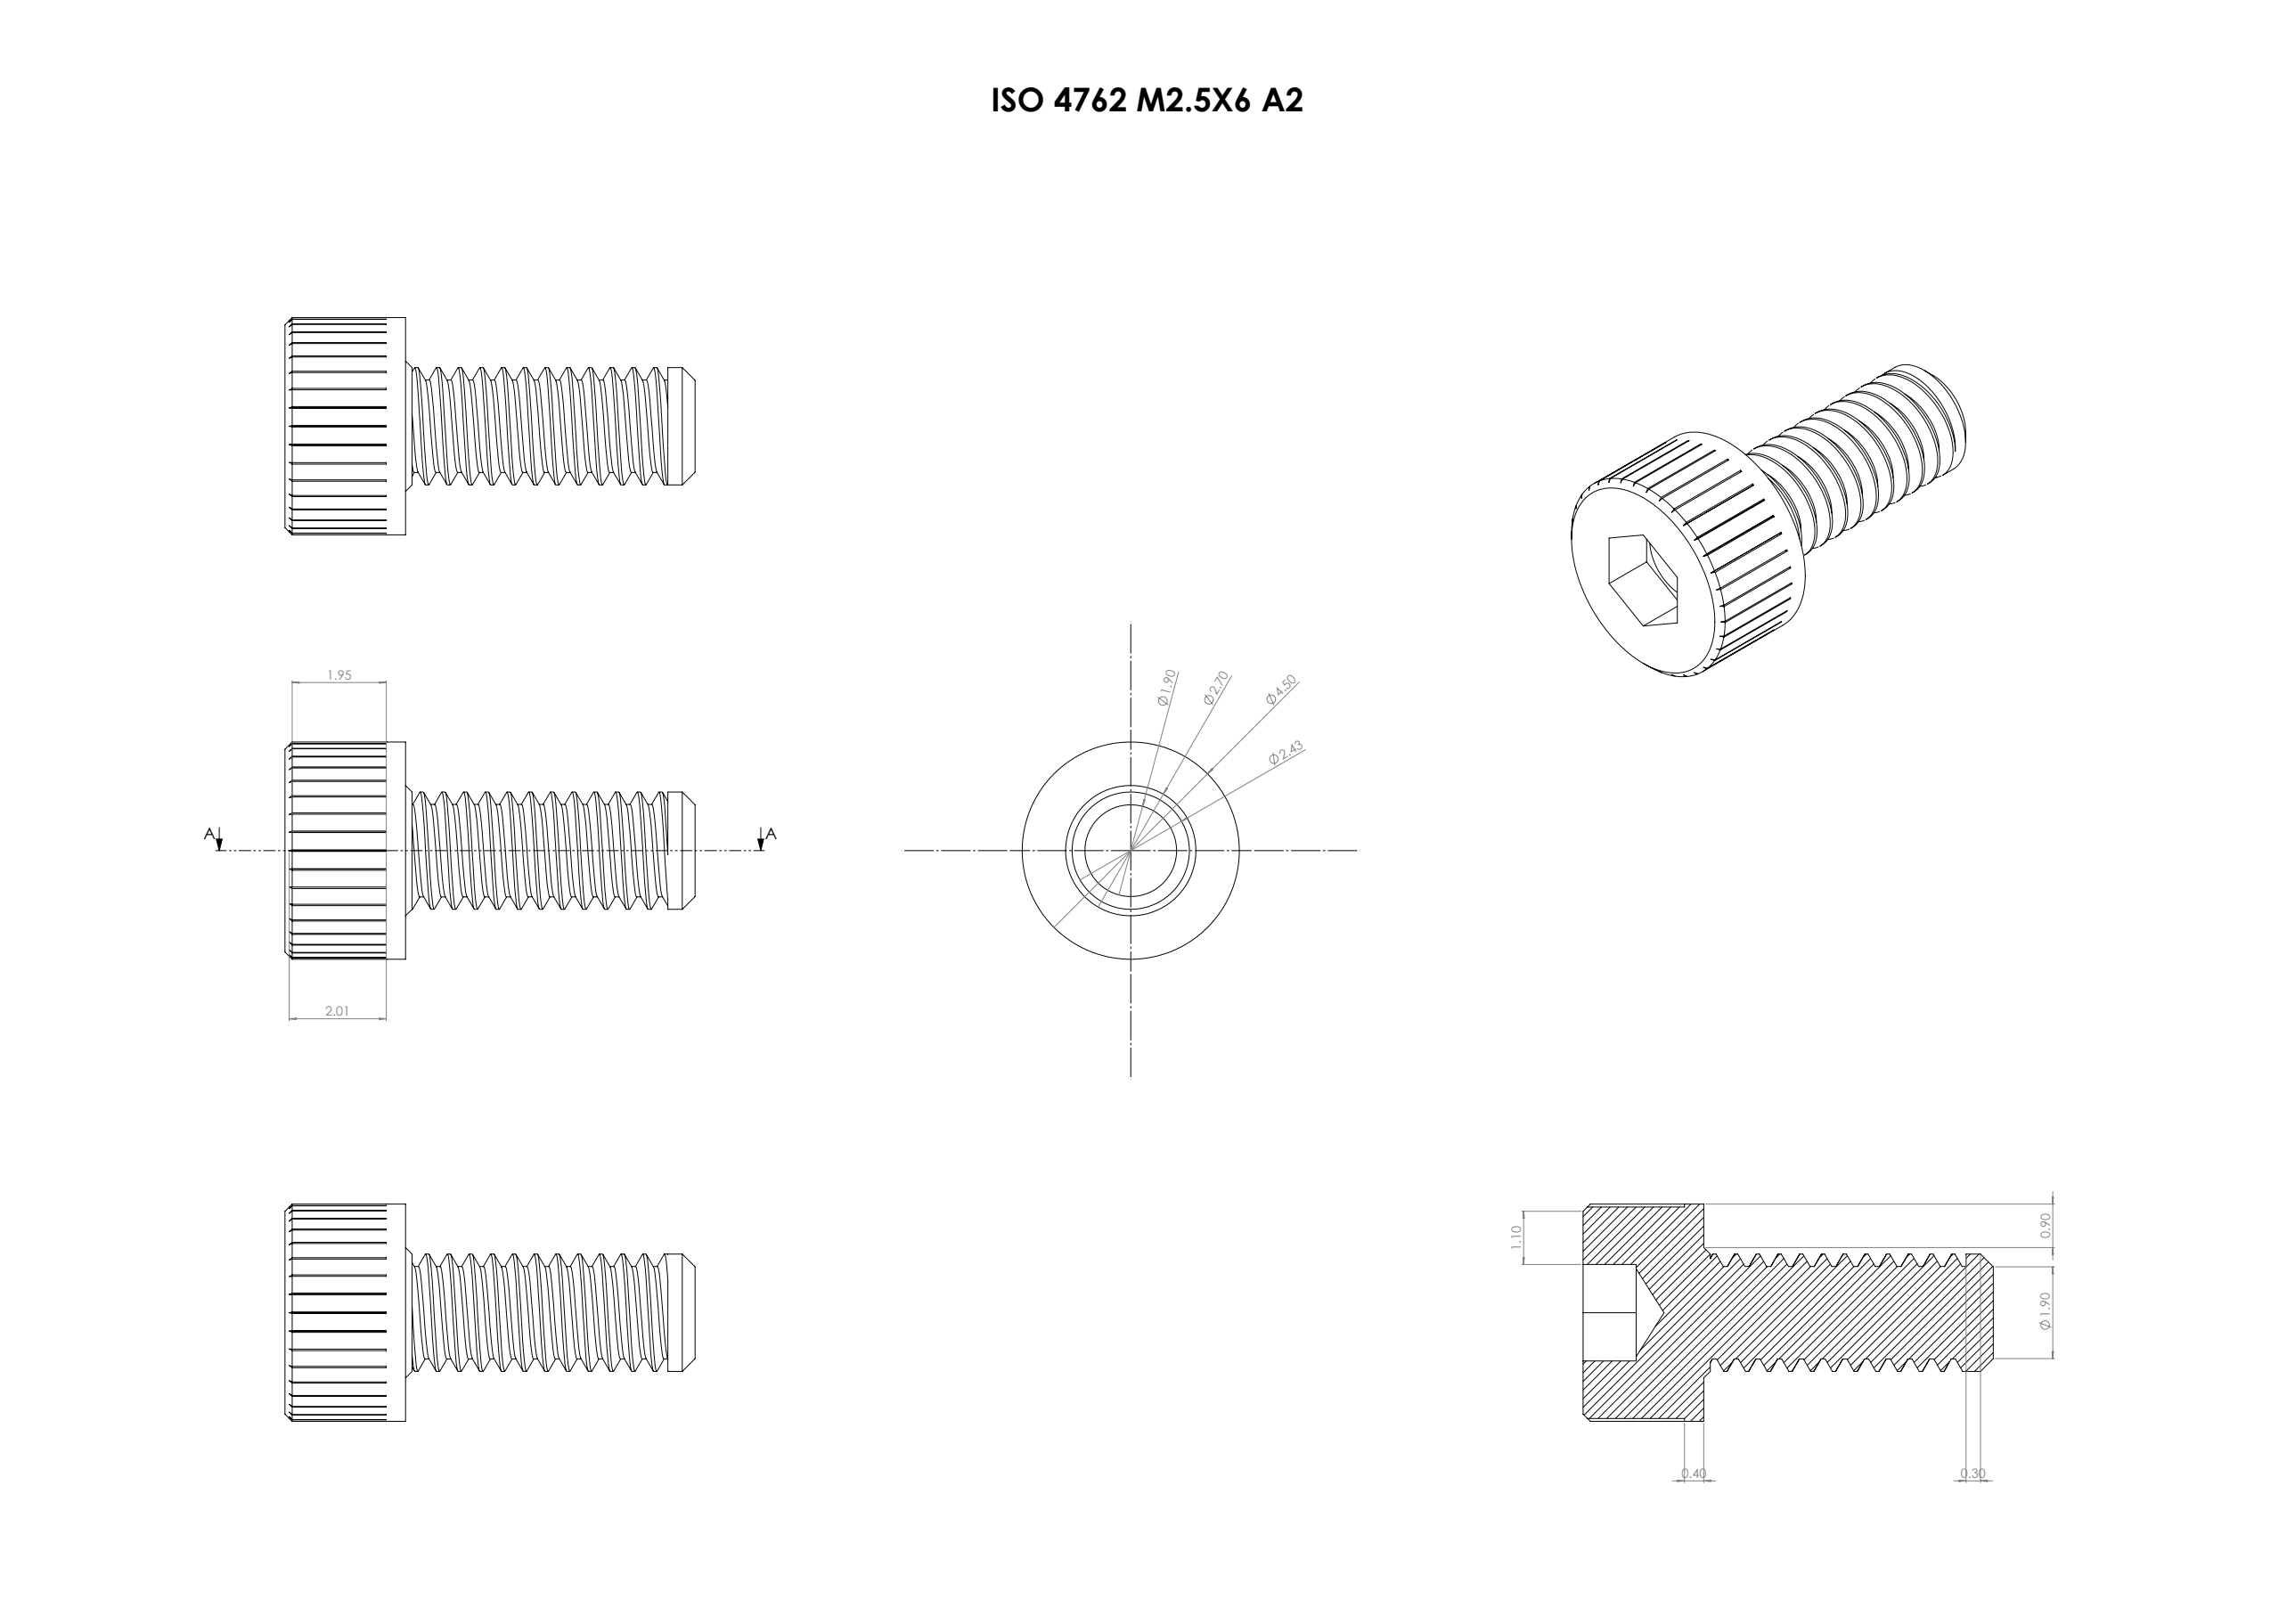
ISO-10303-21;
HEADER;
/* Generated by software containing ST-Developer
 * from STEP Tools, Inc. (www.steptools.com) 
 */

FILE_DESCRIPTION(
/* description */ (''),
/* implementation_level */ '2;1');

FILE_NAME(
/* name */ '17_ISO_4762_M2.5x6_A2.step',
/* time_stamp */ '2026-10-19T23:00:43-07:00',
/* author */ (''),
/* organization */ (''),
/* preprocessor_version */ 'ST-DEVELOPER v20.2',
/* originating_system */ 'Autodesk Translation Framework v15.15.0.0',
/* authorisation */ '');

FILE_SCHEMA (('AUTOMOTIVE_DESIGN { 1 0 10303 214 3 1 1 }'));
ENDSEC;

DATA;
#10=MECHANICAL_DESIGN_GEOMETRIC_PRESENTATION_REPRESENTATION('',(#1013),#55002);
#395=(
BOUNDED_CURVE()
B_SPLINE_CURVE(2,(#50435,#50436,#50437),.UNSPECIFIED.,.F.,.F.)
B_SPLINE_CURVE_WITH_KNOTS((3,3),(0.,0.00844890352465847),.UNSPECIFIED.)
CURVE()
GEOMETRIC_REPRESENTATION_ITEM()
RATIONAL_B_SPLINE_CURVE((1.,1.00024991829741,1.0003043270601))
REPRESENTATION_ITEM('')
);
#396=(
BOUNDED_CURVE()
B_SPLINE_CURVE(2,(#50441,#50442,#50443),.UNSPECIFIED.,.F.,.F.)
B_SPLINE_CURVE_WITH_KNOTS((3,3),(0.0131514300538184,0.0216003335786744),
 .UNSPECIFIED.)
CURVE()
GEOMETRIC_REPRESENTATION_ITEM()
RATIONAL_B_SPLINE_CURVE((1.00030432705462,1.00024991829291,1.))
REPRESENTATION_ITEM('')
);
#397=(
BOUNDED_CURVE()
B_SPLINE_CURVE(2,(#50456,#50457,#50458),.UNSPECIFIED.,.F.,.F.)
B_SPLINE_CURVE_WITH_KNOTS((3,3),(0.,0.00844890352461359),.UNSPECIFIED.)
CURVE()
GEOMETRIC_REPRESENTATION_ITEM()
RATIONAL_B_SPLINE_CURVE((1.,1.00024991829433,1.00030432705636))
REPRESENTATION_ITEM('')
);
#398=(
BOUNDED_CURVE()
B_SPLINE_CURVE(2,(#50462,#50463,#50464),.UNSPECIFIED.,.F.,.F.)
B_SPLINE_CURVE_WITH_KNOTS((3,3),(0.0131514300539352,0.0216003335786744),
 .UNSPECIFIED.)
CURVE()
GEOMETRIC_REPRESENTATION_ITEM()
RATIONAL_B_SPLINE_CURVE((1.0003043270645,1.00024991830102,1.))
REPRESENTATION_ITEM('')
);
#399=(
BOUNDED_CURVE()
B_SPLINE_CURVE(2,(#50477,#50478,#50479),.UNSPECIFIED.,.F.,.F.)
B_SPLINE_CURVE_WITH_KNOTS((3,3),(0.,0.00844890352451554),.UNSPECIFIED.)
CURVE()
GEOMETRIC_REPRESENTATION_ITEM()
RATIONAL_B_SPLINE_CURVE((1.,1.00024991829624,1.00030432705868))
REPRESENTATION_ITEM('')
);
#400=(
BOUNDED_CURVE()
B_SPLINE_CURVE(2,(#50483,#50484,#50485),.UNSPECIFIED.,.F.,.F.)
B_SPLINE_CURVE_WITH_KNOTS((3,3),(0.0131514300537974,0.0216003335786744),
 .UNSPECIFIED.)
CURVE()
GEOMETRIC_REPRESENTATION_ITEM()
RATIONAL_B_SPLINE_CURVE((1.00030432705135,1.00024991829022,1.))
REPRESENTATION_ITEM('')
);
#401=(
BOUNDED_CURVE()
B_SPLINE_CURVE(2,(#50498,#50499,#50500),.UNSPECIFIED.,.F.,.F.)
B_SPLINE_CURVE_WITH_KNOTS((3,3),(0.,0.00844890352473773),.UNSPECIFIED.)
CURVE()
GEOMETRIC_REPRESENTATION_ITEM()
RATIONAL_B_SPLINE_CURVE((1.,1.00024991829766,1.0003043270604))
REPRESENTATION_ITEM('')
);
#402=(
BOUNDED_CURVE()
B_SPLINE_CURVE(2,(#50504,#50505,#50506),.UNSPECIFIED.,.F.,.F.)
B_SPLINE_CURVE_WITH_KNOTS((3,3),(0.0131514300540393,0.0216003335786744),
 .UNSPECIFIED.)
CURVE()
GEOMETRIC_REPRESENTATION_ITEM()
RATIONAL_B_SPLINE_CURVE((1.00030432705889,1.00024991829642,1.))
REPRESENTATION_ITEM('')
);
#403=(
BOUNDED_CURVE()
B_SPLINE_CURVE(2,(#50519,#50520,#50521),.UNSPECIFIED.,.F.,.F.)
B_SPLINE_CURVE_WITH_KNOTS((3,3),(0.,0.00844890352488385),.UNSPECIFIED.)
CURVE()
GEOMETRIC_REPRESENTATION_ITEM()
RATIONAL_B_SPLINE_CURVE((1.,1.00024991830158,1.00030432706517))
REPRESENTATION_ITEM('')
);
#404=(
BOUNDED_CURVE()
B_SPLINE_CURVE(2,(#50525,#50526,#50527),.UNSPECIFIED.,.F.,.F.)
B_SPLINE_CURVE_WITH_KNOTS((3,3),(0.0131514300539214,0.0216003335786743),
 .UNSPECIFIED.)
CURVE()
GEOMETRIC_REPRESENTATION_ITEM()
RATIONAL_B_SPLINE_CURVE((1.00030432705957,1.00024991829698,1.))
REPRESENTATION_ITEM('')
);
#405=(
BOUNDED_CURVE()
B_SPLINE_CURVE(2,(#50540,#50541,#50542),.UNSPECIFIED.,.F.,.F.)
B_SPLINE_CURVE_WITH_KNOTS((3,3),(0.,0.00844890352469842),.UNSPECIFIED.)
CURVE()
GEOMETRIC_REPRESENTATION_ITEM()
RATIONAL_B_SPLINE_CURVE((1.,1.00024991830078,1.00030432706421))
REPRESENTATION_ITEM('')
);
#406=(
BOUNDED_CURVE()
B_SPLINE_CURVE(2,(#50546,#50547,#50548),.UNSPECIFIED.,.F.,.F.)
B_SPLINE_CURVE_WITH_KNOTS((3,3),(0.0131514300540325,0.0216003335786744),
 .UNSPECIFIED.)
CURVE()
GEOMETRIC_REPRESENTATION_ITEM()
RATIONAL_B_SPLINE_CURVE((1.00030432705744,1.00024991829522,1.))
REPRESENTATION_ITEM('')
);
#407=(
BOUNDED_CURVE()
B_SPLINE_CURVE(2,(#50561,#50562,#50563),.UNSPECIFIED.,.F.,.F.)
B_SPLINE_CURVE_WITH_KNOTS((3,3),(0.,0.00844890352489384),.UNSPECIFIED.)
CURVE()
GEOMETRIC_REPRESENTATION_ITEM()
RATIONAL_B_SPLINE_CURVE((1.,1.0002499182915,1.0003043270529))
REPRESENTATION_ITEM('')
);
#408=(
BOUNDED_CURVE()
B_SPLINE_CURVE(2,(#50567,#50568,#50569),.UNSPECIFIED.,.F.,.F.)
B_SPLINE_CURVE_WITH_KNOTS((3,3),(0.0131514300537262,0.0216003335786744),
 .UNSPECIFIED.)
CURVE()
GEOMETRIC_REPRESENTATION_ITEM()
RATIONAL_B_SPLINE_CURVE((1.00030432705672,1.00024991829464,1.))
REPRESENTATION_ITEM('')
);
#409=(
BOUNDED_CURVE()
B_SPLINE_CURVE(2,(#50582,#50583,#50584),.UNSPECIFIED.,.F.,.F.)
B_SPLINE_CURVE_WITH_KNOTS((3,3),(0.,0.00844890352459677),.UNSPECIFIED.)
CURVE()
GEOMETRIC_REPRESENTATION_ITEM()
RATIONAL_B_SPLINE_CURVE((1.,1.00024991829595,1.00030432705833))
REPRESENTATION_ITEM('')
);
#410=(
BOUNDED_CURVE()
B_SPLINE_CURVE(2,(#50588,#50589,#50590),.UNSPECIFIED.,.F.,.F.)
B_SPLINE_CURVE_WITH_KNOTS((3,3),(0.0131514300537522,0.0216003335786743),
 .UNSPECIFIED.)
CURVE()
GEOMETRIC_REPRESENTATION_ITEM()
RATIONAL_B_SPLINE_CURVE((1.00030432705926,1.00024991829673,1.))
REPRESENTATION_ITEM('')
);
#411=(
BOUNDED_CURVE()
B_SPLINE_CURVE(2,(#50603,#50604,#50605),.UNSPECIFIED.,.F.,.F.)
B_SPLINE_CURVE_WITH_KNOTS((3,3),(0.,0.00844890352497871),.UNSPECIFIED.)
CURVE()
GEOMETRIC_REPRESENTATION_ITEM()
RATIONAL_B_SPLINE_CURVE((1.,1.00024991829262,1.00030432705426))
REPRESENTATION_ITEM('')
);
#412=(
BOUNDED_CURVE()
B_SPLINE_CURVE(2,(#50609,#50610,#50611),.UNSPECIFIED.,.F.,.F.)
B_SPLINE_CURVE_WITH_KNOTS((3,3),(0.013151430053846,0.0216003335786743),
 .UNSPECIFIED.)
CURVE()
GEOMETRIC_REPRESENTATION_ITEM()
RATIONAL_B_SPLINE_CURVE((1.00030432705891,1.00024991829644,1.))
REPRESENTATION_ITEM('')
);
#413=(
BOUNDED_CURVE()
B_SPLINE_CURVE(2,(#50624,#50625,#50626),.UNSPECIFIED.,.F.,.F.)
B_SPLINE_CURVE_WITH_KNOTS((3,3),(0.,0.0084489035249234),.UNSPECIFIED.)
CURVE()
GEOMETRIC_REPRESENTATION_ITEM()
RATIONAL_B_SPLINE_CURVE((1.,1.00024991829376,1.00030432705565))
REPRESENTATION_ITEM('')
);
#414=(
BOUNDED_CURVE()
B_SPLINE_CURVE(2,(#50630,#50631,#50632),.UNSPECIFIED.,.F.,.F.)
B_SPLINE_CURVE_WITH_KNOTS((3,3),(0.0131514300540803,0.0216003335786743),
 .UNSPECIFIED.)
CURVE()
GEOMETRIC_REPRESENTATION_ITEM()
RATIONAL_B_SPLINE_CURVE((1.00030432705876,1.00024991829631,1.))
REPRESENTATION_ITEM('')
);
#415=(
BOUNDED_CURVE()
B_SPLINE_CURVE(2,(#50645,#50646,#50647),.UNSPECIFIED.,.F.,.F.)
B_SPLINE_CURVE_WITH_KNOTS((3,3),(0.,0.00844890352494163),.UNSPECIFIED.)
CURVE()
GEOMETRIC_REPRESENTATION_ITEM()
RATIONAL_B_SPLINE_CURVE((1.,1.00024991829715,1.00030432705978))
REPRESENTATION_ITEM('')
);
#416=(
BOUNDED_CURVE()
B_SPLINE_CURVE(2,(#50651,#50652,#50653),.UNSPECIFIED.,.F.,.F.)
B_SPLINE_CURVE_WITH_KNOTS((3,3),(0.0131514300539219,0.0216003335786744),
 .UNSPECIFIED.)
CURVE()
GEOMETRIC_REPRESENTATION_ITEM()
RATIONAL_B_SPLINE_CURVE((1.00030432706217,1.00024991829911,1.))
REPRESENTATION_ITEM('')
);
#417=(
BOUNDED_CURVE()
B_SPLINE_CURVE(2,(#50666,#50667,#50668),.UNSPECIFIED.,.F.,.F.)
B_SPLINE_CURVE_WITH_KNOTS((3,3),(0.,0.00844890352451554),.UNSPECIFIED.)
CURVE()
GEOMETRIC_REPRESENTATION_ITEM()
RATIONAL_B_SPLINE_CURVE((1.,1.00024991829624,1.00030432705868))
REPRESENTATION_ITEM('')
);
#418=(
BOUNDED_CURVE()
B_SPLINE_CURVE(2,(#50672,#50673,#50674),.UNSPECIFIED.,.F.,.F.)
B_SPLINE_CURVE_WITH_KNOTS((3,3),(0.0131514300537974,0.0216003335786744),
 .UNSPECIFIED.)
CURVE()
GEOMETRIC_REPRESENTATION_ITEM()
RATIONAL_B_SPLINE_CURVE((1.00030432705135,1.00024991829022,1.))
REPRESENTATION_ITEM('')
);
#419=(
BOUNDED_CURVE()
B_SPLINE_CURVE(2,(#50687,#50688,#50689),.UNSPECIFIED.,.F.,.F.)
B_SPLINE_CURVE_WITH_KNOTS((3,3),(0.,0.00844890352463462),.UNSPECIFIED.)
CURVE()
GEOMETRIC_REPRESENTATION_ITEM()
RATIONAL_B_SPLINE_CURVE((1.,1.00024991830016,1.00030432706346))
REPRESENTATION_ITEM('')
);
#420=(
BOUNDED_CURVE()
B_SPLINE_CURVE(2,(#50693,#50694,#50695),.UNSPECIFIED.,.F.,.F.)
B_SPLINE_CURVE_WITH_KNOTS((3,3),(0.0131514300541893,0.0216003335786744),
 .UNSPECIFIED.)
CURVE()
GEOMETRIC_REPRESENTATION_ITEM()
RATIONAL_B_SPLINE_CURVE((1.00030432706113,1.00024991829825,1.))
REPRESENTATION_ITEM('')
);
#421=(
BOUNDED_CURVE()
B_SPLINE_CURVE(2,(#50708,#50709,#50710),.UNSPECIFIED.,.F.,.F.)
B_SPLINE_CURVE_WITH_KNOTS((3,3),(0.,0.00844890352460222),.UNSPECIFIED.)
CURVE()
GEOMETRIC_REPRESENTATION_ITEM()
RATIONAL_B_SPLINE_CURVE((1.,1.00024991829658,1.00030432705909))
REPRESENTATION_ITEM('')
);
#422=(
BOUNDED_CURVE()
B_SPLINE_CURVE(2,(#50714,#50715,#50716),.UNSPECIFIED.,.F.,.F.)
B_SPLINE_CURVE_WITH_KNOTS((3,3),(0.0131514300537623,0.0216003335786744),
 .UNSPECIFIED.)
CURVE()
GEOMETRIC_REPRESENTATION_ITEM()
RATIONAL_B_SPLINE_CURVE((1.00030432705572,1.00024991829381,1.))
REPRESENTATION_ITEM('')
);
#423=(
BOUNDED_CURVE()
B_SPLINE_CURVE(2,(#50729,#50730,#50731),.UNSPECIFIED.,.F.,.F.)
B_SPLINE_CURVE_WITH_KNOTS((3,3),(0.,0.00844890352469488),.UNSPECIFIED.)
CURVE()
GEOMETRIC_REPRESENTATION_ITEM()
RATIONAL_B_SPLINE_CURVE((1.,1.00024991830183,1.00030432706549))
REPRESENTATION_ITEM('')
);
#424=(
BOUNDED_CURVE()
B_SPLINE_CURVE(2,(#50735,#50736,#50737),.UNSPECIFIED.,.F.,.F.)
B_SPLINE_CURVE_WITH_KNOTS((3,3),(0.0131514300540722,0.0216003335786744),
 .UNSPECIFIED.)
CURVE()
GEOMETRIC_REPRESENTATION_ITEM()
RATIONAL_B_SPLINE_CURVE((1.00030432706317,1.00024991829993,1.))
REPRESENTATION_ITEM('')
);
#425=(
BOUNDED_CURVE()
B_SPLINE_CURVE(2,(#50750,#50751,#50752),.UNSPECIFIED.,.F.,.F.)
B_SPLINE_CURVE_WITH_KNOTS((3,3),(0.,0.00844890352449406),.UNSPECIFIED.)
CURVE()
GEOMETRIC_REPRESENTATION_ITEM()
RATIONAL_B_SPLINE_CURVE((1.,1.00024991829771,1.00030432706047))
REPRESENTATION_ITEM('')
);
#426=(
BOUNDED_CURVE()
B_SPLINE_CURVE(2,(#50756,#50757,#50758),.UNSPECIFIED.,.F.,.F.)
B_SPLINE_CURVE_WITH_KNOTS((3,3),(0.0131514300538891,0.0216003335786743),
 .UNSPECIFIED.)
CURVE()
GEOMETRIC_REPRESENTATION_ITEM()
RATIONAL_B_SPLINE_CURVE((1.00030432705489,1.00024991829313,1.))
REPRESENTATION_ITEM('')
);
#427=(
BOUNDED_CURVE()
B_SPLINE_CURVE(2,(#50771,#50772,#50773),.UNSPECIFIED.,.F.,.F.)
B_SPLINE_CURVE_WITH_KNOTS((3,3),(0.,0.0084489035245959),.UNSPECIFIED.)
CURVE()
GEOMETRIC_REPRESENTATION_ITEM()
RATIONAL_B_SPLINE_CURVE((1.,1.00024991829567,1.00030432705798))
REPRESENTATION_ITEM('')
);
#428=(
BOUNDED_CURVE()
B_SPLINE_CURVE(2,(#50777,#50778,#50779),.UNSPECIFIED.,.F.,.F.)
B_SPLINE_CURVE_WITH_KNOTS((3,3),(0.0131514300537466,0.0216003335786743),
 .UNSPECIFIED.)
CURVE()
GEOMETRIC_REPRESENTATION_ITEM()
RATIONAL_B_SPLINE_CURVE((1.00030432705734,1.00024991829515,1.))
REPRESENTATION_ITEM('')
);
#429=(
BOUNDED_CURVE()
B_SPLINE_CURVE(2,(#50794,#50795,#50796),.UNSPECIFIED.,.F.,.F.)
B_SPLINE_CURVE_WITH_KNOTS((3,3),(0.,0.00844890352496291),.UNSPECIFIED.)
CURVE()
GEOMETRIC_REPRESENTATION_ITEM()
RATIONAL_B_SPLINE_CURVE((1.,1.00024991829663,1.00030432705914))
REPRESENTATION_ITEM('')
);
#430=(
BOUNDED_CURVE()
B_SPLINE_CURVE(2,(#50800,#50801,#50802),.UNSPECIFIED.,.F.,.F.)
B_SPLINE_CURVE_WITH_KNOTS((3,3),(0.0131514300540908,0.0216003335786744),
 .UNSPECIFIED.)
CURVE()
GEOMETRIC_REPRESENTATION_ITEM()
RATIONAL_B_SPLINE_CURVE((1.00030432705721,1.00024991829503,1.))
REPRESENTATION_ITEM('')
);
#431=(
BOUNDED_CURVE()
B_SPLINE_CURVE(2,(#50815,#50816,#50817),.UNSPECIFIED.,.F.,.F.)
B_SPLINE_CURVE_WITH_KNOTS((3,3),(0.,0.00844890352464343),.UNSPECIFIED.)
CURVE()
GEOMETRIC_REPRESENTATION_ITEM()
RATIONAL_B_SPLINE_CURVE((1.,1.00024991829906,1.00030432706212))
REPRESENTATION_ITEM('')
);
#432=(
BOUNDED_CURVE()
B_SPLINE_CURVE(2,(#50821,#50822,#50823),.UNSPECIFIED.,.F.,.F.)
B_SPLINE_CURVE_WITH_KNOTS((3,3),(0.0131514300538374,0.0216003335786744),
 .UNSPECIFIED.)
CURVE()
GEOMETRIC_REPRESENTATION_ITEM()
RATIONAL_B_SPLINE_CURVE((1.00030432706069,1.0002499182979,1.))
REPRESENTATION_ITEM('')
);
#433=(
BOUNDED_CURVE()
B_SPLINE_CURVE(2,(#50836,#50837,#50838),.UNSPECIFIED.,.F.,.F.)
B_SPLINE_CURVE_WITH_KNOTS((3,3),(0.,0.00844890352478188),.UNSPECIFIED.)
CURVE()
GEOMETRIC_REPRESENTATION_ITEM()
RATIONAL_B_SPLINE_CURVE((1.,1.00024991829664,1.00030432705917))
REPRESENTATION_ITEM('')
);
#434=(
BOUNDED_CURVE()
B_SPLINE_CURVE(2,(#50842,#50843,#50844),.UNSPECIFIED.,.F.,.F.)
B_SPLINE_CURVE_WITH_KNOTS((3,3),(0.0131514300539186,0.0216003335786744),
 .UNSPECIFIED.)
CURVE()
GEOMETRIC_REPRESENTATION_ITEM()
RATIONAL_B_SPLINE_CURVE((1.00030432706174,1.00024991829875,1.))
REPRESENTATION_ITEM('')
);
#435=(
BOUNDED_CURVE()
B_SPLINE_CURVE(2,(#50857,#50858,#50859),.UNSPECIFIED.,.F.,.F.)
B_SPLINE_CURVE_WITH_KNOTS((3,3),(0.,0.00844890352473528),.UNSPECIFIED.)
CURVE()
GEOMETRIC_REPRESENTATION_ITEM()
RATIONAL_B_SPLINE_CURVE((1.,1.00024991829715,1.00030432705979))
REPRESENTATION_ITEM('')
);
#436=(
BOUNDED_CURVE()
B_SPLINE_CURVE(2,(#50863,#50864,#50865),.UNSPECIFIED.,.F.,.F.)
B_SPLINE_CURVE_WITH_KNOTS((3,3),(0.0131514300540877,0.0216003335786744),
 .UNSPECIFIED.)
CURVE()
GEOMETRIC_REPRESENTATION_ITEM()
RATIONAL_B_SPLINE_CURVE((1.00030432705704,1.0002499182949,1.))
REPRESENTATION_ITEM('')
);
#437=(
BOUNDED_CURVE()
B_SPLINE_CURVE(2,(#50878,#50879,#50880),.UNSPECIFIED.,.F.,.F.)
B_SPLINE_CURVE_WITH_KNOTS((3,3),(0.,0.00844890352463462),.UNSPECIFIED.)
CURVE()
GEOMETRIC_REPRESENTATION_ITEM()
RATIONAL_B_SPLINE_CURVE((1.,1.00024991830016,1.00030432706346))
REPRESENTATION_ITEM('')
);
#438=(
BOUNDED_CURVE()
B_SPLINE_CURVE(2,(#50884,#50885,#50886),.UNSPECIFIED.,.F.,.F.)
B_SPLINE_CURVE_WITH_KNOTS((3,3),(0.0131514300541893,0.0216003335786744),
 .UNSPECIFIED.)
CURVE()
GEOMETRIC_REPRESENTATION_ITEM()
RATIONAL_B_SPLINE_CURVE((1.00030432706113,1.00024991829825,1.))
REPRESENTATION_ITEM('')
);
#439=(
BOUNDED_CURVE()
B_SPLINE_CURVE(2,(#50899,#50900,#50901),.UNSPECIFIED.,.F.,.F.)
B_SPLINE_CURVE_WITH_KNOTS((3,3),(0.,0.00844890352448517),.UNSPECIFIED.)
CURVE()
GEOMETRIC_REPRESENTATION_ITEM()
RATIONAL_B_SPLINE_CURVE((1.,1.00024991829772,1.00030432706048))
REPRESENTATION_ITEM('')
);
#440=(
BOUNDED_CURVE()
B_SPLINE_CURVE(2,(#50905,#50906,#50907),.UNSPECIFIED.,.F.,.F.)
B_SPLINE_CURVE_WITH_KNOTS((3,3),(0.0131514300541692,0.0216003335786743),
 .UNSPECIFIED.)
CURVE()
GEOMETRIC_REPRESENTATION_ITEM()
RATIONAL_B_SPLINE_CURVE((1.00030432705767,1.00024991829541,1.))
REPRESENTATION_ITEM('')
);
#441=(
BOUNDED_CURVE()
B_SPLINE_CURVE(2,(#50920,#50921,#50922),.UNSPECIFIED.,.F.,.F.)
B_SPLINE_CURVE_WITH_KNOTS((3,3),(0.,0.00844890352459986),.UNSPECIFIED.)
CURVE()
GEOMETRIC_REPRESENTATION_ITEM()
RATIONAL_B_SPLINE_CURVE((1.,1.00024991829621,1.00030432705864))
REPRESENTATION_ITEM('')
);
#442=(
BOUNDED_CURVE()
B_SPLINE_CURVE(2,(#50926,#50927,#50928),.UNSPECIFIED.,.F.,.F.)
B_SPLINE_CURVE_WITH_KNOTS((3,3),(0.0131514300539527,0.0216003335786744),
 .UNSPECIFIED.)
CURVE()
GEOMETRIC_REPRESENTATION_ITEM()
RATIONAL_B_SPLINE_CURVE((1.0003043270617,1.00024991829873,1.))
REPRESENTATION_ITEM('')
);
#443=(
BOUNDED_CURVE()
B_SPLINE_CURVE(2,(#50941,#50942,#50943),.UNSPECIFIED.,.F.,.F.)
B_SPLINE_CURVE_WITH_KNOTS((3,3),(0.,0.00844890352449406),.UNSPECIFIED.)
CURVE()
GEOMETRIC_REPRESENTATION_ITEM()
RATIONAL_B_SPLINE_CURVE((1.,1.00024991829771,1.00030432706047))
REPRESENTATION_ITEM('')
);
#444=(
BOUNDED_CURVE()
B_SPLINE_CURVE(2,(#50947,#50948,#50949),.UNSPECIFIED.,.F.,.F.)
B_SPLINE_CURVE_WITH_KNOTS((3,3),(0.0131514300538891,0.0216003335786743),
 .UNSPECIFIED.)
CURVE()
GEOMETRIC_REPRESENTATION_ITEM()
RATIONAL_B_SPLINE_CURVE((1.00030432705489,1.00024991829313,1.))
REPRESENTATION_ITEM('')
);
#445=(
BOUNDED_CURVE()
B_SPLINE_CURVE(2,(#50962,#50963,#50964),.UNSPECIFIED.,.F.,.F.)
B_SPLINE_CURVE_WITH_KNOTS((3,3),(0.,0.00844890352485641),.UNSPECIFIED.)
CURVE()
GEOMETRIC_REPRESENTATION_ITEM()
RATIONAL_B_SPLINE_CURVE((1.,1.00024991829199,1.0003043270535))
REPRESENTATION_ITEM('')
);
#446=(
BOUNDED_CURVE()
B_SPLINE_CURVE(2,(#50968,#50969,#50970),.UNSPECIFIED.,.F.,.F.)
B_SPLINE_CURVE_WITH_KNOTS((3,3),(0.0131514300537428,0.0216003335786744),
 .UNSPECIFIED.)
CURVE()
GEOMETRIC_REPRESENTATION_ITEM()
RATIONAL_B_SPLINE_CURVE((1.00030432705361,1.00024991829208,1.))
REPRESENTATION_ITEM('')
);
#447=(
BOUNDED_CURVE()
B_SPLINE_CURVE(2,(#50983,#50984,#50985),.UNSPECIFIED.,.F.,.F.)
B_SPLINE_CURVE_WITH_KNOTS((3,3),(0.,0.00844890352496226),.UNSPECIFIED.)
CURVE()
GEOMETRIC_REPRESENTATION_ITEM()
RATIONAL_B_SPLINE_CURVE((1.,1.00024991829658,1.00030432705909))
REPRESENTATION_ITEM('')
);
#448=(
BOUNDED_CURVE()
B_SPLINE_CURVE(2,(#50989,#50990,#50991),.UNSPECIFIED.,.F.,.F.)
B_SPLINE_CURVE_WITH_KNOTS((3,3),(0.013151430054111,0.0216003335786744),
 .UNSPECIFIED.)
CURVE()
GEOMETRIC_REPRESENTATION_ITEM()
RATIONAL_B_SPLINE_CURVE((1.00030432706545,1.0002499183018,1.))
REPRESENTATION_ITEM('')
);
#449=(
BOUNDED_CURVE()
B_SPLINE_CURVE(2,(#51004,#51005,#51006),.UNSPECIFIED.,.F.,.F.)
B_SPLINE_CURVE_WITH_KNOTS((3,3),(0.,0.00844890352465218),.UNSPECIFIED.)
CURVE()
GEOMETRIC_REPRESENTATION_ITEM()
RATIONAL_B_SPLINE_CURVE((1.,1.0002499182964,1.00030432705887))
REPRESENTATION_ITEM('')
);
#450=(
BOUNDED_CURVE()
B_SPLINE_CURVE(2,(#51010,#51011,#51012),.UNSPECIFIED.,.F.,.F.)
B_SPLINE_CURVE_WITH_KNOTS((3,3),(0.0131514300538194,0.0216003335786744),
 .UNSPECIFIED.)
CURVE()
GEOMETRIC_REPRESENTATION_ITEM()
RATIONAL_B_SPLINE_CURVE((1.00030432705442,1.00024991829275,1.))
REPRESENTATION_ITEM('')
);
#451=(
BOUNDED_CURVE()
B_SPLINE_CURVE(2,(#51025,#51026,#51027),.UNSPECIFIED.,.F.,.F.)
B_SPLINE_CURVE_WITH_KNOTS((3,3),(0.,0.00844890352478188),.UNSPECIFIED.)
CURVE()
GEOMETRIC_REPRESENTATION_ITEM()
RATIONAL_B_SPLINE_CURVE((1.,1.00024991829664,1.00030432705917))
REPRESENTATION_ITEM('')
);
#452=(
BOUNDED_CURVE()
B_SPLINE_CURVE(2,(#51031,#51032,#51033),.UNSPECIFIED.,.F.,.F.)
B_SPLINE_CURVE_WITH_KNOTS((3,3),(0.0131514300539186,0.0216003335786744),
 .UNSPECIFIED.)
CURVE()
GEOMETRIC_REPRESENTATION_ITEM()
RATIONAL_B_SPLINE_CURVE((1.00030432706174,1.00024991829875,1.))
REPRESENTATION_ITEM('')
);
#453=(
BOUNDED_CURVE()
B_SPLINE_CURVE(2,(#51046,#51047,#51048),.UNSPECIFIED.,.F.,.F.)
B_SPLINE_CURVE_WITH_KNOTS((3,3),(0.,0.00844890352442994),.UNSPECIFIED.)
CURVE()
GEOMETRIC_REPRESENTATION_ITEM()
RATIONAL_B_SPLINE_CURVE((1.,1.00024991829785,1.00030432706064))
REPRESENTATION_ITEM('')
);
#454=(
BOUNDED_CURVE()
B_SPLINE_CURVE(2,(#51052,#51053,#51054),.UNSPECIFIED.,.F.,.F.)
B_SPLINE_CURVE_WITH_KNOTS((3,3),(0.0131514300540965,0.0216003335786744),
 .UNSPECIFIED.)
CURVE()
GEOMETRIC_REPRESENTATION_ITEM()
RATIONAL_B_SPLINE_CURVE((1.00030432706039,1.00024991829765,1.))
REPRESENTATION_ITEM('')
);
#455=(
BOUNDED_CURVE()
B_SPLINE_CURVE(2,(#51067,#51068,#51069),.UNSPECIFIED.,.F.,.F.)
B_SPLINE_CURVE_WITH_KNOTS((3,3),(0.,0.00844890352481575),.UNSPECIFIED.)
CURVE()
GEOMETRIC_REPRESENTATION_ITEM()
RATIONAL_B_SPLINE_CURVE((1.,1.00024991829544,1.00030432705769))
REPRESENTATION_ITEM('')
);
#456=(
BOUNDED_CURVE()
B_SPLINE_CURVE(2,(#51073,#51074,#51075),.UNSPECIFIED.,.F.,.F.)
B_SPLINE_CURVE_WITH_KNOTS((3,3),(0.0131514300539347,0.0216003335786744),
 .UNSPECIFIED.)
CURVE()
GEOMETRIC_REPRESENTATION_ITEM()
RATIONAL_B_SPLINE_CURVE((1.0003043270581,1.00024991829577,1.))
REPRESENTATION_ITEM('')
);
#457=(
BOUNDED_CURVE()
B_SPLINE_CURVE(2,(#51088,#51089,#51090),.UNSPECIFIED.,.F.,.F.)
B_SPLINE_CURVE_WITH_KNOTS((3,3),(0.,0.00844890352460222),.UNSPECIFIED.)
CURVE()
GEOMETRIC_REPRESENTATION_ITEM()
RATIONAL_B_SPLINE_CURVE((1.,1.00024991829658,1.00030432705909))
REPRESENTATION_ITEM('')
);
#458=(
BOUNDED_CURVE()
B_SPLINE_CURVE(2,(#51094,#51095,#51096),.UNSPECIFIED.,.F.,.F.)
B_SPLINE_CURVE_WITH_KNOTS((3,3),(0.0131514300537623,0.0216003335786744),
 .UNSPECIFIED.)
CURVE()
GEOMETRIC_REPRESENTATION_ITEM()
RATIONAL_B_SPLINE_CURVE((1.00030432705572,1.00024991829381,1.))
REPRESENTATION_ITEM('')
);
#459=(
BOUNDED_CURVE()
B_SPLINE_CURVE(2,(#51109,#51110,#51111),.UNSPECIFIED.,.F.,.F.)
B_SPLINE_CURVE_WITH_KNOTS((3,3),(0.,0.00844890352458545),.UNSPECIFIED.)
CURVE()
GEOMETRIC_REPRESENTATION_ITEM()
RATIONAL_B_SPLINE_CURVE((1.,1.00024991829762,1.00030432706036))
REPRESENTATION_ITEM('')
);
#460=(
BOUNDED_CURVE()
B_SPLINE_CURVE(2,(#51115,#51116,#51117),.UNSPECIFIED.,.F.,.F.)
B_SPLINE_CURVE_WITH_KNOTS((3,3),(0.0131514300540622,0.0216003335786744),
 .UNSPECIFIED.)
CURVE()
GEOMETRIC_REPRESENTATION_ITEM()
RATIONAL_B_SPLINE_CURVE((1.0003043270597,1.00024991829708,1.))
REPRESENTATION_ITEM('')
);
#461=(
BOUNDED_CURVE()
B_SPLINE_CURVE(2,(#51130,#51131,#51132),.UNSPECIFIED.,.F.,.F.)
B_SPLINE_CURVE_WITH_KNOTS((3,3),(0.,0.00844890352449406),.UNSPECIFIED.)
CURVE()
GEOMETRIC_REPRESENTATION_ITEM()
RATIONAL_B_SPLINE_CURVE((1.,1.00024991829771,1.00030432706047))
REPRESENTATION_ITEM('')
);
#462=(
BOUNDED_CURVE()
B_SPLINE_CURVE(2,(#51136,#51137,#51138),.UNSPECIFIED.,.F.,.F.)
B_SPLINE_CURVE_WITH_KNOTS((3,3),(0.0131514300538891,0.0216003335786743),
 .UNSPECIFIED.)
CURVE()
GEOMETRIC_REPRESENTATION_ITEM()
RATIONAL_B_SPLINE_CURVE((1.00030432705489,1.00024991829313,1.))
REPRESENTATION_ITEM('')
);
#463=(
BOUNDED_CURVE()
B_SPLINE_CURVE(2,(#51151,#51152,#51153),.UNSPECIFIED.,.F.,.F.)
B_SPLINE_CURVE_WITH_KNOTS((3,3),(0.,0.00844890352472574),.UNSPECIFIED.)
CURVE()
GEOMETRIC_REPRESENTATION_ITEM()
RATIONAL_B_SPLINE_CURVE((1.,1.00024991829962,1.00030432706279))
REPRESENTATION_ITEM('')
);
#464=(
BOUNDED_CURVE()
B_SPLINE_CURVE(2,(#51157,#51158,#51159),.UNSPECIFIED.,.F.,.F.)
B_SPLINE_CURVE_WITH_KNOTS((3,3),(0.0131514300538617,0.0216003335786744),
 .UNSPECIFIED.)
CURVE()
GEOMETRIC_REPRESENTATION_ITEM()
RATIONAL_B_SPLINE_CURVE((1.00030432705112,1.00024991829003,1.))
REPRESENTATION_ITEM('')
);
#465=(
BOUNDED_CURVE()
B_SPLINE_CURVE(2,(#51212,#51213,#51214),.UNSPECIFIED.,.F.,.F.)
B_SPLINE_CURVE_WITH_KNOTS((3,3),(0.,0.00844890352456175),.UNSPECIFIED.)
CURVE()
GEOMETRIC_REPRESENTATION_ITEM()
RATIONAL_B_SPLINE_CURVE((1.,1.00024991829887,1.00030432706188))
REPRESENTATION_ITEM('')
);
#466=(
BOUNDED_CURVE()
B_SPLINE_CURVE(2,(#51216,#51217,#51218),.UNSPECIFIED.,.F.,.F.)
B_SPLINE_CURVE_WITH_KNOTS((3,3),(0.0131514300541029,0.0216003335786743),
 .UNSPECIFIED.)
CURVE()
GEOMETRIC_REPRESENTATION_ITEM()
RATIONAL_B_SPLINE_CURVE((1.00030432705952,1.00024991829693,1.))
REPRESENTATION_ITEM('')
);
#478=B_SPLINE_SURFACE_WITH_KNOTS('',3,3,((#49663,#49664,#49665,#49666,#49667,
#49668,#49669,#49670,#49671,#49672,#49673,#49674,#49675,#49676,#49677,#49678,
#49679,#49680,#49681,#49682,#49683,#49684,#49685,#49686,#49687,#49688,#49689,
#49690,#49691,#49692,#49693,#49694,#49695,#49696,#49697,#49698,#49699,#49700,
#49701,#49702,#49703,#49704,#49705,#49706,#49707,#49708,#49709,#49710,#49711,
#49712,#49713,#49714,#49715,#49716,#49717,#49718,#49719,#49720,#49721,#49722,
#49723,#49724,#49725,#49726,#49727,#49728,#49729,#49730,#49731,#49732,#49733,
#49734,#49735,#49736,#49737,#49738,#49739,#49740,#49741,#49742),(#49743,
#49744,#49745,#49746,#49747,#49748,#49749,#49750,#49751,#49752,#49753,#49754,
#49755,#49756,#49757,#49758,#49759,#49760,#49761,#49762,#49763,#49764,#49765,
#49766,#49767,#49768,#49769,#49770,#49771,#49772,#49773,#49774,#49775,#49776,
#49777,#49778,#49779,#49780,#49781,#49782,#49783,#49784,#49785,#49786,#49787,
#49788,#49789,#49790,#49791,#49792,#49793,#49794,#49795,#49796,#49797,#49798,
#49799,#49800,#49801,#49802,#49803,#49804,#49805,#49806,#49807,#49808,#49809,
#49810,#49811,#49812,#49813,#49814,#49815,#49816,#49817,#49818,#49819,#49820,
#49821,#49822),(#49823,#49824,#49825,#49826,#49827,#49828,#49829,#49830,
#49831,#49832,#49833,#49834,#49835,#49836,#49837,#49838,#49839,#49840,#49841,
#49842,#49843,#49844,#49845,#49846,#49847,#49848,#49849,#49850,#49851,#49852,
#49853,#49854,#49855,#49856,#49857,#49858,#49859,#49860,#49861,#49862,#49863,
#49864,#49865,#49866,#49867,#49868,#49869,#49870,#49871,#49872,#49873,#49874,
#49875,#49876,#49877,#49878,#49879,#49880,#49881,#49882,#49883,#49884,#49885,
#49886,#49887,#49888,#49889,#49890,#49891,#49892,#49893,#49894,#49895,#49896,
#49897,#49898,#49899,#49900,#49901,#49902),(#49903,#49904,#49905,#49906,
#49907,#49908,#49909,#49910,#49911,#49912,#49913,#49914,#49915,#49916,#49917,
#49918,#49919,#49920,#49921,#49922,#49923,#49924,#49925,#49926,#49927,#49928,
#49929,#49930,#49931,#49932,#49933,#49934,#49935,#49936,#49937,#49938,#49939,
#49940,#49941,#49942,#49943,#49944,#49945,#49946,#49947,#49948,#49949,#49950,
#49951,#49952,#49953,#49954,#49955,#49956,#49957,#49958,#49959,#49960,#49961,
#49962,#49963,#49964,#49965,#49966,#49967,#49968,#49969,#49970,#49971,#49972,
#49973,#49974,#49975,#49976,#49977,#49978,#49979,#49980,#49981,#49982)),
 .UNSPECIFIED.,.F.,.F.,.F.,(4,4),(4,1,1,1,1,1,1,1,1,1,1,1,1,1,1,1,1,1,1,
1,1,1,1,1,1,1,1,1,1,1,1,1,1,1,1,1,1,1,1,1,1,1,1,1,1,1,1,1,1,1,1,1,1,1,1,
1,1,1,1,1,1,1,1,1,1,1,1,1,1,1,1,1,1,1,1,1,1,4),(0.,0.0296469363228873),
(12.4950585576113,13.4830028029673,14.4709470483233,15.4588912936793,16.4468355390354,
17.4347797843914,18.4227240297474,19.4106682751034,20.3986125204594,21.3865567658155,
22.3745010111715,23.3624452565275,24.3503895018835,25.3383337472395,26.3262779925956,
27.3142222379516,28.3021664833076,29.2901107286636,30.2780549740196,31.2659992193757,
32.2539434647317,33.2418877100877,34.2298319554437,35.2177762007997,36.2057204461558,
37.1936646915118,38.1816089368678,39.1695531822238,40.1574974275798,41.1454416729359,
42.1333859182919,43.1213301636479,44.1092744090039,45.0972186543599,46.085162899716,
47.073107145072,48.061051390428,49.048995635784,50.03693988114,51.0248841264961,
52.0128283718521,53.0007726172081,53.9887168625641,54.9766611079201,55.9646053532762,
56.9525495986322,57.9404938439882,58.9284380893442,59.9163823347002,60.9043265800563,
61.8922708254123,62.8802150707683,63.8681593161243,64.8561035614803,65.8440478068363,
66.8319920521924,67.8199362975484,68.8078805429044,69.7958247882604,70.7837690336165,
71.7717132789725,72.7596575243285,73.7476017696845,74.7355460150405,75.7234902603965,
76.7114345057526,77.6993787511086,78.6873229964646,79.6752672418206,80.6632114871766,
81.6511557325327,82.6390999778887,83.6270442232447,84.6149884686007,85.6029327139567,
86.5908769593128,87.5788212046688,88.5667654500248),.UNSPECIFIED.);
#479=B_SPLINE_SURFACE_WITH_KNOTS('',3,3,((#50097,#50098,#50099,#50100,#50101,
#50102,#50103,#50104,#50105,#50106,#50107,#50108,#50109,#50110,#50111,#50112,
#50113,#50114,#50115,#50116,#50117,#50118,#50119,#50120,#50121,#50122,#50123,
#50124,#50125,#50126,#50127,#50128,#50129,#50130,#50131,#50132,#50133,#50134,
#50135,#50136,#50137,#50138,#50139,#50140,#50141,#50142,#50143,#50144,#50145,
#50146,#50147,#50148,#50149,#50150,#50151,#50152,#50153,#50154,#50155,#50156,
#50157,#50158,#50159,#50160,#50161,#50162,#50163,#50164,#50165,#50166,#50167,
#50168,#50169,#50170,#50171,#50172,#50173,#50174,#50175,#50176),(#50177,
#50178,#50179,#50180,#50181,#50182,#50183,#50184,#50185,#50186,#50187,#50188,
#50189,#50190,#50191,#50192,#50193,#50194,#50195,#50196,#50197,#50198,#50199,
#50200,#50201,#50202,#50203,#50204,#50205,#50206,#50207,#50208,#50209,#50210,
#50211,#50212,#50213,#50214,#50215,#50216,#50217,#50218,#50219,#50220,#50221,
#50222,#50223,#50224,#50225,#50226,#50227,#50228,#50229,#50230,#50231,#50232,
#50233,#50234,#50235,#50236,#50237,#50238,#50239,#50240,#50241,#50242,#50243,
#50244,#50245,#50246,#50247,#50248,#50249,#50250,#50251,#50252,#50253,#50254,
#50255,#50256),(#50257,#50258,#50259,#50260,#50261,#50262,#50263,#50264,
#50265,#50266,#50267,#50268,#50269,#50270,#50271,#50272,#50273,#50274,#50275,
#50276,#50277,#50278,#50279,#50280,#50281,#50282,#50283,#50284,#50285,#50286,
#50287,#50288,#50289,#50290,#50291,#50292,#50293,#50294,#50295,#50296,#50297,
#50298,#50299,#50300,#50301,#50302,#50303,#50304,#50305,#50306,#50307,#50308,
#50309,#50310,#50311,#50312,#50313,#50314,#50315,#50316,#50317,#50318,#50319,
#50320,#50321,#50322,#50323,#50324,#50325,#50326,#50327,#50328,#50329,#50330,
#50331,#50332,#50333,#50334,#50335,#50336),(#50337,#50338,#50339,#50340,
#50341,#50342,#50343,#50344,#50345,#50346,#50347,#50348,#50349,#50350,#50351,
#50352,#50353,#50354,#50355,#50356,#50357,#50358,#50359,#50360,#50361,#50362,
#50363,#50364,#50365,#50366,#50367,#50368,#50369,#50370,#50371,#50372,#50373,
#50374,#50375,#50376,#50377,#50378,#50379,#50380,#50381,#50382,#50383,#50384,
#50385,#50386,#50387,#50388,#50389,#50390,#50391,#50392,#50393,#50394,#50395,
#50396,#50397,#50398,#50399,#50400,#50401,#50402,#50403,#50404,#50405,#50406,
#50407,#50408,#50409,#50410,#50411,#50412,#50413,#50414,#50415,#50416)),
 .UNSPECIFIED.,.F.,.F.,.F.,(4,4),(4,1,1,1,1,1,1,1,1,1,1,1,1,1,1,1,1,1,1,
1,1,1,1,1,1,1,1,1,1,1,1,1,1,1,1,1,1,1,1,1,1,1,1,1,1,1,1,1,1,1,1,1,1,1,1,
1,1,1,1,1,1,1,1,1,1,1,1,1,1,1,1,1,1,1,1,1,1,4),(0.,0.0296469363228873),
(15.803923819236,16.791868064592,17.779812309948,18.767756555304,19.7557008006601,
20.7436450460161,21.7315892913721,22.7195335367281,23.7074777820841,24.6954220274402,
25.6833662727962,26.6713105181522,27.6592547635082,28.6471990088642,29.6351432542203,
30.6230874995763,31.6110317449323,32.5989759902883,33.5869202356443,34.5748644810004,
35.5628087263564,36.5507529717124,37.5386972170684,38.5266414624244,39.5145857077805,
40.5025299531365,41.4904741984925,42.4784184438485,43.4663626892045,44.4543069345606,
45.4422511799166,46.4301954252726,47.4181396706286,48.4060839159846,49.3940281613407,
50.3819724066967,51.3699166520527,52.3578608974087,53.3458051427647,54.3337493881208,
55.3216936334768,56.3096378788328,57.2975821241888,58.2855263695448,59.2734706149009,
60.2614148602569,61.2493591056129,62.2373033509689,63.2252475963249,64.213191841681,
65.201136087037,66.189080332393,67.177024577749,68.164968823105,69.1529130684611,
70.1408573138171,71.1288015591731,72.1167458045291,73.1046900498851,74.0926342952412,
75.0805785405972,76.0685227859532,77.0564670313092,78.0444112766652,79.0323555220213,
80.0202997673773,81.0082440127333,81.9961882580893,82.9841325034453,83.9720767488014,
84.9600209941574,85.9479652395134,86.9359094848694,87.9238537302254,88.9117979755815,
89.8997422209375,90.8876864662935,91.8756307116495),.UNSPECIFIED.);
#790=B_SPLINE_CURVE_WITH_KNOTS('',3,(#48675,#48676,#48677,#48678,#48679,
#48680,#48681,#48682,#48683,#48684,#48685,#48686,#48687,#48688,#48689,#48690),
 .UNSPECIFIED.,.F.,.F.,(4,3,3,3,3,4),(-6.1872247558925,-5.92766547213612,
-4.9397212267801,-3.95177698142408,-2.96383273606806,-2.06974660785395),
 .UNSPECIFIED.);
#791=B_SPLINE_CURVE_WITH_KNOTS('',3,(#48698,#48699,#48700,#48701,#48702,
#48703,#48704,#48705,#48706,#48707,#48708,#48709,#48710),.UNSPECIFIED.,
 .F.,.F.,(4,3,3,3,4),(0.,0.987944245356008,1.97588849071203,2.96383273606806,
3.21290471033757),.UNSPECIFIED.);
#792=B_SPLINE_CURVE_WITH_KNOTS('',3,(#48715,#48716,#48717,#48718,#48719,
#48720,#48721,#48722,#48723,#48724,#48725,#48726,#48727,#48728,#48729,#48730,
#48731,#48732,#48733,#48734,#48735,#48736),.UNSPECIFIED.,.F.,.F.,(4,3,3,
3,3,3,3,4),(-12.4704100630721,-11.8553309442722,-10.8673866989162,-9.8794424535602,
-8.89149820820418,-7.90355396284816,-6.91560971749214,-6.1872247558925),
 .UNSPECIFIED.);
#793=B_SPLINE_CURVE_WITH_KNOTS('',3,(#48737,#48738,#48739,#48740,#48741,
#48742,#48743,#48744,#48745,#48746,#48747,#48748,#48749,#48750,#48751,#48752,
#48753,#48754,#48755,#48756,#48757,#48758),.UNSPECIFIED.,.F.,.F.,(4,3,3,
3,3,3,3,4),(3.21290471033757,3.95177698142408,4.9397212267801,5.92766547213613,
6.91560971749214,7.90355396284817,8.89149820820418,9.49609001751715),
 .UNSPECIFIED.);
#794=B_SPLINE_CURVE_WITH_KNOTS('',3,(#48763,#48764,#48765,#48766,#48767,
#48768,#48769,#48770,#48771,#48772,#48773,#48774,#48775,#48776,#48777,#48778,
#48779,#48780,#48781,#48782,#48783,#48784),.UNSPECIFIED.,.F.,.F.,(4,3,3,
3,3,3,3,4),(-18.7535953702517,-17.7829964164084,-16.7950521710523,-15.8071079256963,
-14.8191636803403,-13.8312194349843,-12.8432751896283,-12.4704100630721),
 .UNSPECIFIED.);
#795=B_SPLINE_CURVE_WITH_KNOTS('',3,(#48785,#48786,#48787,#48788,#48789,
#48790,#48791,#48792,#48793,#48794,#48795,#48796,#48797,#48798,#48799,#48800,
#48801,#48802,#48803,#48804,#48805,#48806),.UNSPECIFIED.,.F.,.F.,(4,3,3,
3,3,3,3,4),(9.49609001751715,9.8794424535602,10.8673866989162,11.8553309442722,
12.8432751896283,13.8312194349843,14.8191636803403,15.7792753246967),
 .UNSPECIFIED.);
#796=B_SPLINE_CURVE_WITH_KNOTS('',3,(#48811,#48812,#48813,#48814,#48815,
#48816,#48817,#48818,#48819,#48820,#48821,#48822,#48823,#48824,#48825,#48826,
#48827,#48828,#48829,#48830,#48831,#48832,#48833,#48834,#48835),
 .UNSPECIFIED.,.F.,.F.,(4,3,3,3,3,3,3,3,4),(-25.0367806774313,-24.6986061339005,
-23.7106618885445,-22.7227176431885,-21.7347733978324,-20.7468291524764,
-19.7588849071204,-18.7709406617644,-18.7535953702517),.UNSPECIFIED.);
#797=B_SPLINE_CURVE_WITH_KNOTS('',3,(#48836,#48837,#48838,#48839,#48840,
#48841,#48842,#48843,#48844,#48845,#48846,#48847,#48848,#48849,#48850,#48851,
#48852,#48853,#48854,#48855,#48856,#48857,#48858,#48859,#48860),
 .UNSPECIFIED.,.F.,.F.,(4,3,3,3,3,3,3,3,4),(15.7792753246967,15.8071079256963,
16.7950521710523,17.7829964164084,18.7709406617644,19.7588849071204,20.7468291524764,
21.7347733978324,22.0624606318763),.UNSPECIFIED.);
#798=B_SPLINE_CURVE_WITH_KNOTS('',3,(#48865,#48866,#48867,#48868,#48869,
#48870,#48871,#48872,#48873,#48874,#48875,#48876,#48877,#48878,#48879,#48880,
#48881,#48882,#48883,#48884,#48885,#48886),.UNSPECIFIED.,.F.,.F.,(4,3,3,
3,3,3,3,4),(-31.3199659846109,-30.6262716060366,-29.6383273606806,-28.6503831153246,
-27.6624388699686,-26.6744946246125,-25.6865503792565,-25.0367806774313),
 .UNSPECIFIED.);
#799=B_SPLINE_CURVE_WITH_KNOTS('',3,(#48887,#48888,#48889,#48890,#48891,
#48892,#48893,#48894,#48895,#48896,#48897,#48898,#48899,#48900,#48901,#48902,
#48903,#48904,#48905,#48906,#48907,#48908),.UNSPECIFIED.,.F.,.F.,(4,3,3,
3,3,3,3,4),(22.0624606318763,22.7227176431885,23.7106618885445,24.6986061339005,
25.6865503792565,26.6744946246125,27.6624388699686,28.3456459390559),
 .UNSPECIFIED.);
#800=B_SPLINE_CURVE_WITH_KNOTS('',3,(#48913,#48914,#48915,#48916,#48917,
#48918,#48919,#48920,#48921,#48922,#48923,#48924,#48925,#48926,#48927,#48928,
#48929,#48930,#48931,#48932,#48933,#48934,#48935,#48936,#48937),
 .UNSPECIFIED.,.F.,.F.,(4,3,3,3,3,3,3,3,4),(-37.6031512917904,-37.5418813235288,
-36.5539370781727,-35.5659928328167,-34.5780485874607,-33.5901043421047,
-32.6021600967487,-31.6142158513926,-31.3199659846109),.UNSPECIFIED.);
#801=B_SPLINE_CURVE_WITH_KNOTS('',3,(#48938,#48939,#48940,#48941,#48942,
#48943,#48944,#48945,#48946,#48947,#48948,#48949,#48950,#48951,#48952,#48953,
#48954,#48955,#48956,#48957,#48958,#48959,#48960,#48961,#48962),
 .UNSPECIFIED.,.F.,.F.,(4,3,3,3,3,3,3,3,4),(28.3456459390559,28.6503831153246,
29.6383273606806,30.6262716060366,31.6142158513926,32.6021600967487,33.5901043421047,
34.5780485874607,34.6288312462355),.UNSPECIFIED.);
#802=B_SPLINE_CURVE_WITH_KNOTS('',3,(#48967,#48968,#48969,#48970,#48971,
#48972,#48973,#48974,#48975,#48976,#48977,#48978,#48979,#48980,#48981,#48982,
#48983,#48984,#48985,#48986,#48987,#48988),.UNSPECIFIED.,.F.,.F.,(4,3,3,
3,3,3,3,4),(-43.88633659897,-43.4695467956649,-42.4816025503089,-41.4936583049528,
-40.5057140595968,-39.5177698142408,-38.5298255688848,-37.6031512917904),
 .UNSPECIFIED.);
#803=B_SPLINE_CURVE_WITH_KNOTS('',3,(#48989,#48990,#48991,#48992,#48993,
#48994,#48995,#48996,#48997,#48998,#48999,#49000,#49001,#49002,#49003,#49004,
#49005,#49006,#49007,#49008,#49009,#49010),.UNSPECIFIED.,.F.,.F.,(4,3,3,
3,3,3,3,4),(34.6288312462355,35.5659928328167,36.5539370781727,37.5418813235288,
38.5298255688848,39.5177698142408,40.5057140595968,40.9120165534151),
 .UNSPECIFIED.);
#804=B_SPLINE_CURVE_WITH_KNOTS('',3,(#49015,#49016,#49017,#49018,#49019,
#49020,#49021,#49022,#49023,#49024,#49025,#49026,#49027,#49028,#49029,#49030,
#49031,#49032,#49033,#49034,#49035,#49036),.UNSPECIFIED.,.F.,.F.,(4,3,3,
3,3,3,3,4),(-50.1695219061496,-49.397212267801,-48.409268022445,-47.421323777089,
-46.4333795317329,-45.4454352863769,-44.4574910410209,-43.88633659897),
 .UNSPECIFIED.);
#805=B_SPLINE_CURVE_WITH_KNOTS('',3,(#49037,#49038,#49039,#49040,#49041,
#49042,#49043,#49044,#49045,#49046,#49047,#49048,#49049,#49050,#49051,#49052,
#49053,#49054,#49055,#49056,#49057,#49058),.UNSPECIFIED.,.F.,.F.,(4,3,3,
3,3,3,3,4),(40.9120165534151,41.4936583049528,42.4816025503089,43.4695467956649,
44.4574910410209,45.4454352863769,46.4333795317329,47.1952018605947),
 .UNSPECIFIED.);
#806=B_SPLINE_CURVE_WITH_KNOTS('',3,(#49063,#49064,#49065,#49066,#49067,
#49068,#49069,#49070,#49071,#49072,#49073,#49074,#49075,#49076,#49077,#49078,
#49079,#49080,#49081,#49082,#49083,#49084,#49085,#49086,#49087),
 .UNSPECIFIED.,.F.,.F.,(4,3,3,3,3,3,3,3,4),(-56.4527072133292,-56.3128219852932,
-55.3248777399371,-54.3369334945811,-53.3489892492251,-52.3610450038691,
-51.373100758513,-50.385156513157,-50.1695219061496),.UNSPECIFIED.);
#807=B_SPLINE_CURVE_WITH_KNOTS('',3,(#49088,#49089,#49090,#49091,#49092,
#49093,#49094,#49095,#49096,#49097,#49098,#49099,#49100,#49101,#49102,#49103,
#49104,#49105,#49106,#49107,#49108,#49109,#49110,#49111,#49112),
 .UNSPECIFIED.,.F.,.F.,(4,3,3,3,3,3,3,3,4),(47.1952018605947,47.421323777089,
48.409268022445,49.397212267801,50.385156513157,51.373100758513,52.3610450038691,
53.3489892492251,53.4783871677743),.UNSPECIFIED.);
#808=B_SPLINE_CURVE_WITH_KNOTS('',3,(#49117,#49118,#49119,#49120,#49121,
#49122,#49123,#49124,#49125,#49126,#49127,#49128,#49129,#49130,#49131,#49132,
#49133,#49134,#49135,#49136,#49137,#49138),.UNSPECIFIED.,.F.,.F.,(4,3,3,
3,3,3,3,4),(-62.7358925205088,-62.2404874574293,-61.2525432120733,-60.2645989667172,
-59.2766547213612,-58.2887104760052,-57.3007662306492,-56.4527072133292),
 .UNSPECIFIED.);
#809=B_SPLINE_CURVE_WITH_KNOTS('',3,(#49139,#49140,#49141,#49142,#49143,
#49144,#49145,#49146,#49147,#49148,#49149,#49150,#49151,#49152,#49153,#49154,
#49155,#49156,#49157,#49158,#49159,#49160),.UNSPECIFIED.,.F.,.F.,(4,3,3,
3,3,3,3,4),(53.4783871677743,54.3369334945811,55.3248777399371,56.3128219852931,
57.3007662306492,58.2887104760052,59.2766547213612,59.7615724749539),
 .UNSPECIFIED.);
#810=B_SPLINE_CURVE_WITH_KNOTS('',3,(#49165,#49166,#49167,#49168,#49169,
#49170,#49171,#49172,#49173,#49174,#49175,#49176,#49177,#49178,#49179,#49180,
#49181,#49182,#49183,#49184,#49185,#49186),.UNSPECIFIED.,.F.,.F.,(4,3,3,
3,3,3,3,4),(-69.0190778276884,-68.1681529295654,-67.1802086842094,-66.1922644388533,
-65.2043201934973,-64.2163759481413,-63.2284317027853,-62.7358925205088),
 .UNSPECIFIED.);
#811=B_SPLINE_CURVE_WITH_KNOTS('',3,(#49187,#49188,#49189,#49190,#49191,
#49192,#49193,#49194,#49195,#49196,#49197,#49198,#49199,#49200,#49201,#49202,
#49203,#49204,#49205,#49206,#49207,#49208),.UNSPECIFIED.,.F.,.F.,(4,3,3,
3,3,3,3,4),(59.7615724749539,60.2645989667172,61.2525432120732,62.2404874574293,
63.2284317027853,64.2163759481413,65.2043201934973,66.0447577821335),
 .UNSPECIFIED.);
#812=B_SPLINE_CURVE_WITH_KNOTS('',3,(#49213,#49214,#49215,#49216,#49217,
#49218,#49219,#49220,#49221,#49222,#49223,#49224,#49225,#49226,#49227,#49228,
#49229,#49230,#49231,#49232,#49233,#49234,#49235,#49236,#49237),
 .UNSPECIFIED.,.F.,.F.,(4,3,3,3,3,3,3,3,4),(-75.302263134868,-75.0837626470575,
-74.0958184017015,-73.1078741563455,-72.1199299109895,-71.1319856656335,
-70.1440414202774,-69.1560971749214,-69.0190778276884),.UNSPECIFIED.);
#813=B_SPLINE_CURVE_WITH_KNOTS('',3,(#49238,#49239,#49240,#49241,#49242,
#49243,#49244,#49245,#49246,#49247,#49248,#49249,#49250,#49251,#49252,#49253,
#49254,#49255,#49256,#49257,#49258,#49259,#49260,#49261,#49262),
 .UNSPECIFIED.,.F.,.F.,(4,3,3,3,3,3,3,3,4),(66.0447577821335,66.1922644388533,
67.1802086842094,68.1681529295654,69.1560971749214,70.1440414202774,71.1319856656334,
72.1199299109894,72.3279430893131),.UNSPECIFIED.);
#814=B_SPLINE_CURVE_WITH_KNOTS('',3,(#49268,#49269,#49270,#49271,#49272,
#49273,#49274,#49275,#49276),.UNSPECIFIED.,.F.,.F.,(4,1,1,1,1,1,4),(84.8230016469244,
84.9600209941574,85.9479652395134,86.9359094848694,87.9238537302254,88.9117979755815,
89.8058841037956),.UNSPECIFIED.);
#815=B_SPLINE_CURVE_WITH_KNOTS('',3,(#49279,#49280,#49281,#49282,#49283,
#49284,#49285),.UNSPECIFIED.,.F.,.F.,(4,1,1,1,4),(84.8230016469244,85.6029327139567,
86.5908769593128,87.5788212046688,88.5667654500248),.UNSPECIFIED.);
#816=B_SPLINE_CURVE_WITH_KNOTS('',3,(#49290,#49291,#49292,#49293,#49294,
#49295,#49296,#49297,#49298,#49299),.UNSPECIFIED.,.F.,.F.,(4,1,1,1,1,1,
1,4),(78.5398163397448,79.0323555220213,80.0202997673773,81.0082440127333,
81.9961882580893,82.9841325034453,83.9720767488014,84.8230016469244),
 .UNSPECIFIED.);
#817=B_SPLINE_CURVE_WITH_KNOTS('',3,(#49300,#49301,#49302,#49303,#49304,
#49305,#49306,#49307,#49308,#49309,#49310),.UNSPECIFIED.,.F.,.F.,(4,1,1,
1,1,1,1,1,4),(78.5398163397448,78.6873229964646,79.6752672418206,80.6632114871766,
81.6511557325327,82.6390999778887,83.6270442232447,84.6149884686007,84.8230016469244),
 .UNSPECIFIED.);
#818=B_SPLINE_CURVE_WITH_KNOTS('',3,(#49315,#49316,#49317,#49318,#49319,
#49320,#49321,#49322,#49323,#49324),.UNSPECIFIED.,.F.,.F.,(4,1,1,1,1,1,
1,4),(72.2566310325652,73.1046900498851,74.0926342952412,75.0805785405972,
76.0685227859532,77.0564670313092,78.0444112766652,78.5398163397448),
 .UNSPECIFIED.);
#819=B_SPLINE_CURVE_WITH_KNOTS('',3,(#49325,#49326,#49327,#49328,#49329,
#49330,#49331,#49332,#49333,#49334),.UNSPECIFIED.,.F.,.F.,(4,1,1,1,1,1,
1,4),(72.2566310325652,72.7596575243285,73.7476017696845,74.7355460150405,
75.7234902603965,76.7114345057526,77.6993787511086,78.5398163397448),
 .UNSPECIFIED.);
#820=B_SPLINE_CURVE_WITH_KNOTS('',3,(#49339,#49340,#49341,#49342,#49343,
#49344,#49345,#49346,#49347,#49348,#49349),.UNSPECIFIED.,.F.,.F.,(4,1,1,
1,1,1,1,1,4),(65.9734457253856,66.189080332393,67.177024577749,68.164968823105,
69.1529130684611,70.1408573138171,71.1288015591731,72.1167458045291,72.2566310325652),
 .UNSPECIFIED.);
#821=B_SPLINE_CURVE_WITH_KNOTS('',3,(#49350,#49351,#49352,#49353,#49354,
#49355,#49356,#49357,#49358,#49359),.UNSPECIFIED.,.F.,.F.,(4,1,1,1,1,1,
1,4),(65.9734457253856,66.8319920521924,67.8199362975484,68.8078805429044,
69.7958247882604,70.7837690336165,71.7717132789725,72.2566310325652),
 .UNSPECIFIED.);
#822=B_SPLINE_CURVE_WITH_KNOTS('',3,(#49364,#49365,#49366,#49367,#49368,
#49369,#49370,#49371,#49372,#49373),.UNSPECIFIED.,.F.,.F.,(4,1,1,1,1,1,
1,4),(59.6902604182061,60.2614148602569,61.2493591056129,62.2373033509689,
63.2252475963249,64.213191841681,65.201136087037,65.9734457253856),
 .UNSPECIFIED.);
#823=B_SPLINE_CURVE_WITH_KNOTS('',3,(#49374,#49375,#49376,#49377,#49378,
#49379,#49380,#49381,#49382,#49383,#49384),.UNSPECIFIED.,.F.,.F.,(4,1,1,
1,1,1,1,1,4),(59.690260418206,59.9163823347002,60.9043265800563,61.8922708254123,
62.8802150707683,63.8681593161243,64.8561035614803,65.8440478068363,65.9734457253856),
 .UNSPECIFIED.);
#824=B_SPLINE_CURVE_WITH_KNOTS('',3,(#49389,#49390,#49391,#49392,#49393,
#49394,#49395,#49396,#49397,#49398),.UNSPECIFIED.,.F.,.F.,(4,1,1,1,1,1,
1,4),(53.4070751110265,54.3337493881208,55.3216936334768,56.3096378788328,
57.2975821241888,58.2855263695448,59.2734706149009,59.6902604182061),
 .UNSPECIFIED.);
#825=B_SPLINE_CURVE_WITH_KNOTS('',3,(#49399,#49400,#49401,#49402,#49403,
#49404,#49405,#49406,#49407,#49408),.UNSPECIFIED.,.F.,.F.,(4,1,1,1,1,1,
1,4),(53.4070751110264,53.9887168625641,54.9766611079201,55.9646053532762,
56.9525495986322,57.9404938439882,58.9284380893442,59.690260418206),
 .UNSPECIFIED.);
#826=B_SPLINE_CURVE_WITH_KNOTS('',3,(#49413,#49414,#49415,#49416,#49417,
#49418,#49419,#49420,#49421,#49422,#49423),.UNSPECIFIED.,.F.,.F.,(4,1,1,
1,1,1,1,1,4),(47.1238898038469,47.4181396706286,48.4060839159846,49.3940281613407,
50.3819724066967,51.3699166520527,52.3578608974087,53.3458051427647,53.4070751110265),
 .UNSPECIFIED.);
#827=B_SPLINE_CURVE_WITH_KNOTS('',3,(#49424,#49425,#49426,#49427,#49428,
#49429,#49430,#49431,#49432,#49433),.UNSPECIFIED.,.F.,.F.,(4,1,1,1,1,1,
1,4),(47.1238898038469,48.061051390428,49.048995635784,50.03693988114,51.0248841264961,
52.0128283718521,53.0007726172081,53.4070751110264),.UNSPECIFIED.);
#828=B_SPLINE_CURVE_WITH_KNOTS('',3,(#49438,#49439,#49440,#49441,#49442,
#49443,#49444,#49445,#49446,#49447),.UNSPECIFIED.,.F.,.F.,(4,1,1,1,1,1,
1,4),(40.8407044966673,41.4904741984925,42.4784184438485,43.4663626892045,
44.4543069345606,45.4422511799166,46.4301954252726,47.1238898038469),
 .UNSPECIFIED.);
#829=B_SPLINE_CURVE_WITH_KNOTS('',3,(#49448,#49449,#49450,#49451,#49452,
#49453,#49454,#49455,#49456,#49457,#49458),.UNSPECIFIED.,.F.,.F.,(4,1,1,
1,1,1,1,1,4),(40.8407044966673,41.1454416729359,42.1333859182919,43.1213301636479,
44.1092744090039,45.0972186543599,46.085162899716,47.073107145072,47.1238898038469),
 .UNSPECIFIED.);
#830=B_SPLINE_CURVE_WITH_KNOTS('',3,(#49463,#49464,#49465,#49466,#49467,
#49468,#49469,#49470,#49471,#49472,#49473),.UNSPECIFIED.,.F.,.F.,(4,1,1,
1,1,1,1,1,4),(34.5575191894877,34.5748644810004,35.5628087263564,36.5507529717124,
37.5386972170684,38.5266414624244,39.5145857077805,40.5025299531365,40.8407044966673),
 .UNSPECIFIED.);
#831=B_SPLINE_CURVE_WITH_KNOTS('',3,(#49474,#49475,#49476,#49477,#49478,
#49479,#49480,#49481,#49482,#49483),.UNSPECIFIED.,.F.,.F.,(4,1,1,1,1,1,
1,4),(34.5575191894877,35.2177762007997,36.2057204461558,37.1936646915118,
38.1816089368678,39.1695531822238,40.1574974275798,40.8407044966673),
 .UNSPECIFIED.);
#832=B_SPLINE_CURVE_WITH_KNOTS('',3,(#49488,#49489,#49490,#49491,#49492,
#49493,#49494,#49495,#49496,#49497),.UNSPECIFIED.,.F.,.F.,(4,1,1,1,1,1,
1,4),(28.2743338823081,28.6471990088642,29.6351432542203,30.6230874995763,
31.6110317449323,32.5989759902883,33.5869202356443,34.5575191894877),
 .UNSPECIFIED.);
#833=B_SPLINE_CURVE_WITH_KNOTS('',3,(#49498,#49499,#49500,#49501,#49502,
#49503,#49504,#49505,#49506,#49507,#49508),.UNSPECIFIED.,.F.,.F.,(4,1,1,
1,1,1,1,1,4),(28.2743338823081,28.3021664833076,29.2901107286636,30.2780549740196,
31.2659992193757,32.2539434647317,33.2418877100877,34.2298319554437,34.5575191894877),
 .UNSPECIFIED.);
#834=B_SPLINE_CURVE_WITH_KNOTS('',3,(#49513,#49514,#49515,#49516,#49517,
#49518,#49519,#49520,#49521,#49522),.UNSPECIFIED.,.F.,.F.,(4,1,1,1,1,1,
1,4),(21.9911485751285,22.7195335367281,23.7074777820841,24.6954220274402,
25.6833662727962,26.6713105181522,27.6592547635082,28.2743338823081),
 .UNSPECIFIED.);
#835=B_SPLINE_CURVE_WITH_KNOTS('',3,(#49523,#49524,#49525,#49526,#49527,
#49528,#49529,#49530,#49531,#49532),.UNSPECIFIED.,.F.,.F.,(4,1,1,1,1,1,
1,4),(21.9911485751285,22.3745010111715,23.3624452565275,24.3503895018835,
25.3383337472395,26.3262779925956,27.3142222379516,28.2743338823081),
 .UNSPECIFIED.);
#836=B_SPLINE_CURVE_WITH_KNOTS('',3,(#49539,#49540,#49541,#49542,#49543,
#49544,#49545,#49546,#49547,#49548),.UNSPECIFIED.,.F.,.F.,(4,1,1,1,1,1,
1,4),(15.803923819236,16.791868064592,17.779812309948,18.767756555304,19.7557008006601,
20.7436450460161,21.7315892913721,21.9911485751285),.UNSPECIFIED.);
#837=B_SPLINE_CURVE_WITH_KNOTS('',3,(#49549,#49550,#49551,#49552,#49553,
#49554,#49555,#49556,#49557,#49558),.UNSPECIFIED.,.F.,.F.,(4,1,1,1,1,1,
1,4),(15.7079632679489,16.4468355390354,17.4347797843914,18.4227240297474,
19.4106682751034,20.3986125204594,21.3865567658155,21.9911485751285),
 .UNSPECIFIED.);
#838=B_SPLINE_CURVE_WITH_KNOTS('',3,(#49561,#49562,#49563,#49564,#49565,
#49566,#49567,#49568,#49569,#49570,#49571,#49572,#49573,#49574,#49575,#49576,
#49577,#49578,#49579,#49580,#49581,#49582,#49583,#49584,#49585,#49586,#49587,
#49588,#49589,#49590,#49591,#49592,#49593,#49594,#49595,#49596,#49597,#49598,
#49599,#49600,#49601,#49602,#49603,#49604,#49605,#49606,#49607,#49608,#49609),
 .UNSPECIFIED.,.F.,.F.,(4,3,3,3,3,3,3,3,3,3,3,3,3,3,3,3,4),(-0.227523845437324,
-0.218350149341661,-0.205842204254971,-0.194305484443851,-0.180954054603224,
-0.167897350901462,-0.143373661203175,-0.133616778871748,-0.125537010422148,
-0.115138897237553,-0.0973810329882545,-0.0847723556366763,-0.0635792667275072,
-0.0502539163266662,-0.0410435569307654,-0.0141179092232515,0.),
 .UNSPECIFIED.);
#839=B_SPLINE_CURVE_WITH_KNOTS('',3,(#49614,#49615,#49616,#49617,#49618,
#49619,#49620,#49621,#49622,#49623,#49624,#49625,#49626,#49627,#49628,#49629,
#49630,#49631,#49632,#49633,#49634,#49635,#49636,#49637,#49638,#49639,#49640,
#49641,#49642,#49643,#49644,#49645,#49646,#49647,#49648,#49649,#49650,#49651,
#49652,#49653,#49654,#49655,#49656,#49657,#49658,#49659,#49660,#49661,#49662),
 .UNSPECIFIED.,.F.,.F.,(4,3,3,3,3,3,3,3,3,3,3,3,3,3,3,3,4),(-0.226379821609596,
-0.215007753384842,-0.195255307837548,-0.183767362539732,-0.169423470115966,
-0.156758753808324,-0.131327701983312,-0.121202735143442,-0.113669834739438,
-0.101656477907397,-0.0859751299016101,-0.0772104628791785,-0.0531806453069207,
-0.0418075009839797,-0.032303590237005,-0.00987926401158647,0.),
 .UNSPECIFIED.);
#840=B_SPLINE_CURVE_WITH_KNOTS('',3,(#49983,#49984,#49985,#49986,#49987,
#49988,#49989),.UNSPECIFIED.,.F.,.F.,(4,3,4),(72.3279430893131,73.1078741563455,
74.0019602845596),.UNSPECIFIED.);
#841=B_SPLINE_CURVE_WITH_KNOTS('',3,(#49991,#49992,#49993,#49994,#49995,
#49996,#49997,#49998,#49999,#50000,#50001,#50002,#50003,#50004,#50005,#50006,
#50007,#50008,#50009,#50010,#50011,#50012,#50013,#50014,#50015,#50016,#50017,
#50018,#50019,#50020,#50021,#50022,#50023,#50024,#50025,#50026,#50027,#50028,
#50029,#50030,#50031,#50032,#50033,#50034,#50035,#50036,#50037,#50038,#50039),
 .UNSPECIFIED.,.F.,.F.,(4,3,3,3,3,3,3,3,3,3,3,3,3,3,3,3,4),(-0.227523845437316,
-0.218350149341655,-0.205842197866321,-0.194305484374478,-0.180954006819641,
-0.167897358466276,-0.143373669279798,-0.133616834209574,-0.125537019650691,
-0.115138897237547,-0.097381026810668,-0.0847723567113073,-0.0635792675334805,
-0.0502539177590211,-0.0410435559730182,-0.0141179048973905,0.),
 .UNSPECIFIED.);
#842=B_SPLINE_CURVE_WITH_KNOTS('',3,(#50040,#50041,#50042,#50043,#50044),
 .UNSPECIFIED.,.F.,.F.,(4,1,4),(14.5648051654652,15.4588912936793,15.7079632679489),
 .UNSPECIFIED.);
#843=B_SPLINE_CURVE_WITH_KNOTS('',3,(#50046,#50047,#50048,#50049,#50050,
#50051,#50052,#50053,#50054,#50055,#50056,#50057,#50058,#50059,#50060,#50061,
#50062,#50063,#50064,#50065,#50066,#50067,#50068,#50069,#50070,#50071,#50072,
#50073,#50074,#50075,#50076,#50077,#50078,#50079,#50080,#50081,#50082,#50083,
#50084,#50085,#50086,#50087,#50088,#50089,#50090,#50091,#50092,#50093,#50094),
 .UNSPECIFIED.,.F.,.F.,(4,3,3,3,3,3,3,3,3,3,3,3,3,3,3,3,4),(-0.226379821609599,
-0.215007753384844,-0.19525530446945,-0.183767359662995,-0.169423451536204,
-0.156758753435164,-0.131327696656529,-0.121202706406611,-0.113669787610754,
-0.101656477907395,-0.0859751252241449,-0.077210461042814,-0.0531806474590482,
-0.0418075086540048,-0.032303593576968,-0.00987927928781002,0.),
 .UNSPECIFIED.);
#844=B_SPLINE_CURVE_WITH_KNOTS('',3,(#50417,#50418,#50419,#50420),
 .UNSPECIFIED.,.F.,.F.,(4,4),(-76.0717068924135,-75.302263134868),
 .UNSPECIFIED.);
#973=SHAPE_REPRESENTATION_RELATIONSHIP('SRR','None',#55121,#993);
#993=ADVANCED_BREP_SHAPE_REPRESENTATION('',(#1033),#54999);
#1013=STYLED_ITEM('',(#55393),#1033);
#1033=MANIFOLD_SOLID_BREP('ISO_4762_M2.5x6_A2',#24546);
#1269=FACE_BOUND('',#5272,.T.);
#1270=FACE_BOUND('',#5277,.T.);
#1271=FACE_BOUND('',#5279,.T.);
#1798=PLANE('',#26816);
#1799=PLANE('',#26819);
#1800=PLANE('',#26824);
#1801=PLANE('',#26826);
#1802=PLANE('',#26827);
#1803=PLANE('',#26828);
#1804=PLANE('',#26830);
#1805=PLANE('',#26831);
#1806=PLANE('',#26832);
#1807=PLANE('',#26834);
#1808=PLANE('',#26835);
#1809=PLANE('',#26836);
#1810=PLANE('',#26838);
#1811=PLANE('',#26839);
#1812=PLANE('',#26840);
#1813=PLANE('',#26842);
#1814=PLANE('',#26843);
#1815=PLANE('',#26844);
#1816=PLANE('',#26846);
#1817=PLANE('',#26847);
#1818=PLANE('',#26848);
#1819=PLANE('',#26850);
#1820=PLANE('',#26851);
#1821=PLANE('',#26852);
#1822=PLANE('',#26854);
#1823=PLANE('',#26855);
#1824=PLANE('',#26856);
#1825=PLANE('',#26858);
#1826=PLANE('',#26859);
#1827=PLANE('',#26860);
#1828=PLANE('',#26862);
#1829=PLANE('',#26863);
#1830=PLANE('',#26864);
#1831=PLANE('',#26866);
#1832=PLANE('',#26867);
#1833=PLANE('',#26868);
#1834=PLANE('',#26870);
#1835=PLANE('',#26871);
#1836=PLANE('',#26872);
#1837=PLANE('',#26874);
#1838=PLANE('',#26875);
#1839=PLANE('',#26876);
#1840=PLANE('',#26878);
#1841=PLANE('',#26879);
#1842=PLANE('',#26880);
#1843=PLANE('',#26882);
#1844=PLANE('',#26883);
#1845=PLANE('',#26884);
#1846=PLANE('',#26886);
#1847=PLANE('',#26887);
#1848=PLANE('',#26888);
#1849=PLANE('',#26890);
#1850=PLANE('',#26891);
#1851=PLANE('',#26892);
#1852=PLANE('',#26895);
#1853=PLANE('',#26896);
#1854=PLANE('',#26897);
#1855=PLANE('',#26899);
#1856=PLANE('',#26900);
#1857=PLANE('',#26901);
#1858=PLANE('',#26903);
#1859=PLANE('',#26904);
#1860=PLANE('',#26905);
#1861=PLANE('',#26907);
#1862=PLANE('',#26908);
#1863=PLANE('',#26909);
#1864=PLANE('',#26911);
#1865=PLANE('',#26912);
#1866=PLANE('',#26913);
#1867=PLANE('',#26915);
#1868=PLANE('',#26916);
#1869=PLANE('',#26917);
#1870=PLANE('',#26919);
#1871=PLANE('',#26920);
#1872=PLANE('',#26921);
#1873=PLANE('',#26923);
#1874=PLANE('',#26924);
#1875=PLANE('',#26925);
#1876=PLANE('',#26927);
#1877=PLANE('',#26928);
#1878=PLANE('',#26929);
#1879=PLANE('',#26931);
#1880=PLANE('',#26932);
#1881=PLANE('',#26933);
#1882=PLANE('',#26935);
#1883=PLANE('',#26936);
#1884=PLANE('',#26937);
#1885=PLANE('',#26939);
#1886=PLANE('',#26940);
#1887=PLANE('',#26941);
#1888=PLANE('',#26943);
#1889=PLANE('',#26944);
#1890=PLANE('',#26945);
#1891=PLANE('',#26947);
#1892=PLANE('',#26948);
#1893=PLANE('',#26949);
#1894=PLANE('',#26951);
#1895=PLANE('',#26952);
#1896=PLANE('',#26953);
#1897=PLANE('',#26955);
#1898=PLANE('',#26956);
#1899=PLANE('',#26957);
#1900=PLANE('',#26959);
#1901=PLANE('',#26960);
#1902=PLANE('',#26961);
#1903=PLANE('',#26963);
#1904=PLANE('',#26964);
#1905=PLANE('',#27004);
#1906=PLANE('',#27005);
#1907=PLANE('',#27006);
#1908=PLANE('',#27011);
#1909=PLANE('',#27012);
#1910=PLANE('',#27013);
#1911=PLANE('',#27014);
#1912=PLANE('',#27015);
#1913=PLANE('',#27016);
#1914=PLANE('',#27017);
#1915=PLANE('',#27018);
#1916=PLANE('',#27023);
#1917=PLANE('',#27024);
#2331=CYLINDRICAL_SURFACE('',#26787,0.1215);
#2332=CYLINDRICAL_SURFACE('',#26791,0.1215);
#2333=CYLINDRICAL_SURFACE('',#26792,0.1215);
#2334=CYLINDRICAL_SURFACE('',#26793,0.1215);
#2335=CYLINDRICAL_SURFACE('',#26794,0.1215);
#2336=CYLINDRICAL_SURFACE('',#26795,0.1215);
#2337=CYLINDRICAL_SURFACE('',#26796,0.1215);
#2338=CYLINDRICAL_SURFACE('',#26797,0.1215);
#2339=CYLINDRICAL_SURFACE('',#26798,0.1215);
#2340=CYLINDRICAL_SURFACE('',#26799,0.1215);
#2341=CYLINDRICAL_SURFACE('',#26800,0.1215);
#2342=CYLINDRICAL_SURFACE('',#26801,0.1215);
#2343=CYLINDRICAL_SURFACE('',#26802,0.095825);
#2344=CYLINDRICAL_SURFACE('',#26804,0.095825);
#2345=CYLINDRICAL_SURFACE('',#26805,0.095825);
#2346=CYLINDRICAL_SURFACE('',#26806,0.095825);
#2347=CYLINDRICAL_SURFACE('',#26807,0.095825);
#2348=CYLINDRICAL_SURFACE('',#26808,0.095825);
#2349=CYLINDRICAL_SURFACE('',#26809,0.095825);
#2350=CYLINDRICAL_SURFACE('',#26810,0.095825);
#2351=CYLINDRICAL_SURFACE('',#26811,0.095825);
#2352=CYLINDRICAL_SURFACE('',#26812,0.095825);
#2353=CYLINDRICAL_SURFACE('',#26813,0.095825);
#2354=CYLINDRICAL_SURFACE('',#26814,0.095825);
#2355=CYLINDRICAL_SURFACE('',#26821,0.095825);
#2356=CYLINDRICAL_SURFACE('',#26822,0.1215);
#2357=CYLINDRICAL_SURFACE('',#26965,0.225);
#3527=FACE_OUTER_BOUND('',#5124,.T.);
#3528=FACE_OUTER_BOUND('',#5125,.T.);
#3529=FACE_OUTER_BOUND('',#5126,.T.);
#3530=FACE_OUTER_BOUND('',#5127,.T.);
#3531=FACE_OUTER_BOUND('',#5128,.T.);
#3532=FACE_OUTER_BOUND('',#5129,.T.);
#3533=FACE_OUTER_BOUND('',#5130,.T.);
#3534=FACE_OUTER_BOUND('',#5131,.T.);
#3535=FACE_OUTER_BOUND('',#5132,.T.);
#3536=FACE_OUTER_BOUND('',#5133,.T.);
#3537=FACE_OUTER_BOUND('',#5134,.T.);
#3538=FACE_OUTER_BOUND('',#5135,.T.);
#3539=FACE_OUTER_BOUND('',#5136,.T.);
#3540=FACE_OUTER_BOUND('',#5137,.T.);
#3541=FACE_OUTER_BOUND('',#5138,.T.);
#3542=FACE_OUTER_BOUND('',#5139,.T.);
#3543=FACE_OUTER_BOUND('',#5140,.T.);
#3544=FACE_OUTER_BOUND('',#5141,.T.);
#3545=FACE_OUTER_BOUND('',#5142,.T.);
#3546=FACE_OUTER_BOUND('',#5143,.T.);
#3547=FACE_OUTER_BOUND('',#5144,.T.);
#3548=FACE_OUTER_BOUND('',#5145,.T.);
#3549=FACE_OUTER_BOUND('',#5146,.T.);
#3550=FACE_OUTER_BOUND('',#5147,.T.);
#3551=FACE_OUTER_BOUND('',#5148,.T.);
#3552=FACE_OUTER_BOUND('',#5149,.T.);
#3553=FACE_OUTER_BOUND('',#5150,.T.);
#3554=FACE_OUTER_BOUND('',#5151,.T.);
#3555=FACE_OUTER_BOUND('',#5152,.T.);
#3556=FACE_OUTER_BOUND('',#5153,.T.);
#3557=FACE_OUTER_BOUND('',#5154,.T.);
#3558=FACE_OUTER_BOUND('',#5155,.T.);
#3559=FACE_OUTER_BOUND('',#5156,.T.);
#3560=FACE_OUTER_BOUND('',#5157,.T.);
#3561=FACE_OUTER_BOUND('',#5158,.T.);
#3562=FACE_OUTER_BOUND('',#5159,.T.);
#3563=FACE_OUTER_BOUND('',#5160,.T.);
#3564=FACE_OUTER_BOUND('',#5161,.T.);
#3565=FACE_OUTER_BOUND('',#5162,.T.);
#3566=FACE_OUTER_BOUND('',#5163,.T.);
#3567=FACE_OUTER_BOUND('',#5164,.T.);
#3568=FACE_OUTER_BOUND('',#5165,.T.);
#3569=FACE_OUTER_BOUND('',#5166,.T.);
#3570=FACE_OUTER_BOUND('',#5167,.T.);
#3571=FACE_OUTER_BOUND('',#5168,.T.);
#3572=FACE_OUTER_BOUND('',#5169,.T.);
#3573=FACE_OUTER_BOUND('',#5170,.T.);
#3574=FACE_OUTER_BOUND('',#5171,.T.);
#3575=FACE_OUTER_BOUND('',#5172,.T.);
#3576=FACE_OUTER_BOUND('',#5173,.T.);
#3577=FACE_OUTER_BOUND('',#5174,.T.);
#3578=FACE_OUTER_BOUND('',#5175,.T.);
#3579=FACE_OUTER_BOUND('',#5176,.T.);
#3580=FACE_OUTER_BOUND('',#5177,.T.);
#3581=FACE_OUTER_BOUND('',#5178,.T.);
#3582=FACE_OUTER_BOUND('',#5179,.T.);
#3583=FACE_OUTER_BOUND('',#5180,.T.);
#3584=FACE_OUTER_BOUND('',#5181,.T.);
#3585=FACE_OUTER_BOUND('',#5182,.T.);
#3586=FACE_OUTER_BOUND('',#5183,.T.);
#3587=FACE_OUTER_BOUND('',#5184,.T.);
#3588=FACE_OUTER_BOUND('',#5185,.T.);
#3589=FACE_OUTER_BOUND('',#5186,.T.);
#3590=FACE_OUTER_BOUND('',#5187,.T.);
#3591=FACE_OUTER_BOUND('',#5188,.T.);
#3592=FACE_OUTER_BOUND('',#5189,.T.);
#3593=FACE_OUTER_BOUND('',#5190,.T.);
#3594=FACE_OUTER_BOUND('',#5191,.T.);
#3595=FACE_OUTER_BOUND('',#5192,.T.);
#3596=FACE_OUTER_BOUND('',#5193,.T.);
#3597=FACE_OUTER_BOUND('',#5194,.T.);
#3598=FACE_OUTER_BOUND('',#5195,.T.);
#3599=FACE_OUTER_BOUND('',#5196,.T.);
#3600=FACE_OUTER_BOUND('',#5197,.T.);
#3601=FACE_OUTER_BOUND('',#5198,.T.);
#3602=FACE_OUTER_BOUND('',#5199,.T.);
#3603=FACE_OUTER_BOUND('',#5200,.T.);
#3604=FACE_OUTER_BOUND('',#5201,.T.);
#3605=FACE_OUTER_BOUND('',#5202,.T.);
#3606=FACE_OUTER_BOUND('',#5203,.T.);
#3607=FACE_OUTER_BOUND('',#5204,.T.);
#3608=FACE_OUTER_BOUND('',#5205,.T.);
#3609=FACE_OUTER_BOUND('',#5206,.T.);
#3610=FACE_OUTER_BOUND('',#5207,.T.);
#3611=FACE_OUTER_BOUND('',#5208,.T.);
#3612=FACE_OUTER_BOUND('',#5209,.T.);
#3613=FACE_OUTER_BOUND('',#5210,.T.);
#3614=FACE_OUTER_BOUND('',#5211,.T.);
#3615=FACE_OUTER_BOUND('',#5212,.T.);
#3616=FACE_OUTER_BOUND('',#5213,.T.);
#3617=FACE_OUTER_BOUND('',#5214,.T.);
#3618=FACE_OUTER_BOUND('',#5215,.T.);
#3619=FACE_OUTER_BOUND('',#5216,.T.);
#3620=FACE_OUTER_BOUND('',#5217,.T.);
#3621=FACE_OUTER_BOUND('',#5218,.T.);
#3622=FACE_OUTER_BOUND('',#5219,.T.);
#3623=FACE_OUTER_BOUND('',#5220,.T.);
#3624=FACE_OUTER_BOUND('',#5221,.T.);
#3625=FACE_OUTER_BOUND('',#5222,.T.);
#3626=FACE_OUTER_BOUND('',#5223,.T.);
#3627=FACE_OUTER_BOUND('',#5224,.T.);
#3628=FACE_OUTER_BOUND('',#5225,.T.);
#3629=FACE_OUTER_BOUND('',#5226,.T.);
#3630=FACE_OUTER_BOUND('',#5227,.T.);
#3631=FACE_OUTER_BOUND('',#5228,.T.);
#3632=FACE_OUTER_BOUND('',#5229,.T.);
#3633=FACE_OUTER_BOUND('',#5230,.T.);
#3634=FACE_OUTER_BOUND('',#5231,.T.);
#3635=FACE_OUTER_BOUND('',#5232,.T.);
#3636=FACE_OUTER_BOUND('',#5233,.T.);
#3637=FACE_OUTER_BOUND('',#5234,.T.);
#3638=FACE_OUTER_BOUND('',#5235,.T.);
#3639=FACE_OUTER_BOUND('',#5236,.T.);
#3640=FACE_OUTER_BOUND('',#5237,.T.);
#3641=FACE_OUTER_BOUND('',#5238,.T.);
#3642=FACE_OUTER_BOUND('',#5239,.T.);
#3643=FACE_OUTER_BOUND('',#5240,.T.);
#3644=FACE_OUTER_BOUND('',#5241,.T.);
#3645=FACE_OUTER_BOUND('',#5242,.T.);
#3646=FACE_OUTER_BOUND('',#5243,.T.);
#3647=FACE_OUTER_BOUND('',#5244,.T.);
#3648=FACE_OUTER_BOUND('',#5245,.T.);
#3649=FACE_OUTER_BOUND('',#5246,.T.);
#3650=FACE_OUTER_BOUND('',#5247,.T.);
#3651=FACE_OUTER_BOUND('',#5248,.T.);
#3652=FACE_OUTER_BOUND('',#5249,.T.);
#3653=FACE_OUTER_BOUND('',#5250,.T.);
#3654=FACE_OUTER_BOUND('',#5251,.T.);
#3655=FACE_OUTER_BOUND('',#5252,.T.);
#3656=FACE_OUTER_BOUND('',#5253,.T.);
#3657=FACE_OUTER_BOUND('',#5254,.T.);
#3658=FACE_OUTER_BOUND('',#5255,.T.);
#3659=FACE_OUTER_BOUND('',#5256,.T.);
#3660=FACE_OUTER_BOUND('',#5257,.T.);
#3661=FACE_OUTER_BOUND('',#5258,.T.);
#3662=FACE_OUTER_BOUND('',#5259,.T.);
#3663=FACE_OUTER_BOUND('',#5260,.T.);
#3664=FACE_OUTER_BOUND('',#5261,.T.);
#3665=FACE_OUTER_BOUND('',#5262,.T.);
#3666=FACE_OUTER_BOUND('',#5263,.T.);
#3667=FACE_OUTER_BOUND('',#5264,.T.);
#3668=FACE_OUTER_BOUND('',#5265,.T.);
#3669=FACE_OUTER_BOUND('',#5266,.T.);
#3670=FACE_OUTER_BOUND('',#5267,.T.);
#3671=FACE_OUTER_BOUND('',#5268,.T.);
#3672=FACE_OUTER_BOUND('',#5269,.T.);
#3673=FACE_OUTER_BOUND('',#5270,.T.);
#3674=FACE_OUTER_BOUND('',#5271,.T.);
#3675=FACE_OUTER_BOUND('',#5273,.T.);
#3676=FACE_OUTER_BOUND('',#5274,.T.);
#3677=FACE_OUTER_BOUND('',#5275,.T.);
#3678=FACE_OUTER_BOUND('',#5276,.T.);
#3679=FACE_OUTER_BOUND('',#5278,.T.);
#5124=EDGE_LOOP('',(#21552,#21553,#21554,#21555,#21556,#21557,#21558,#21559));
#5125=EDGE_LOOP('',(#21560,#21561,#21562,#21563));
#5126=EDGE_LOOP('',(#21564,#21565,#21566,#21567));
#5127=EDGE_LOOP('',(#21568,#21569,#21570,#21571));
#5128=EDGE_LOOP('',(#21572,#21573,#21574,#21575));
#5129=EDGE_LOOP('',(#21576,#21577,#21578,#21579));
#5130=EDGE_LOOP('',(#21580,#21581,#21582,#21583));
#5131=EDGE_LOOP('',(#21584,#21585,#21586,#21587));
#5132=EDGE_LOOP('',(#21588,#21589,#21590,#21591));
#5133=EDGE_LOOP('',(#21592,#21593,#21594,#21595));
#5134=EDGE_LOOP('',(#21596,#21597,#21598,#21599));
#5135=EDGE_LOOP('',(#21600,#21601,#21602,#21603));
#5136=EDGE_LOOP('',(#21604,#21605,#21606,#21607));
#5137=EDGE_LOOP('',(#21608,#21609,#21610,#21611));
#5138=EDGE_LOOP('',(#21612,#21613,#21614,#21615));
#5139=EDGE_LOOP('',(#21616,#21617,#21618,#21619));
#5140=EDGE_LOOP('',(#21620,#21621,#21622,#21623));
#5141=EDGE_LOOP('',(#21624,#21625,#21626,#21627));
#5142=EDGE_LOOP('',(#21628,#21629,#21630,#21631));
#5143=EDGE_LOOP('',(#21632,#21633,#21634,#21635));
#5144=EDGE_LOOP('',(#21636,#21637,#21638,#21639));
#5145=EDGE_LOOP('',(#21640,#21641,#21642,#21643));
#5146=EDGE_LOOP('',(#21644,#21645,#21646,#21647));
#5147=EDGE_LOOP('',(#21648,#21649,#21650,#21651,#21652));
#5148=EDGE_LOOP('',(#21653,#21654,#21655,#21656,#21657));
#5149=EDGE_LOOP('',(#21658,#21659,#21660,#21661,#21662,#21663,#21664,#21665,
#21666,#21667,#21668,#21669,#21670,#21671,#21672,#21673,#21674,#21675,#21676,
#21677,#21678,#21679,#21680,#21681,#21682,#21683,#21684,#21685));
#5150=EDGE_LOOP('',(#21686,#21687,#21688,#21689,#21690,#21691));
#5151=EDGE_LOOP('',(#21692,#21693,#21694));
#5152=EDGE_LOOP('',(#21695,#21696,#21697,#21698,#21699,#21700,#21701,#21702,
#21703,#21704,#21705,#21706,#21707,#21708,#21709,#21710,#21711,#21712,#21713,
#21714,#21715,#21716,#21717,#21718,#21719,#21720,#21721));
#5153=EDGE_LOOP('',(#21722,#21723,#21724,#21725));
#5154=EDGE_LOOP('',(#21726,#21727,#21728));
#5155=EDGE_LOOP('',(#21729,#21730,#21731,#21732));
#5156=EDGE_LOOP('',(#21733,#21734,#21735,#21736));
#5157=EDGE_LOOP('',(#21737,#21738,#21739));
#5158=EDGE_LOOP('',(#21740,#21741,#21742,#21743));
#5159=EDGE_LOOP('',(#21744,#21745,#21746,#21747));
#5160=EDGE_LOOP('',(#21748,#21749,#21750));
#5161=EDGE_LOOP('',(#21751,#21752,#21753,#21754));
#5162=EDGE_LOOP('',(#21755,#21756,#21757,#21758));
#5163=EDGE_LOOP('',(#21759,#21760,#21761));
#5164=EDGE_LOOP('',(#21762,#21763,#21764,#21765));
#5165=EDGE_LOOP('',(#21766,#21767,#21768,#21769));
#5166=EDGE_LOOP('',(#21770,#21771,#21772));
#5167=EDGE_LOOP('',(#21773,#21774,#21775,#21776));
#5168=EDGE_LOOP('',(#21777,#21778,#21779,#21780));
#5169=EDGE_LOOP('',(#21781,#21782,#21783));
#5170=EDGE_LOOP('',(#21784,#21785,#21786,#21787));
#5171=EDGE_LOOP('',(#21788,#21789,#21790,#21791));
#5172=EDGE_LOOP('',(#21792,#21793,#21794));
#5173=EDGE_LOOP('',(#21795,#21796,#21797,#21798));
#5174=EDGE_LOOP('',(#21799,#21800,#21801,#21802));
#5175=EDGE_LOOP('',(#21803,#21804,#21805));
#5176=EDGE_LOOP('',(#21806,#21807,#21808,#21809));
#5177=EDGE_LOOP('',(#21810,#21811,#21812,#21813));
#5178=EDGE_LOOP('',(#21814,#21815,#21816));
#5179=EDGE_LOOP('',(#21817,#21818,#21819,#21820));
#5180=EDGE_LOOP('',(#21821,#21822,#21823,#21824));
#5181=EDGE_LOOP('',(#21825,#21826,#21827));
#5182=EDGE_LOOP('',(#21828,#21829,#21830,#21831));
#5183=EDGE_LOOP('',(#21832,#21833,#21834,#21835));
#5184=EDGE_LOOP('',(#21836,#21837,#21838));
#5185=EDGE_LOOP('',(#21839,#21840,#21841,#21842));
#5186=EDGE_LOOP('',(#21843,#21844,#21845,#21846));
#5187=EDGE_LOOP('',(#21847,#21848,#21849));
#5188=EDGE_LOOP('',(#21850,#21851,#21852,#21853));
#5189=EDGE_LOOP('',(#21854,#21855,#21856,#21857));
#5190=EDGE_LOOP('',(#21858,#21859,#21860));
#5191=EDGE_LOOP('',(#21861,#21862,#21863,#21864));
#5192=EDGE_LOOP('',(#21865,#21866,#21867,#21868));
#5193=EDGE_LOOP('',(#21869,#21870,#21871));
#5194=EDGE_LOOP('',(#21872,#21873,#21874,#21875));
#5195=EDGE_LOOP('',(#21876,#21877,#21878,#21879));
#5196=EDGE_LOOP('',(#21880,#21881,#21882));
#5197=EDGE_LOOP('',(#21883,#21884,#21885,#21886));
#5198=EDGE_LOOP('',(#21887,#21888,#21889,#21890));
#5199=EDGE_LOOP('',(#21891,#21892,#21893));
#5200=EDGE_LOOP('',(#21894,#21895,#21896,#21897));
#5201=EDGE_LOOP('',(#21898,#21899,#21900,#21901));
#5202=EDGE_LOOP('',(#21902,#21903,#21904));
#5203=EDGE_LOOP('',(#21905,#21906,#21907,#21908));
#5204=EDGE_LOOP('',(#21909,#21910,#21911,#21912));
#5205=EDGE_LOOP('',(#21913,#21914,#21915,#21916));
#5206=EDGE_LOOP('',(#21917,#21918,#21919,#21920));
#5207=EDGE_LOOP('',(#21921,#21922,#21923,#21924));
#5208=EDGE_LOOP('',(#21925,#21926,#21927));
#5209=EDGE_LOOP('',(#21928,#21929,#21930,#21931));
#5210=EDGE_LOOP('',(#21932,#21933,#21934,#21935));
#5211=EDGE_LOOP('',(#21936,#21937,#21938));
#5212=EDGE_LOOP('',(#21939,#21940,#21941,#21942));
#5213=EDGE_LOOP('',(#21943,#21944,#21945,#21946));
#5214=EDGE_LOOP('',(#21947,#21948,#21949));
#5215=EDGE_LOOP('',(#21950,#21951,#21952,#21953));
#5216=EDGE_LOOP('',(#21954,#21955,#21956,#21957));
#5217=EDGE_LOOP('',(#21958,#21959,#21960));
#5218=EDGE_LOOP('',(#21961,#21962,#21963,#21964));
#5219=EDGE_LOOP('',(#21965,#21966,#21967,#21968));
#5220=EDGE_LOOP('',(#21969,#21970,#21971));
#5221=EDGE_LOOP('',(#21972,#21973,#21974,#21975));
#5222=EDGE_LOOP('',(#21976,#21977,#21978,#21979));
#5223=EDGE_LOOP('',(#21980,#21981,#21982));
#5224=EDGE_LOOP('',(#21983,#21984,#21985,#21986));
#5225=EDGE_LOOP('',(#21987,#21988,#21989,#21990));
#5226=EDGE_LOOP('',(#21991,#21992,#21993));
#5227=EDGE_LOOP('',(#21994,#21995,#21996,#21997));
#5228=EDGE_LOOP('',(#21998,#21999,#22000,#22001));
#5229=EDGE_LOOP('',(#22002,#22003,#22004));
#5230=EDGE_LOOP('',(#22005,#22006,#22007,#22008));
#5231=EDGE_LOOP('',(#22009,#22010,#22011,#22012));
#5232=EDGE_LOOP('',(#22013,#22014,#22015));
#5233=EDGE_LOOP('',(#22016,#22017,#22018,#22019));
#5234=EDGE_LOOP('',(#22020,#22021,#22022,#22023));
#5235=EDGE_LOOP('',(#22024,#22025,#22026));
#5236=EDGE_LOOP('',(#22027,#22028,#22029,#22030));
#5237=EDGE_LOOP('',(#22031,#22032,#22033,#22034));
#5238=EDGE_LOOP('',(#22035,#22036,#22037));
#5239=EDGE_LOOP('',(#22038,#22039,#22040,#22041));
#5240=EDGE_LOOP('',(#22042,#22043,#22044,#22045));
#5241=EDGE_LOOP('',(#22046,#22047,#22048));
#5242=EDGE_LOOP('',(#22049,#22050,#22051,#22052));
#5243=EDGE_LOOP('',(#22053,#22054,#22055,#22056));
#5244=EDGE_LOOP('',(#22057,#22058,#22059));
#5245=EDGE_LOOP('',(#22060,#22061,#22062,#22063));
#5246=EDGE_LOOP('',(#22064,#22065,#22066,#22067));
#5247=EDGE_LOOP('',(#22068,#22069,#22070));
#5248=EDGE_LOOP('',(#22071,#22072,#22073,#22074));
#5249=EDGE_LOOP('',(#22075,#22076,#22077,#22078));
#5250=EDGE_LOOP('',(#22079,#22080,#22081));
#5251=EDGE_LOOP('',(#22082,#22083,#22084,#22085));
#5252=EDGE_LOOP('',(#22086,#22087,#22088,#22089));
#5253=EDGE_LOOP('',(#22090,#22091,#22092));
#5254=EDGE_LOOP('',(#22093,#22094,#22095,#22096));
#5255=EDGE_LOOP('',(#22097,#22098,#22099,#22100));
#5256=EDGE_LOOP('',(#22101,#22102,#22103));
#5257=EDGE_LOOP('',(#22104,#22105,#22106,#22107));
#5258=EDGE_LOOP('',(#22108,#22109,#22110,#22111));
#5259=EDGE_LOOP('',(#22112,#22113,#22114,#22115,#22116,#22117,#22118,#22119,
#22120,#22121,#22122,#22123,#22124,#22125,#22126,#22127,#22128,#22129,#22130,
#22131,#22132,#22133,#22134,#22135,#22136,#22137,#22138,#22139,#22140,#22141,
#22142,#22143,#22144,#22145,#22146,#22147,#22148,#22149,#22150,#22151,#22152,
#22153,#22154,#22155,#22156,#22157,#22158,#22159,#22160,#22161,#22162,#22163,
#22164,#22165,#22166,#22167,#22168,#22169,#22170,#22171,#22172,#22173,#22174,
#22175,#22176,#22177,#22178,#22179,#22180,#22181,#22182,#22183,#22184,#22185,
#22186,#22187,#22188,#22189,#22190,#22191,#22192,#22193,#22194,#22195,#22196,
#22197,#22198,#22199,#22200,#22201,#22202,#22203,#22204,#22205,#22206,#22207,
#22208,#22209,#22210,#22211,#22212,#22213,#22214,#22215,#22216,#22217,#22218,
#22219,#22220,#22221,#22222,#22223,#22224,#22225,#22226,#22227,#22228,#22229,
#22230,#22231,#22232,#22233,#22234,#22235,#22236,#22237,#22238,#22239,#22240,
#22241,#22242,#22243,#22244,#22245,#22246,#22247,#22248,#22249,#22250,#22251,
#22252,#22253,#22254,#22255,#22256,#22257,#22258,#22259));
#5260=EDGE_LOOP('',(#22260,#22261,#22262,#22263));
#5261=EDGE_LOOP('',(#22264,#22265,#22266,#22267));
#5262=EDGE_LOOP('',(#22268,#22269,#22270));
#5263=EDGE_LOOP('',(#22271,#22272,#22273,#22274,#22275,#22276,#22277,#22278,
#22279,#22280,#22281,#22282,#22283,#22284,#22285,#22286,#22287,#22288,#22289,
#22290,#22291,#22292,#22293,#22294,#22295,#22296,#22297,#22298,#22299,#22300,
#22301,#22302,#22303,#22304,#22305,#22306,#22307,#22308,#22309,#22310,#22311,
#22312,#22313,#22314,#22315,#22316,#22317,#22318,#22319,#22320,#22321,#22322,
#22323,#22324,#22325,#22326,#22327,#22328,#22329,#22330,#22331,#22332,#22333,
#22334,#22335,#22336,#22337,#22338,#22339,#22340,#22341,#22342,#22343,#22344,
#22345,#22346,#22347,#22348,#22349,#22350,#22351,#22352,#22353,#22354,#22355,
#22356,#22357,#22358,#22359,#22360,#22361,#22362,#22363,#22364,#22365,#22366,
#22367,#22368,#22369,#22370,#22371,#22372,#22373,#22374,#22375,#22376,#22377,
#22378,#22379,#22380,#22381));
#5264=EDGE_LOOP('',(#22382,#22383,#22384));
#5265=EDGE_LOOP('',(#22385,#22386,#22387,#22388));
#5266=EDGE_LOOP('',(#22389,#22390,#22391,#22392));
#5267=EDGE_LOOP('',(#22393,#22394,#22395,#22396));
#5268=EDGE_LOOP('',(#22397,#22398,#22399,#22400));
#5269=EDGE_LOOP('',(#22401,#22402,#22403,#22404));
#5270=EDGE_LOOP('',(#22405,#22406,#22407,#22408));
#5271=EDGE_LOOP('',(#22409,#22410,#22411,#22412,#22413,#22414));
#5272=EDGE_LOOP('',(#22415));
#5273=EDGE_LOOP('',(#22416));
#5274=EDGE_LOOP('',(#22417,#22418,#22419,#22420));
#5275=EDGE_LOOP('',(#22421,#22422,#22423,#22424,#22425,#22426));
#5276=EDGE_LOOP('',(#22427));
#5277=EDGE_LOOP('',(#22428));
#5278=EDGE_LOOP('',(#22429));
#5279=EDGE_LOOP('',(#22430,#22431,#22432,#22433,#22434,#22435));
#6845=LINE('',#48673,#8666);
#6846=LINE('',#48694,#8667);
#6847=LINE('',#48714,#8668);
#6848=LINE('',#48762,#8669);
#6849=LINE('',#48810,#8670);
#6850=LINE('',#48864,#8671);
#6851=LINE('',#48912,#8672);
#6852=LINE('',#48966,#8673);
#6853=LINE('',#49014,#8674);
#6854=LINE('',#49062,#8675);
#6855=LINE('',#49116,#8676);
#6856=LINE('',#49164,#8677);
#6857=LINE('',#49212,#8678);
#6858=LINE('',#49266,#8679);
#6859=LINE('',#49289,#8680);
#6860=LINE('',#49314,#8681);
#6861=LINE('',#49338,#8682);
#6862=LINE('',#49363,#8683);
#6863=LINE('',#49388,#8684);
#6864=LINE('',#49412,#8685);
#6865=LINE('',#49437,#8686);
#6866=LINE('',#49462,#8687);
#6867=LINE('',#49487,#8688);
#6868=LINE('',#49512,#8689);
#6869=LINE('',#49536,#8690);
#6870=LINE('',#50428,#8691);
#6871=LINE('',#50429,#8692);
#6872=LINE('',#50432,#8693);
#6873=LINE('',#50434,#8694);
#6874=LINE('',#50440,#8695);
#6875=LINE('',#50449,#8696);
#6876=LINE('',#50450,#8697);
#6877=LINE('',#50453,#8698);
#6878=LINE('',#50455,#8699);
#6879=LINE('',#50461,#8700);
#6880=LINE('',#50470,#8701);
#6881=LINE('',#50471,#8702);
#6882=LINE('',#50474,#8703);
#6883=LINE('',#50476,#8704);
#6884=LINE('',#50482,#8705);
#6885=LINE('',#50491,#8706);
#6886=LINE('',#50492,#8707);
#6887=LINE('',#50495,#8708);
#6888=LINE('',#50497,#8709);
#6889=LINE('',#50503,#8710);
#6890=LINE('',#50512,#8711);
#6891=LINE('',#50513,#8712);
#6892=LINE('',#50516,#8713);
#6893=LINE('',#50518,#8714);
#6894=LINE('',#50524,#8715);
#6895=LINE('',#50533,#8716);
#6896=LINE('',#50534,#8717);
#6897=LINE('',#50537,#8718);
#6898=LINE('',#50539,#8719);
#6899=LINE('',#50545,#8720);
#6900=LINE('',#50554,#8721);
#6901=LINE('',#50555,#8722);
#6902=LINE('',#50558,#8723);
#6903=LINE('',#50560,#8724);
#6904=LINE('',#50566,#8725);
#6905=LINE('',#50575,#8726);
#6906=LINE('',#50576,#8727);
#6907=LINE('',#50579,#8728);
#6908=LINE('',#50581,#8729);
#6909=LINE('',#50587,#8730);
#6910=LINE('',#50596,#8731);
#6911=LINE('',#50597,#8732);
#6912=LINE('',#50600,#8733);
#6913=LINE('',#50602,#8734);
#6914=LINE('',#50608,#8735);
#6915=LINE('',#50617,#8736);
#6916=LINE('',#50618,#8737);
#6917=LINE('',#50621,#8738);
#6918=LINE('',#50623,#8739);
#6919=LINE('',#50629,#8740);
#6920=LINE('',#50638,#8741);
#6921=LINE('',#50639,#8742);
#6922=LINE('',#50642,#8743);
#6923=LINE('',#50644,#8744);
#6924=LINE('',#50650,#8745);
#6925=LINE('',#50659,#8746);
#6926=LINE('',#50660,#8747);
#6927=LINE('',#50663,#8748);
#6928=LINE('',#50665,#8749);
#6929=LINE('',#50671,#8750);
#6930=LINE('',#50680,#8751);
#6931=LINE('',#50681,#8752);
#6932=LINE('',#50684,#8753);
#6933=LINE('',#50686,#8754);
#6934=LINE('',#50692,#8755);
#6935=LINE('',#50701,#8756);
#6936=LINE('',#50702,#8757);
#6937=LINE('',#50705,#8758);
#6938=LINE('',#50707,#8759);
#6939=LINE('',#50713,#8760);
#6940=LINE('',#50722,#8761);
#6941=LINE('',#50723,#8762);
#6942=LINE('',#50726,#8763);
#6943=LINE('',#50728,#8764);
#6944=LINE('',#50734,#8765);
#6945=LINE('',#50743,#8766);
#6946=LINE('',#50744,#8767);
#6947=LINE('',#50747,#8768);
#6948=LINE('',#50749,#8769);
#6949=LINE('',#50755,#8770);
#6950=LINE('',#50764,#8771);
#6951=LINE('',#50765,#8772);
#6952=LINE('',#50768,#8773);
#6953=LINE('',#50770,#8774);
#6954=LINE('',#50776,#8775);
#6955=LINE('',#50785,#8776);
#6956=LINE('',#50787,#8777);
#6957=LINE('',#50791,#8778);
#6958=LINE('',#50793,#8779);
#6959=LINE('',#50799,#8780);
#6960=LINE('',#50808,#8781);
#6961=LINE('',#50809,#8782);
#6962=LINE('',#50812,#8783);
#6963=LINE('',#50814,#8784);
#6964=LINE('',#50820,#8785);
#6965=LINE('',#50829,#8786);
#6966=LINE('',#50830,#8787);
#6967=LINE('',#50833,#8788);
#6968=LINE('',#50835,#8789);
#6969=LINE('',#50841,#8790);
#6970=LINE('',#50850,#8791);
#6971=LINE('',#50851,#8792);
#6972=LINE('',#50854,#8793);
#6973=LINE('',#50856,#8794);
#6974=LINE('',#50862,#8795);
#6975=LINE('',#50871,#8796);
#6976=LINE('',#50872,#8797);
#6977=LINE('',#50875,#8798);
#6978=LINE('',#50877,#8799);
#6979=LINE('',#50883,#8800);
#6980=LINE('',#50892,#8801);
#6981=LINE('',#50893,#8802);
#6982=LINE('',#50896,#8803);
#6983=LINE('',#50898,#8804);
#6984=LINE('',#50904,#8805);
#6985=LINE('',#50913,#8806);
#6986=LINE('',#50914,#8807);
#6987=LINE('',#50917,#8808);
#6988=LINE('',#50919,#8809);
#6989=LINE('',#50925,#8810);
#6990=LINE('',#50934,#8811);
#6991=LINE('',#50935,#8812);
#6992=LINE('',#50938,#8813);
#6993=LINE('',#50940,#8814);
#6994=LINE('',#50946,#8815);
#6995=LINE('',#50955,#8816);
#6996=LINE('',#50956,#8817);
#6997=LINE('',#50959,#8818);
#6998=LINE('',#50961,#8819);
#6999=LINE('',#50967,#8820);
#7000=LINE('',#50976,#8821);
#7001=LINE('',#50977,#8822);
#7002=LINE('',#50980,#8823);
#7003=LINE('',#50982,#8824);
#7004=LINE('',#50988,#8825);
#7005=LINE('',#50997,#8826);
#7006=LINE('',#50998,#8827);
#7007=LINE('',#51001,#8828);
#7008=LINE('',#51003,#8829);
#7009=LINE('',#51009,#8830);
#7010=LINE('',#51018,#8831);
#7011=LINE('',#51019,#8832);
#7012=LINE('',#51022,#8833);
#7013=LINE('',#51024,#8834);
#7014=LINE('',#51030,#8835);
#7015=LINE('',#51039,#8836);
#7016=LINE('',#51040,#8837);
#7017=LINE('',#51043,#8838);
#7018=LINE('',#51045,#8839);
#7019=LINE('',#51051,#8840);
#7020=LINE('',#51060,#8841);
#7021=LINE('',#51061,#8842);
#7022=LINE('',#51064,#8843);
#7023=LINE('',#51066,#8844);
#7024=LINE('',#51072,#8845);
#7025=LINE('',#51081,#8846);
#7026=LINE('',#51082,#8847);
#7027=LINE('',#51085,#8848);
#7028=LINE('',#51087,#8849);
#7029=LINE('',#51093,#8850);
#7030=LINE('',#51102,#8851);
#7031=LINE('',#51103,#8852);
#7032=LINE('',#51106,#8853);
#7033=LINE('',#51108,#8854);
#7034=LINE('',#51114,#8855);
#7035=LINE('',#51123,#8856);
#7036=LINE('',#51124,#8857);
#7037=LINE('',#51127,#8858);
#7038=LINE('',#51129,#8859);
#7039=LINE('',#51135,#8860);
#7040=LINE('',#51144,#8861);
#7041=LINE('',#51145,#8862);
#7042=LINE('',#51148,#8863);
#7043=LINE('',#51150,#8864);
#7044=LINE('',#51156,#8865);
#7045=LINE('',#51179,#8866);
#7046=LINE('',#51201,#8867);
#7047=LINE('',#51205,#8868);
#7048=LINE('',#51209,#8869);
#7049=LINE('',#51211,#8870);
#7050=LINE('',#51219,#8871);
#7051=LINE('',#51224,#8872);
#7052=LINE('',#51228,#8873);
#7053=LINE('',#51233,#8874);
#7054=LINE('',#51235,#8875);
#7055=LINE('',#51237,#8876);
#7056=LINE('',#51238,#8877);
#7057=LINE('',#51241,#8878);
#7058=LINE('',#51243,#8879);
#7059=LINE('',#51244,#8880);
#7060=LINE('',#51247,#8881);
#7061=LINE('',#51249,#8882);
#7062=LINE('',#51250,#8883);
#7063=LINE('',#51253,#8884);
#7064=LINE('',#51255,#8885);
#7065=LINE('',#51256,#8886);
#7066=LINE('',#51259,#8887);
#7067=LINE('',#51261,#8888);
#7068=LINE('',#51262,#8889);
#7069=LINE('',#51264,#8890);
#7070=LINE('',#51265,#8891);
#7071=LINE('',#51271,#8892);
#7072=LINE('',#51275,#8893);
#8666=VECTOR('',#32697,0.125);
#8667=VECTOR('',#32700,0.125);
#8668=VECTOR('',#32707,0.125);
#8669=VECTOR('',#32710,0.125);
#8670=VECTOR('',#32713,0.125);
#8671=VECTOR('',#32716,0.125);
#8672=VECTOR('',#32719,0.125);
#8673=VECTOR('',#32722,0.125);
#8674=VECTOR('',#32725,0.125);
#8675=VECTOR('',#32728,0.125);
#8676=VECTOR('',#32731,0.125);
#8677=VECTOR('',#32734,0.125);
#8678=VECTOR('',#32737,0.125);
#8679=VECTOR('',#32740,0.095825);
#8680=VECTOR('',#32745,0.095825);
#8681=VECTOR('',#32748,0.095825);
#8682=VECTOR('',#32751,0.095825);
#8683=VECTOR('',#32754,0.095825);
#8684=VECTOR('',#32757,0.095825);
#8685=VECTOR('',#32760,0.095825);
#8686=VECTOR('',#32763,0.095825);
#8687=VECTOR('',#32766,0.095825);
#8688=VECTOR('',#32769,0.095825);
#8689=VECTOR('',#32772,0.095825);
#8690=VECTOR('',#32775,0.095825);
#8691=VECTOR('',#32798,1.);
#8692=VECTOR('',#32799,1.);
#8693=VECTOR('',#32802,1.);
#8694=VECTOR('',#32803,1.);
#8695=VECTOR('',#32806,1.);
#8696=VECTOR('',#32811,1.);
#8697=VECTOR('',#32812,1.);
#8698=VECTOR('',#32815,1.);
#8699=VECTOR('',#32816,1.);
#8700=VECTOR('',#32819,1.);
#8701=VECTOR('',#32824,1.);
#8702=VECTOR('',#32825,1.);
#8703=VECTOR('',#32828,1.);
#8704=VECTOR('',#32829,1.);
#8705=VECTOR('',#32832,1.);
#8706=VECTOR('',#32837,1.);
#8707=VECTOR('',#32838,1.);
#8708=VECTOR('',#32841,1.);
#8709=VECTOR('',#32842,1.);
#8710=VECTOR('',#32845,1.);
#8711=VECTOR('',#32850,1.);
#8712=VECTOR('',#32851,1.);
#8713=VECTOR('',#32854,1.);
#8714=VECTOR('',#32855,1.);
#8715=VECTOR('',#32858,1.);
#8716=VECTOR('',#32863,1.);
#8717=VECTOR('',#32864,1.);
#8718=VECTOR('',#32867,1.);
#8719=VECTOR('',#32868,1.);
#8720=VECTOR('',#32871,1.);
#8721=VECTOR('',#32876,1.);
#8722=VECTOR('',#32877,1.);
#8723=VECTOR('',#32880,1.);
#8724=VECTOR('',#32881,1.);
#8725=VECTOR('',#32884,1.);
#8726=VECTOR('',#32889,1.);
#8727=VECTOR('',#32890,1.);
#8728=VECTOR('',#32893,1.);
#8729=VECTOR('',#32894,1.);
#8730=VECTOR('',#32897,1.);
#8731=VECTOR('',#32902,1.);
#8732=VECTOR('',#32903,1.);
#8733=VECTOR('',#32906,1.);
#8734=VECTOR('',#32907,1.);
#8735=VECTOR('',#32910,1.);
#8736=VECTOR('',#32915,1.);
#8737=VECTOR('',#32916,1.);
#8738=VECTOR('',#32919,1.);
#8739=VECTOR('',#32920,1.);
#8740=VECTOR('',#32923,1.);
#8741=VECTOR('',#32928,1.);
#8742=VECTOR('',#32929,1.);
#8743=VECTOR('',#32932,1.);
#8744=VECTOR('',#32933,1.);
#8745=VECTOR('',#32936,1.);
#8746=VECTOR('',#32941,1.);
#8747=VECTOR('',#32942,1.);
#8748=VECTOR('',#32945,1.);
#8749=VECTOR('',#32946,1.);
#8750=VECTOR('',#32949,1.);
#8751=VECTOR('',#32954,1.);
#8752=VECTOR('',#32955,1.);
#8753=VECTOR('',#32958,1.);
#8754=VECTOR('',#32959,1.);
#8755=VECTOR('',#32962,1.);
#8756=VECTOR('',#32967,1.);
#8757=VECTOR('',#32968,1.);
#8758=VECTOR('',#32971,1.);
#8759=VECTOR('',#32972,1.);
#8760=VECTOR('',#32975,1.);
#8761=VECTOR('',#32980,1.);
#8762=VECTOR('',#32981,1.);
#8763=VECTOR('',#32984,1.);
#8764=VECTOR('',#32985,1.);
#8765=VECTOR('',#32988,1.);
#8766=VECTOR('',#32993,1.);
#8767=VECTOR('',#32994,1.);
#8768=VECTOR('',#32997,1.);
#8769=VECTOR('',#32998,1.);
#8770=VECTOR('',#33001,1.);
#8771=VECTOR('',#33006,1.);
#8772=VECTOR('',#33007,1.);
#8773=VECTOR('',#33010,1.);
#8774=VECTOR('',#33011,1.);
#8775=VECTOR('',#33014,1.);
#8776=VECTOR('',#33019,1.);
#8777=VECTOR('',#33020,1.);
#8778=VECTOR('',#33025,1.);
#8779=VECTOR('',#33026,1.);
#8780=VECTOR('',#33029,1.);
#8781=VECTOR('',#33034,1.);
#8782=VECTOR('',#33035,1.);
#8783=VECTOR('',#33038,1.);
#8784=VECTOR('',#33039,1.);
#8785=VECTOR('',#33042,1.);
#8786=VECTOR('',#33047,1.);
#8787=VECTOR('',#33048,1.);
#8788=VECTOR('',#33051,1.);
#8789=VECTOR('',#33052,1.);
#8790=VECTOR('',#33055,1.);
#8791=VECTOR('',#33060,1.);
#8792=VECTOR('',#33061,1.);
#8793=VECTOR('',#33064,1.);
#8794=VECTOR('',#33065,1.);
#8795=VECTOR('',#33068,1.);
#8796=VECTOR('',#33073,1.);
#8797=VECTOR('',#33074,1.);
#8798=VECTOR('',#33077,1.);
#8799=VECTOR('',#33078,1.);
#8800=VECTOR('',#33081,1.);
#8801=VECTOR('',#33086,1.);
#8802=VECTOR('',#33087,1.);
#8803=VECTOR('',#33090,1.);
#8804=VECTOR('',#33091,1.);
#8805=VECTOR('',#33094,1.);
#8806=VECTOR('',#33099,1.);
#8807=VECTOR('',#33100,1.);
#8808=VECTOR('',#33103,1.);
#8809=VECTOR('',#33104,1.);
#8810=VECTOR('',#33107,1.);
#8811=VECTOR('',#33112,1.);
#8812=VECTOR('',#33113,1.);
#8813=VECTOR('',#33116,1.);
#8814=VECTOR('',#33117,1.);
#8815=VECTOR('',#33120,1.);
#8816=VECTOR('',#33125,1.);
#8817=VECTOR('',#33126,1.);
#8818=VECTOR('',#33129,1.);
#8819=VECTOR('',#33130,1.);
#8820=VECTOR('',#33133,1.);
#8821=VECTOR('',#33138,1.);
#8822=VECTOR('',#33139,1.);
#8823=VECTOR('',#33142,1.);
#8824=VECTOR('',#33143,1.);
#8825=VECTOR('',#33146,1.);
#8826=VECTOR('',#33151,1.);
#8827=VECTOR('',#33152,1.);
#8828=VECTOR('',#33155,1.);
#8829=VECTOR('',#33156,1.);
#8830=VECTOR('',#33159,1.);
#8831=VECTOR('',#33164,1.);
#8832=VECTOR('',#33165,1.);
#8833=VECTOR('',#33168,1.);
#8834=VECTOR('',#33169,1.);
#8835=VECTOR('',#33172,1.);
#8836=VECTOR('',#33177,1.);
#8837=VECTOR('',#33178,1.);
#8838=VECTOR('',#33181,1.);
#8839=VECTOR('',#33182,1.);
#8840=VECTOR('',#33185,1.);
#8841=VECTOR('',#33190,1.);
#8842=VECTOR('',#33191,1.);
#8843=VECTOR('',#33194,1.);
#8844=VECTOR('',#33195,1.);
#8845=VECTOR('',#33198,1.);
#8846=VECTOR('',#33203,1.);
#8847=VECTOR('',#33204,1.);
#8848=VECTOR('',#33207,1.);
#8849=VECTOR('',#33208,1.);
#8850=VECTOR('',#33211,1.);
#8851=VECTOR('',#33216,1.);
#8852=VECTOR('',#33217,1.);
#8853=VECTOR('',#33220,1.);
#8854=VECTOR('',#33221,1.);
#8855=VECTOR('',#33224,1.);
#8856=VECTOR('',#33229,1.);
#8857=VECTOR('',#33230,1.);
#8858=VECTOR('',#33233,1.);
#8859=VECTOR('',#33234,1.);
#8860=VECTOR('',#33237,1.);
#8861=VECTOR('',#33242,1.);
#8862=VECTOR('',#33243,1.);
#8863=VECTOR('',#33246,1.);
#8864=VECTOR('',#33247,1.);
#8865=VECTOR('',#33250,1.);
#8866=VECTOR('',#33287,0.225);
#8867=VECTOR('',#33326,1.);
#8868=VECTOR('',#33329,1.);
#8869=VECTOR('',#33334,1.);
#8870=VECTOR('',#33335,1.);
#8871=VECTOR('',#33338,1.);
#8872=VECTOR('',#33345,0.2175);
#8873=VECTOR('',#33348,0.0461880215351701);
#8874=VECTOR('',#33353,1.);
#8875=VECTOR('',#33354,1.);
#8876=VECTOR('',#33355,1.);
#8877=VECTOR('',#33356,1.);
#8878=VECTOR('',#33359,1.);
#8879=VECTOR('',#33360,1.);
#8880=VECTOR('',#33361,1.);
#8881=VECTOR('',#33364,1.);
#8882=VECTOR('',#33365,1.);
#8883=VECTOR('',#33366,1.);
#8884=VECTOR('',#33369,1.);
#8885=VECTOR('',#33370,1.);
#8886=VECTOR('',#33371,1.);
#8887=VECTOR('',#33374,1.);
#8888=VECTOR('',#33375,1.);
#8889=VECTOR('',#33376,1.);
#8890=VECTOR('',#33379,1.);
#8891=VECTOR('',#33380,1.);
#8892=VECTOR('',#33389,0.11);
#8893=VECTOR('',#33394,0.13);
#9916=CIRCLE('',#26788,0.1215);
#9917=CIRCLE('',#26789,0.1215);
#9918=CIRCLE('',#26790,0.1215);
#9919=CIRCLE('',#26803,0.095825);
#9920=CIRCLE('',#26815,0.095825);
#9921=CIRCLE('',#26817,0.1215);
#9922=CIRCLE('',#26818,0.1215);
#9923=CIRCLE('',#26820,0.095825);
#9924=CIRCLE('',#26823,0.1215);
#9925=CIRCLE('',#26825,0.225);
#9926=CIRCLE('',#26829,0.225);
#9927=CIRCLE('',#26833,0.225);
#9928=CIRCLE('',#26837,0.225);
#9929=CIRCLE('',#26841,0.225);
#9930=CIRCLE('',#26845,0.225);
#9931=CIRCLE('',#26849,0.225);
#9932=CIRCLE('',#26853,0.225);
#9933=CIRCLE('',#26857,0.225);
#9934=CIRCLE('',#26861,0.225);
#9935=CIRCLE('',#26865,0.225);
#9936=CIRCLE('',#26869,0.225);
#9937=CIRCLE('',#26873,0.225);
#9938=CIRCLE('',#26877,0.225);
#9939=CIRCLE('',#26881,0.225);
#9940=CIRCLE('',#26885,0.225);
#9941=CIRCLE('',#26889,0.225);
#9942=CIRCLE('',#26893,0.225);
#9943=CIRCLE('',#26894,0.225);
#9944=CIRCLE('',#26898,0.225);
#9945=CIRCLE('',#26902,0.225);
#9946=CIRCLE('',#26906,0.225);
#9947=CIRCLE('',#26910,0.225);
#9948=CIRCLE('',#26914,0.225);
#9949=CIRCLE('',#26918,0.225);
#9950=CIRCLE('',#26922,0.225);
#9951=CIRCLE('',#26926,0.225);
#9952=CIRCLE('',#26930,0.225);
#9953=CIRCLE('',#26934,0.225);
#9954=CIRCLE('',#26938,0.225);
#9955=CIRCLE('',#26942,0.225);
#9956=CIRCLE('',#26946,0.225);
#9957=CIRCLE('',#26950,0.225);
#9958=CIRCLE('',#26954,0.225);
#9959=CIRCLE('',#26958,0.225);
#9960=CIRCLE('',#26962,0.225);
#9961=CIRCLE('',#26966,0.225);
#9962=CIRCLE('',#26967,0.225);
#9963=CIRCLE('',#26968,0.225);
#9964=CIRCLE('',#26969,0.225);
#9965=CIRCLE('',#26970,0.225);
#9966=CIRCLE('',#26971,0.225);
#9967=CIRCLE('',#26972,0.225);
#9968=CIRCLE('',#26973,0.225);
#9969=CIRCLE('',#26974,0.225);
#9970=CIRCLE('',#26975,0.225);
#9971=CIRCLE('',#26976,0.225);
#9972=CIRCLE('',#26977,0.225);
#9973=CIRCLE('',#26978,0.225);
#9974=CIRCLE('',#26979,0.225);
#9975=CIRCLE('',#26980,0.225);
#9976=CIRCLE('',#26981,0.225);
#9977=CIRCLE('',#26982,0.225);
#9978=CIRCLE('',#26983,0.225);
#9979=CIRCLE('',#26984,0.225);
#9980=CIRCLE('',#26985,0.225);
#9981=CIRCLE('',#26986,0.225);
#9982=CIRCLE('',#26987,0.225);
#9983=CIRCLE('',#26988,0.225);
#9984=CIRCLE('',#26989,0.225);
#9985=CIRCLE('',#26990,0.225);
#9986=CIRCLE('',#26991,0.225);
#9987=CIRCLE('',#26992,0.225);
#9988=CIRCLE('',#26993,0.225);
#9989=CIRCLE('',#26994,0.225);
#9990=CIRCLE('',#26995,0.225);
#9991=CIRCLE('',#26996,0.225);
#9992=CIRCLE('',#26997,0.225);
#9993=CIRCLE('',#26998,0.225);
#9994=CIRCLE('',#26999,0.225);
#9995=CIRCLE('',#27000,0.225);
#9996=CIRCLE('',#27001,0.225);
#9997=CIRCLE('',#27002,0.225);
#9998=CIRCLE('',#27003,0.225);
#9999=CIRCLE('',#27008,0.21);
#10000=CIRCLE('',#27010,0.0908032840555568);
#10001=CIRCLE('',#27019,0.095);
#10002=CIRCLE('',#27022,0.135);
#11885=VERTEX_POINT('',#48671);
#11886=VERTEX_POINT('',#48672);
#11887=VERTEX_POINT('',#48674);
#11888=VERTEX_POINT('',#48691);
#11889=VERTEX_POINT('',#48693);
#11890=VERTEX_POINT('',#48696);
#11891=VERTEX_POINT('',#48712);
#11892=VERTEX_POINT('',#48713);
#11893=VERTEX_POINT('',#48760);
#11894=VERTEX_POINT('',#48761);
#11895=VERTEX_POINT('',#48808);
#11896=VERTEX_POINT('',#48809);
#11897=VERTEX_POINT('',#48862);
#11898=VERTEX_POINT('',#48863);
#11899=VERTEX_POINT('',#48910);
#11900=VERTEX_POINT('',#48911);
#11901=VERTEX_POINT('',#48964);
#11902=VERTEX_POINT('',#48965);
#11903=VERTEX_POINT('',#49012);
#11904=VERTEX_POINT('',#49013);
#11905=VERTEX_POINT('',#49060);
#11906=VERTEX_POINT('',#49061);
#11907=VERTEX_POINT('',#49114);
#11908=VERTEX_POINT('',#49115);
#11909=VERTEX_POINT('',#49162);
#11910=VERTEX_POINT('',#49163);
#11911=VERTEX_POINT('',#49210);
#11912=VERTEX_POINT('',#49211);
#11913=VERTEX_POINT('',#49264);
#11914=VERTEX_POINT('',#49265);
#11915=VERTEX_POINT('',#49267);
#11916=VERTEX_POINT('',#49277);
#11917=VERTEX_POINT('',#49287);
#11918=VERTEX_POINT('',#49288);
#11919=VERTEX_POINT('',#49312);
#11920=VERTEX_POINT('',#49313);
#11921=VERTEX_POINT('',#49336);
#11922=VERTEX_POINT('',#49337);
#11923=VERTEX_POINT('',#49361);
#11924=VERTEX_POINT('',#49362);
#11925=VERTEX_POINT('',#49386);
#11926=VERTEX_POINT('',#49387);
#11927=VERTEX_POINT('',#49410);
#11928=VERTEX_POINT('',#49411);
#11929=VERTEX_POINT('',#49435);
#11930=VERTEX_POINT('',#49436);
#11931=VERTEX_POINT('',#49460);
#11932=VERTEX_POINT('',#49461);
#11933=VERTEX_POINT('',#49485);
#11934=VERTEX_POINT('',#49486);
#11935=VERTEX_POINT('',#49510);
#11936=VERTEX_POINT('',#49511);
#11937=VERTEX_POINT('',#49534);
#11938=VERTEX_POINT('',#49535);
#11939=VERTEX_POINT('',#49537);
#11940=VERTEX_POINT('',#49560);
#11941=VERTEX_POINT('',#49610);
#11942=VERTEX_POINT('',#49612);
#11943=VERTEX_POINT('',#49990);
#11944=VERTEX_POINT('',#50424);
#11945=VERTEX_POINT('',#50425);
#11946=VERTEX_POINT('',#50427);
#11947=VERTEX_POINT('',#50431);
#11948=VERTEX_POINT('',#50433);
#11949=VERTEX_POINT('',#50439);
#11950=VERTEX_POINT('',#50445);
#11951=VERTEX_POINT('',#50446);
#11952=VERTEX_POINT('',#50448);
#11953=VERTEX_POINT('',#50452);
#11954=VERTEX_POINT('',#50454);
#11955=VERTEX_POINT('',#50460);
#11956=VERTEX_POINT('',#50466);
#11957=VERTEX_POINT('',#50467);
#11958=VERTEX_POINT('',#50469);
#11959=VERTEX_POINT('',#50473);
#11960=VERTEX_POINT('',#50475);
#11961=VERTEX_POINT('',#50481);
#11962=VERTEX_POINT('',#50487);
#11963=VERTEX_POINT('',#50488);
#11964=VERTEX_POINT('',#50490);
#11965=VERTEX_POINT('',#50494);
#11966=VERTEX_POINT('',#50496);
#11967=VERTEX_POINT('',#50502);
#11968=VERTEX_POINT('',#50508);
#11969=VERTEX_POINT('',#50509);
#11970=VERTEX_POINT('',#50511);
#11971=VERTEX_POINT('',#50515);
#11972=VERTEX_POINT('',#50517);
#11973=VERTEX_POINT('',#50523);
#11974=VERTEX_POINT('',#50529);
#11975=VERTEX_POINT('',#50530);
#11976=VERTEX_POINT('',#50532);
#11977=VERTEX_POINT('',#50536);
#11978=VERTEX_POINT('',#50538);
#11979=VERTEX_POINT('',#50544);
#11980=VERTEX_POINT('',#50550);
#11981=VERTEX_POINT('',#50551);
#11982=VERTEX_POINT('',#50553);
#11983=VERTEX_POINT('',#50557);
#11984=VERTEX_POINT('',#50559);
#11985=VERTEX_POINT('',#50565);
#11986=VERTEX_POINT('',#50571);
#11987=VERTEX_POINT('',#50572);
#11988=VERTEX_POINT('',#50574);
#11989=VERTEX_POINT('',#50578);
#11990=VERTEX_POINT('',#50580);
#11991=VERTEX_POINT('',#50586);
#11992=VERTEX_POINT('',#50592);
#11993=VERTEX_POINT('',#50593);
#11994=VERTEX_POINT('',#50595);
#11995=VERTEX_POINT('',#50599);
#11996=VERTEX_POINT('',#50601);
#11997=VERTEX_POINT('',#50607);
#11998=VERTEX_POINT('',#50613);
#11999=VERTEX_POINT('',#50614);
#12000=VERTEX_POINT('',#50616);
#12001=VERTEX_POINT('',#50620);
#12002=VERTEX_POINT('',#50622);
#12003=VERTEX_POINT('',#50628);
#12004=VERTEX_POINT('',#50634);
#12005=VERTEX_POINT('',#50635);
#12006=VERTEX_POINT('',#50637);
#12007=VERTEX_POINT('',#50641);
#12008=VERTEX_POINT('',#50643);
#12009=VERTEX_POINT('',#50649);
#12010=VERTEX_POINT('',#50655);
#12011=VERTEX_POINT('',#50656);
#12012=VERTEX_POINT('',#50658);
#12013=VERTEX_POINT('',#50662);
#12014=VERTEX_POINT('',#50664);
#12015=VERTEX_POINT('',#50670);
#12016=VERTEX_POINT('',#50676);
#12017=VERTEX_POINT('',#50677);
#12018=VERTEX_POINT('',#50679);
#12019=VERTEX_POINT('',#50683);
#12020=VERTEX_POINT('',#50685);
#12021=VERTEX_POINT('',#50691);
#12022=VERTEX_POINT('',#50697);
#12023=VERTEX_POINT('',#50698);
#12024=VERTEX_POINT('',#50700);
#12025=VERTEX_POINT('',#50704);
#12026=VERTEX_POINT('',#50706);
#12027=VERTEX_POINT('',#50712);
#12028=VERTEX_POINT('',#50718);
#12029=VERTEX_POINT('',#50719);
#12030=VERTEX_POINT('',#50721);
#12031=VERTEX_POINT('',#50725);
#12032=VERTEX_POINT('',#50727);
#12033=VERTEX_POINT('',#50733);
#12034=VERTEX_POINT('',#50739);
#12035=VERTEX_POINT('',#50740);
#12036=VERTEX_POINT('',#50742);
#12037=VERTEX_POINT('',#50746);
#12038=VERTEX_POINT('',#50748);
#12039=VERTEX_POINT('',#50754);
#12040=VERTEX_POINT('',#50760);
#12041=VERTEX_POINT('',#50761);
#12042=VERTEX_POINT('',#50763);
#12043=VERTEX_POINT('',#50767);
#12044=VERTEX_POINT('',#50769);
#12045=VERTEX_POINT('',#50775);
#12046=VERTEX_POINT('',#50781);
#12047=VERTEX_POINT('',#50782);
#12048=VERTEX_POINT('',#50784);
#12049=VERTEX_POINT('',#50786);
#12050=VERTEX_POINT('',#50790);
#12051=VERTEX_POINT('',#50792);
#12052=VERTEX_POINT('',#50798);
#12053=VERTEX_POINT('',#50804);
#12054=VERTEX_POINT('',#50805);
#12055=VERTEX_POINT('',#50807);
#12056=VERTEX_POINT('',#50811);
#12057=VERTEX_POINT('',#50813);
#12058=VERTEX_POINT('',#50819);
#12059=VERTEX_POINT('',#50825);
#12060=VERTEX_POINT('',#50826);
#12061=VERTEX_POINT('',#50828);
#12062=VERTEX_POINT('',#50832);
#12063=VERTEX_POINT('',#50834);
#12064=VERTEX_POINT('',#50840);
#12065=VERTEX_POINT('',#50846);
#12066=VERTEX_POINT('',#50847);
#12067=VERTEX_POINT('',#50849);
#12068=VERTEX_POINT('',#50853);
#12069=VERTEX_POINT('',#50855);
#12070=VERTEX_POINT('',#50861);
#12071=VERTEX_POINT('',#50867);
#12072=VERTEX_POINT('',#50868);
#12073=VERTEX_POINT('',#50870);
#12074=VERTEX_POINT('',#50874);
#12075=VERTEX_POINT('',#50876);
#12076=VERTEX_POINT('',#50882);
#12077=VERTEX_POINT('',#50888);
#12078=VERTEX_POINT('',#50889);
#12079=VERTEX_POINT('',#50891);
#12080=VERTEX_POINT('',#50895);
#12081=VERTEX_POINT('',#50897);
#12082=VERTEX_POINT('',#50903);
#12083=VERTEX_POINT('',#50909);
#12084=VERTEX_POINT('',#50910);
#12085=VERTEX_POINT('',#50912);
#12086=VERTEX_POINT('',#50916);
#12087=VERTEX_POINT('',#50918);
#12088=VERTEX_POINT('',#50924);
#12089=VERTEX_POINT('',#50930);
#12090=VERTEX_POINT('',#50931);
#12091=VERTEX_POINT('',#50933);
#12092=VERTEX_POINT('',#50937);
#12093=VERTEX_POINT('',#50939);
#12094=VERTEX_POINT('',#50945);
#12095=VERTEX_POINT('',#50951);
#12096=VERTEX_POINT('',#50952);
#12097=VERTEX_POINT('',#50954);
#12098=VERTEX_POINT('',#50958);
#12099=VERTEX_POINT('',#50960);
#12100=VERTEX_POINT('',#50966);
#12101=VERTEX_POINT('',#50972);
#12102=VERTEX_POINT('',#50973);
#12103=VERTEX_POINT('',#50975);
#12104=VERTEX_POINT('',#50979);
#12105=VERTEX_POINT('',#50981);
#12106=VERTEX_POINT('',#50987);
#12107=VERTEX_POINT('',#50993);
#12108=VERTEX_POINT('',#50994);
#12109=VERTEX_POINT('',#50996);
#12110=VERTEX_POINT('',#51000);
#12111=VERTEX_POINT('',#51002);
#12112=VERTEX_POINT('',#51008);
#12113=VERTEX_POINT('',#51014);
#12114=VERTEX_POINT('',#51015);
#12115=VERTEX_POINT('',#51017);
#12116=VERTEX_POINT('',#51021);
#12117=VERTEX_POINT('',#51023);
#12118=VERTEX_POINT('',#51029);
#12119=VERTEX_POINT('',#51035);
#12120=VERTEX_POINT('',#51036);
#12121=VERTEX_POINT('',#51038);
#12122=VERTEX_POINT('',#51042);
#12123=VERTEX_POINT('',#51044);
#12124=VERTEX_POINT('',#51050);
#12125=VERTEX_POINT('',#51056);
#12126=VERTEX_POINT('',#51057);
#12127=VERTEX_POINT('',#51059);
#12128=VERTEX_POINT('',#51063);
#12129=VERTEX_POINT('',#51065);
#12130=VERTEX_POINT('',#51071);
#12131=VERTEX_POINT('',#51077);
#12132=VERTEX_POINT('',#51078);
#12133=VERTEX_POINT('',#51080);
#12134=VERTEX_POINT('',#51084);
#12135=VERTEX_POINT('',#51086);
#12136=VERTEX_POINT('',#51092);
#12137=VERTEX_POINT('',#51098);
#12138=VERTEX_POINT('',#51099);
#12139=VERTEX_POINT('',#51101);
#12140=VERTEX_POINT('',#51105);
#12141=VERTEX_POINT('',#51107);
#12142=VERTEX_POINT('',#51113);
#12143=VERTEX_POINT('',#51119);
#12144=VERTEX_POINT('',#51120);
#12145=VERTEX_POINT('',#51122);
#12146=VERTEX_POINT('',#51126);
#12147=VERTEX_POINT('',#51128);
#12148=VERTEX_POINT('',#51134);
#12149=VERTEX_POINT('',#51140);
#12150=VERTEX_POINT('',#51141);
#12151=VERTEX_POINT('',#51143);
#12152=VERTEX_POINT('',#51147);
#12153=VERTEX_POINT('',#51149);
#12154=VERTEX_POINT('',#51155);
#12155=VERTEX_POINT('',#51178);
#12156=VERTEX_POINT('',#51198);
#12157=VERTEX_POINT('',#51200);
#12158=VERTEX_POINT('',#51202);
#12159=VERTEX_POINT('',#51204);
#12160=VERTEX_POINT('',#51208);
#12161=VERTEX_POINT('',#51210);
#12162=VERTEX_POINT('',#51222);
#12163=VERTEX_POINT('',#51226);
#12164=VERTEX_POINT('',#51227);
#12165=VERTEX_POINT('',#51231);
#12166=VERTEX_POINT('',#51232);
#12167=VERTEX_POINT('',#51234);
#12168=VERTEX_POINT('',#51236);
#12169=VERTEX_POINT('',#51240);
#12170=VERTEX_POINT('',#51242);
#12171=VERTEX_POINT('',#51246);
#12172=VERTEX_POINT('',#51248);
#12173=VERTEX_POINT('',#51252);
#12174=VERTEX_POINT('',#51254);
#12175=VERTEX_POINT('',#51258);
#12176=VERTEX_POINT('',#51260);
#12177=VERTEX_POINT('',#51268);
#12178=VERTEX_POINT('',#51273);
#15184=EDGE_CURVE('',#11885,#11886,#6845,.T.);
#15185=EDGE_CURVE('',#11885,#11887,#790,.T.);
#15186=EDGE_CURVE('',#11887,#11888,#9916,.T.);
#15187=EDGE_CURVE('',#11888,#11889,#6846,.T.);
#15188=EDGE_CURVE('',#11889,#11889,#9917,.T.);
#15189=EDGE_CURVE('',#11888,#11890,#9918,.T.);
#15190=EDGE_CURVE('',#11890,#11886,#791,.T.);
#15191=EDGE_CURVE('',#11891,#11892,#6847,.T.);
#15192=EDGE_CURVE('',#11891,#11885,#792,.T.);
#15193=EDGE_CURVE('',#11886,#11892,#793,.T.);
#15194=EDGE_CURVE('',#11893,#11894,#6848,.T.);
#15195=EDGE_CURVE('',#11893,#11891,#794,.T.);
#15196=EDGE_CURVE('',#11892,#11894,#795,.T.);
#15197=EDGE_CURVE('',#11895,#11896,#6849,.T.);
#15198=EDGE_CURVE('',#11895,#11893,#796,.T.);
#15199=EDGE_CURVE('',#11894,#11896,#797,.T.);
#15200=EDGE_CURVE('',#11897,#11898,#6850,.T.);
#15201=EDGE_CURVE('',#11897,#11895,#798,.T.);
#15202=EDGE_CURVE('',#11896,#11898,#799,.T.);
#15203=EDGE_CURVE('',#11899,#11900,#6851,.T.);
#15204=EDGE_CURVE('',#11899,#11897,#800,.T.);
#15205=EDGE_CURVE('',#11898,#11900,#801,.T.);
#15206=EDGE_CURVE('',#11901,#11902,#6852,.T.);
#15207=EDGE_CURVE('',#11901,#11899,#802,.T.);
#15208=EDGE_CURVE('',#11900,#11902,#803,.T.);
#15209=EDGE_CURVE('',#11903,#11904,#6853,.T.);
#15210=EDGE_CURVE('',#11903,#11901,#804,.T.);
#15211=EDGE_CURVE('',#11902,#11904,#805,.T.);
#15212=EDGE_CURVE('',#11905,#11906,#6854,.T.);
#15213=EDGE_CURVE('',#11905,#11903,#806,.T.);
#15214=EDGE_CURVE('',#11904,#11906,#807,.T.);
#15215=EDGE_CURVE('',#11907,#11908,#6855,.T.);
#15216=EDGE_CURVE('',#11907,#11905,#808,.T.);
#15217=EDGE_CURVE('',#11906,#11908,#809,.T.);
#15218=EDGE_CURVE('',#11909,#11910,#6856,.T.);
#15219=EDGE_CURVE('',#11909,#11907,#810,.T.);
#15220=EDGE_CURVE('',#11908,#11910,#811,.T.);
#15221=EDGE_CURVE('',#11911,#11912,#6857,.T.);
#15222=EDGE_CURVE('',#11911,#11909,#812,.T.);
#15223=EDGE_CURVE('',#11910,#11912,#813,.T.);
#15224=EDGE_CURVE('',#11913,#11914,#6858,.T.);
#15225=EDGE_CURVE('',#11913,#11915,#814,.T.);
#15226=EDGE_CURVE('',#11916,#11915,#9919,.T.);
#15227=EDGE_CURVE('',#11914,#11916,#815,.T.);
#15228=EDGE_CURVE('',#11917,#11918,#6859,.T.);
#15229=EDGE_CURVE('',#11917,#11913,#816,.T.);
#15230=EDGE_CURVE('',#11918,#11914,#817,.T.);
#15231=EDGE_CURVE('',#11919,#11920,#6860,.T.);
#15232=EDGE_CURVE('',#11919,#11917,#818,.T.);
#15233=EDGE_CURVE('',#11920,#11918,#819,.T.);
#15234=EDGE_CURVE('',#11921,#11922,#6861,.T.);
#15235=EDGE_CURVE('',#11921,#11919,#820,.T.);
#15236=EDGE_CURVE('',#11922,#11920,#821,.T.);
#15237=EDGE_CURVE('',#11923,#11924,#6862,.T.);
#15238=EDGE_CURVE('',#11923,#11921,#822,.T.);
#15239=EDGE_CURVE('',#11924,#11922,#823,.T.);
#15240=EDGE_CURVE('',#11925,#11926,#6863,.T.);
#15241=EDGE_CURVE('',#11925,#11923,#824,.T.);
#15242=EDGE_CURVE('',#11926,#11924,#825,.T.);
#15243=EDGE_CURVE('',#11927,#11928,#6864,.T.);
#15244=EDGE_CURVE('',#11927,#11925,#826,.T.);
#15245=EDGE_CURVE('',#11928,#11926,#827,.T.);
#15246=EDGE_CURVE('',#11929,#11930,#6865,.T.);
#15247=EDGE_CURVE('',#11929,#11927,#828,.T.);
#15248=EDGE_CURVE('',#11930,#11928,#829,.T.);
#15249=EDGE_CURVE('',#11931,#11932,#6866,.T.);
#15250=EDGE_CURVE('',#11931,#11929,#830,.T.);
#15251=EDGE_CURVE('',#11932,#11930,#831,.T.);
#15252=EDGE_CURVE('',#11933,#11934,#6867,.T.);
#15253=EDGE_CURVE('',#11933,#11931,#832,.T.);
#15254=EDGE_CURVE('',#11934,#11932,#833,.T.);
#15255=EDGE_CURVE('',#11935,#11936,#6868,.T.);
#15256=EDGE_CURVE('',#11935,#11933,#834,.T.);
#15257=EDGE_CURVE('',#11936,#11934,#835,.T.);
#15258=EDGE_CURVE('',#11937,#11938,#6869,.T.);
#15259=EDGE_CURVE('',#11939,#11937,#9920,.T.);
#15260=EDGE_CURVE('',#11939,#11935,#836,.T.);
#15261=EDGE_CURVE('',#11938,#11936,#837,.T.);
#15262=EDGE_CURVE('',#11915,#11940,#838,.T.);
#15263=EDGE_CURVE('',#11941,#11940,#9921,.T.);
#15264=EDGE_CURVE('',#11942,#11941,#9922,.T.);
#15265=EDGE_CURVE('',#11942,#11916,#839,.T.);
#15266=EDGE_CURVE('',#11912,#11942,#840,.T.);
#15267=EDGE_CURVE('',#11943,#11890,#841,.T.);
#15268=EDGE_CURVE('',#11943,#11938,#842,.T.);
#15269=EDGE_CURVE('',#11887,#11939,#843,.T.);
#15270=EDGE_CURVE('',#11937,#11943,#9923,.T.);
#15271=EDGE_CURVE('',#11940,#11911,#844,.T.);
#15272=EDGE_CURVE('',#11940,#11942,#9924,.T.);
#15273=EDGE_CURVE('',#11944,#11945,#9925,.T.);
#15274=EDGE_CURVE('',#11944,#11946,#6870,.T.);
#15275=EDGE_CURVE('',#11946,#11945,#6871,.T.);
#15276=EDGE_CURVE('',#11945,#11947,#6872,.T.);
#15277=EDGE_CURVE('',#11946,#11948,#6873,.T.);
#15278=EDGE_CURVE('',#11947,#11948,#395,.T.);
#15279=EDGE_CURVE('',#11949,#11944,#6874,.T.);
#15280=EDGE_CURVE('',#11948,#11949,#396,.T.);
#15281=EDGE_CURVE('',#11950,#11951,#9926,.T.);
#15282=EDGE_CURVE('',#11950,#11952,#6875,.T.);
#15283=EDGE_CURVE('',#11952,#11951,#6876,.T.);
#15284=EDGE_CURVE('',#11951,#11953,#6877,.T.);
#15285=EDGE_CURVE('',#11952,#11954,#6878,.T.);
#15286=EDGE_CURVE('',#11953,#11954,#397,.T.);
#15287=EDGE_CURVE('',#11955,#11950,#6879,.T.);
#15288=EDGE_CURVE('',#11954,#11955,#398,.T.);
#15289=EDGE_CURVE('',#11956,#11957,#9927,.T.);
#15290=EDGE_CURVE('',#11956,#11958,#6880,.T.);
#15291=EDGE_CURVE('',#11958,#11957,#6881,.T.);
#15292=EDGE_CURVE('',#11957,#11959,#6882,.T.);
#15293=EDGE_CURVE('',#11958,#11960,#6883,.T.);
#15294=EDGE_CURVE('',#11959,#11960,#399,.T.);
#15295=EDGE_CURVE('',#11961,#11956,#6884,.T.);
#15296=EDGE_CURVE('',#11960,#11961,#400,.T.);
#15297=EDGE_CURVE('',#11962,#11963,#9928,.T.);
#15298=EDGE_CURVE('',#11962,#11964,#6885,.T.);
#15299=EDGE_CURVE('',#11964,#11963,#6886,.T.);
#15300=EDGE_CURVE('',#11963,#11965,#6887,.T.);
#15301=EDGE_CURVE('',#11964,#11966,#6888,.T.);
#15302=EDGE_CURVE('',#11965,#11966,#401,.T.);
#15303=EDGE_CURVE('',#11967,#11962,#6889,.T.);
#15304=EDGE_CURVE('',#11966,#11967,#402,.T.);
#15305=EDGE_CURVE('',#11968,#11969,#9929,.T.);
#15306=EDGE_CURVE('',#11968,#11970,#6890,.T.);
#15307=EDGE_CURVE('',#11970,#11969,#6891,.T.);
#15308=EDGE_CURVE('',#11969,#11971,#6892,.T.);
#15309=EDGE_CURVE('',#11970,#11972,#6893,.T.);
#15310=EDGE_CURVE('',#11971,#11972,#403,.T.);
#15311=EDGE_CURVE('',#11973,#11968,#6894,.T.);
#15312=EDGE_CURVE('',#11972,#11973,#404,.T.);
#15313=EDGE_CURVE('',#11974,#11975,#9930,.T.);
#15314=EDGE_CURVE('',#11974,#11976,#6895,.T.);
#15315=EDGE_CURVE('',#11976,#11975,#6896,.T.);
#15316=EDGE_CURVE('',#11975,#11977,#6897,.T.);
#15317=EDGE_CURVE('',#11976,#11978,#6898,.T.);
#15318=EDGE_CURVE('',#11977,#11978,#405,.T.);
#15319=EDGE_CURVE('',#11979,#11974,#6899,.T.);
#15320=EDGE_CURVE('',#11978,#11979,#406,.T.);
#15321=EDGE_CURVE('',#11980,#11981,#9931,.T.);
#15322=EDGE_CURVE('',#11980,#11982,#6900,.T.);
#15323=EDGE_CURVE('',#11982,#11981,#6901,.T.);
#15324=EDGE_CURVE('',#11981,#11983,#6902,.T.);
#15325=EDGE_CURVE('',#11982,#11984,#6903,.T.);
#15326=EDGE_CURVE('',#11983,#11984,#407,.T.);
#15327=EDGE_CURVE('',#11985,#11980,#6904,.T.);
#15328=EDGE_CURVE('',#11984,#11985,#408,.T.);
#15329=EDGE_CURVE('',#11986,#11987,#9932,.T.);
#15330=EDGE_CURVE('',#11986,#11988,#6905,.T.);
#15331=EDGE_CURVE('',#11988,#11987,#6906,.T.);
#15332=EDGE_CURVE('',#11987,#11989,#6907,.T.);
#15333=EDGE_CURVE('',#11988,#11990,#6908,.T.);
#15334=EDGE_CURVE('',#11989,#11990,#409,.T.);
#15335=EDGE_CURVE('',#11991,#11986,#6909,.T.);
#15336=EDGE_CURVE('',#11990,#11991,#410,.T.);
#15337=EDGE_CURVE('',#11992,#11993,#9933,.T.);
#15338=EDGE_CURVE('',#11992,#11994,#6910,.T.);
#15339=EDGE_CURVE('',#11994,#11993,#6911,.T.);
#15340=EDGE_CURVE('',#11993,#11995,#6912,.T.);
#15341=EDGE_CURVE('',#11994,#11996,#6913,.T.);
#15342=EDGE_CURVE('',#11995,#11996,#411,.T.);
#15343=EDGE_CURVE('',#11997,#11992,#6914,.T.);
#15344=EDGE_CURVE('',#11996,#11997,#412,.T.);
#15345=EDGE_CURVE('',#11998,#11999,#9934,.T.);
#15346=EDGE_CURVE('',#11998,#12000,#6915,.T.);
#15347=EDGE_CURVE('',#12000,#11999,#6916,.T.);
#15348=EDGE_CURVE('',#11999,#12001,#6917,.T.);
#15349=EDGE_CURVE('',#12000,#12002,#6918,.T.);
#15350=EDGE_CURVE('',#12001,#12002,#413,.T.);
#15351=EDGE_CURVE('',#12003,#11998,#6919,.T.);
#15352=EDGE_CURVE('',#12002,#12003,#414,.T.);
#15353=EDGE_CURVE('',#12004,#12005,#9935,.T.);
#15354=EDGE_CURVE('',#12004,#12006,#6920,.T.);
#15355=EDGE_CURVE('',#12006,#12005,#6921,.T.);
#15356=EDGE_CURVE('',#12005,#12007,#6922,.T.);
#15357=EDGE_CURVE('',#12006,#12008,#6923,.T.);
#15358=EDGE_CURVE('',#12007,#12008,#415,.T.);
#15359=EDGE_CURVE('',#12009,#12004,#6924,.T.);
#15360=EDGE_CURVE('',#12008,#12009,#416,.T.);
#15361=EDGE_CURVE('',#12010,#12011,#9936,.T.);
#15362=EDGE_CURVE('',#12010,#12012,#6925,.T.);
#15363=EDGE_CURVE('',#12012,#12011,#6926,.T.);
#15364=EDGE_CURVE('',#12011,#12013,#6927,.T.);
#15365=EDGE_CURVE('',#12012,#12014,#6928,.T.);
#15366=EDGE_CURVE('',#12013,#12014,#417,.T.);
#15367=EDGE_CURVE('',#12015,#12010,#6929,.T.);
#15368=EDGE_CURVE('',#12014,#12015,#418,.T.);
#15369=EDGE_CURVE('',#12016,#12017,#9937,.T.);
#15370=EDGE_CURVE('',#12016,#12018,#6930,.T.);
#15371=EDGE_CURVE('',#12018,#12017,#6931,.T.);
#15372=EDGE_CURVE('',#12017,#12019,#6932,.T.);
#15373=EDGE_CURVE('',#12018,#12020,#6933,.T.);
#15374=EDGE_CURVE('',#12019,#12020,#419,.T.);
#15375=EDGE_CURVE('',#12021,#12016,#6934,.T.);
#15376=EDGE_CURVE('',#12020,#12021,#420,.T.);
#15377=EDGE_CURVE('',#12022,#12023,#9938,.T.);
#15378=EDGE_CURVE('',#12022,#12024,#6935,.T.);
#15379=EDGE_CURVE('',#12024,#12023,#6936,.T.);
#15380=EDGE_CURVE('',#12023,#12025,#6937,.T.);
#15381=EDGE_CURVE('',#12024,#12026,#6938,.T.);
#15382=EDGE_CURVE('',#12025,#12026,#421,.T.);
#15383=EDGE_CURVE('',#12027,#12022,#6939,.T.);
#15384=EDGE_CURVE('',#12026,#12027,#422,.T.);
#15385=EDGE_CURVE('',#12028,#12029,#9939,.T.);
#15386=EDGE_CURVE('',#12028,#12030,#6940,.T.);
#15387=EDGE_CURVE('',#12030,#12029,#6941,.T.);
#15388=EDGE_CURVE('',#12029,#12031,#6942,.T.);
#15389=EDGE_CURVE('',#12030,#12032,#6943,.T.);
#15390=EDGE_CURVE('',#12031,#12032,#423,.T.);
#15391=EDGE_CURVE('',#12033,#12028,#6944,.T.);
#15392=EDGE_CURVE('',#12032,#12033,#424,.T.);
#15393=EDGE_CURVE('',#12034,#12035,#9940,.T.);
#15394=EDGE_CURVE('',#12034,#12036,#6945,.T.);
#15395=EDGE_CURVE('',#12036,#12035,#6946,.T.);
#15396=EDGE_CURVE('',#12035,#12037,#6947,.T.);
#15397=EDGE_CURVE('',#12036,#12038,#6948,.T.);
#15398=EDGE_CURVE('',#12037,#12038,#425,.T.);
#15399=EDGE_CURVE('',#12039,#12034,#6949,.T.);
#15400=EDGE_CURVE('',#12038,#12039,#426,.T.);
#15401=EDGE_CURVE('',#12040,#12041,#9941,.T.);
#15402=EDGE_CURVE('',#12040,#12042,#6950,.T.);
#15403=EDGE_CURVE('',#12042,#12041,#6951,.T.);
#15404=EDGE_CURVE('',#12041,#12043,#6952,.T.);
#15405=EDGE_CURVE('',#12042,#12044,#6953,.T.);
#15406=EDGE_CURVE('',#12043,#12044,#427,.T.);
#15407=EDGE_CURVE('',#12045,#12040,#6954,.T.);
#15408=EDGE_CURVE('',#12044,#12045,#428,.T.);
#15409=EDGE_CURVE('',#12046,#12047,#9942,.T.);
#15410=EDGE_CURVE('',#12046,#12048,#6955,.T.);
#15411=EDGE_CURVE('',#12048,#12049,#6956,.T.);
#15412=EDGE_CURVE('',#12047,#12049,#9943,.T.);
#15413=EDGE_CURVE('',#12049,#12050,#6957,.T.);
#15414=EDGE_CURVE('',#12048,#12051,#6958,.T.);
#15415=EDGE_CURVE('',#12050,#12051,#429,.T.);
#15416=EDGE_CURVE('',#12052,#12046,#6959,.T.);
#15417=EDGE_CURVE('',#12051,#12052,#430,.T.);
#15418=EDGE_CURVE('',#12053,#12054,#9944,.T.);
#15419=EDGE_CURVE('',#12053,#12055,#6960,.T.);
#15420=EDGE_CURVE('',#12055,#12054,#6961,.T.);
#15421=EDGE_CURVE('',#12054,#12056,#6962,.T.);
#15422=EDGE_CURVE('',#12055,#12057,#6963,.T.);
#15423=EDGE_CURVE('',#12056,#12057,#431,.T.);
#15424=EDGE_CURVE('',#12058,#12053,#6964,.T.);
#15425=EDGE_CURVE('',#12057,#12058,#432,.T.);
#15426=EDGE_CURVE('',#12059,#12060,#9945,.T.);
#15427=EDGE_CURVE('',#12059,#12061,#6965,.T.);
#15428=EDGE_CURVE('',#12061,#12060,#6966,.T.);
#15429=EDGE_CURVE('',#12060,#12062,#6967,.T.);
#15430=EDGE_CURVE('',#12061,#12063,#6968,.T.);
#15431=EDGE_CURVE('',#12062,#12063,#433,.T.);
#15432=EDGE_CURVE('',#12064,#12059,#6969,.T.);
#15433=EDGE_CURVE('',#12063,#12064,#434,.T.);
#15434=EDGE_CURVE('',#12065,#12066,#9946,.T.);
#15435=EDGE_CURVE('',#12065,#12067,#6970,.T.);
#15436=EDGE_CURVE('',#12067,#12066,#6971,.T.);
#15437=EDGE_CURVE('',#12066,#12068,#6972,.T.);
#15438=EDGE_CURVE('',#12067,#12069,#6973,.T.);
#15439=EDGE_CURVE('',#12068,#12069,#435,.T.);
#15440=EDGE_CURVE('',#12070,#12065,#6974,.T.);
#15441=EDGE_CURVE('',#12069,#12070,#436,.T.);
#15442=EDGE_CURVE('',#12071,#12072,#9947,.T.);
#15443=EDGE_CURVE('',#12071,#12073,#6975,.T.);
#15444=EDGE_CURVE('',#12073,#12072,#6976,.T.);
#15445=EDGE_CURVE('',#12072,#12074,#6977,.T.);
#15446=EDGE_CURVE('',#12073,#12075,#6978,.T.);
#15447=EDGE_CURVE('',#12074,#12075,#437,.T.);
#15448=EDGE_CURVE('',#12076,#12071,#6979,.T.);
#15449=EDGE_CURVE('',#12075,#12076,#438,.T.);
#15450=EDGE_CURVE('',#12077,#12078,#9948,.T.);
#15451=EDGE_CURVE('',#12077,#12079,#6980,.T.);
#15452=EDGE_CURVE('',#12079,#12078,#6981,.T.);
#15453=EDGE_CURVE('',#12078,#12080,#6982,.T.);
#15454=EDGE_CURVE('',#12079,#12081,#6983,.T.);
#15455=EDGE_CURVE('',#12080,#12081,#439,.T.);
#15456=EDGE_CURVE('',#12082,#12077,#6984,.T.);
#15457=EDGE_CURVE('',#12081,#12082,#440,.T.);
#15458=EDGE_CURVE('',#12083,#12084,#9949,.T.);
#15459=EDGE_CURVE('',#12083,#12085,#6985,.T.);
#15460=EDGE_CURVE('',#12085,#12084,#6986,.T.);
#15461=EDGE_CURVE('',#12084,#12086,#6987,.T.);
#15462=EDGE_CURVE('',#12085,#12087,#6988,.T.);
#15463=EDGE_CURVE('',#12086,#12087,#441,.T.);
#15464=EDGE_CURVE('',#12088,#12083,#6989,.T.);
#15465=EDGE_CURVE('',#12087,#12088,#442,.T.);
#15466=EDGE_CURVE('',#12089,#12090,#9950,.T.);
#15467=EDGE_CURVE('',#12089,#12091,#6990,.T.);
#15468=EDGE_CURVE('',#12091,#12090,#6991,.T.);
#15469=EDGE_CURVE('',#12090,#12092,#6992,.T.);
#15470=EDGE_CURVE('',#12091,#12093,#6993,.T.);
#15471=EDGE_CURVE('',#12092,#12093,#443,.T.);
#15472=EDGE_CURVE('',#12094,#12089,#6994,.T.);
#15473=EDGE_CURVE('',#12093,#12094,#444,.T.);
#15474=EDGE_CURVE('',#12095,#12096,#9951,.T.);
#15475=EDGE_CURVE('',#12095,#12097,#6995,.T.);
#15476=EDGE_CURVE('',#12097,#12096,#6996,.T.);
#15477=EDGE_CURVE('',#12096,#12098,#6997,.T.);
#15478=EDGE_CURVE('',#12097,#12099,#6998,.T.);
#15479=EDGE_CURVE('',#12098,#12099,#445,.T.);
#15480=EDGE_CURVE('',#12100,#12095,#6999,.T.);
#15481=EDGE_CURVE('',#12099,#12100,#446,.T.);
#15482=EDGE_CURVE('',#12101,#12102,#9952,.T.);
#15483=EDGE_CURVE('',#12101,#12103,#7000,.T.);
#15484=EDGE_CURVE('',#12103,#12102,#7001,.T.);
#15485=EDGE_CURVE('',#12102,#12104,#7002,.T.);
#15486=EDGE_CURVE('',#12103,#12105,#7003,.T.);
#15487=EDGE_CURVE('',#12104,#12105,#447,.T.);
#15488=EDGE_CURVE('',#12106,#12101,#7004,.T.);
#15489=EDGE_CURVE('',#12105,#12106,#448,.T.);
#15490=EDGE_CURVE('',#12107,#12108,#9953,.T.);
#15491=EDGE_CURVE('',#12107,#12109,#7005,.T.);
#15492=EDGE_CURVE('',#12109,#12108,#7006,.T.);
#15493=EDGE_CURVE('',#12108,#12110,#7007,.T.);
#15494=EDGE_CURVE('',#12109,#12111,#7008,.T.);
#15495=EDGE_CURVE('',#12110,#12111,#449,.T.);
#15496=EDGE_CURVE('',#12112,#12107,#7009,.T.);
#15497=EDGE_CURVE('',#12111,#12112,#450,.T.);
#15498=EDGE_CURVE('',#12113,#12114,#9954,.T.);
#15499=EDGE_CURVE('',#12113,#12115,#7010,.T.);
#15500=EDGE_CURVE('',#12115,#12114,#7011,.T.);
#15501=EDGE_CURVE('',#12114,#12116,#7012,.T.);
#15502=EDGE_CURVE('',#12115,#12117,#7013,.T.);
#15503=EDGE_CURVE('',#12116,#12117,#451,.T.);
#15504=EDGE_CURVE('',#12118,#12113,#7014,.T.);
#15505=EDGE_CURVE('',#12117,#12118,#452,.T.);
#15506=EDGE_CURVE('',#12119,#12120,#9955,.T.);
#15507=EDGE_CURVE('',#12119,#12121,#7015,.T.);
#15508=EDGE_CURVE('',#12121,#12120,#7016,.T.);
#15509=EDGE_CURVE('',#12120,#12122,#7017,.T.);
#15510=EDGE_CURVE('',#12121,#12123,#7018,.T.);
#15511=EDGE_CURVE('',#12122,#12123,#453,.T.);
#15512=EDGE_CURVE('',#12124,#12119,#7019,.T.);
#15513=EDGE_CURVE('',#12123,#12124,#454,.T.);
#15514=EDGE_CURVE('',#12125,#12126,#9956,.T.);
#15515=EDGE_CURVE('',#12125,#12127,#7020,.T.);
#15516=EDGE_CURVE('',#12127,#12126,#7021,.T.);
#15517=EDGE_CURVE('',#12126,#12128,#7022,.T.);
#15518=EDGE_CURVE('',#12127,#12129,#7023,.T.);
#15519=EDGE_CURVE('',#12128,#12129,#455,.T.);
#15520=EDGE_CURVE('',#12130,#12125,#7024,.T.);
#15521=EDGE_CURVE('',#12129,#12130,#456,.T.);
#15522=EDGE_CURVE('',#12131,#12132,#9957,.T.);
#15523=EDGE_CURVE('',#12131,#12133,#7025,.T.);
#15524=EDGE_CURVE('',#12133,#12132,#7026,.T.);
#15525=EDGE_CURVE('',#12132,#12134,#7027,.T.);
#15526=EDGE_CURVE('',#12133,#12135,#7028,.T.);
#15527=EDGE_CURVE('',#12134,#12135,#457,.T.);
#15528=EDGE_CURVE('',#12136,#12131,#7029,.T.);
#15529=EDGE_CURVE('',#12135,#12136,#458,.T.);
#15530=EDGE_CURVE('',#12137,#12138,#9958,.T.);
#15531=EDGE_CURVE('',#12137,#12139,#7030,.T.);
#15532=EDGE_CURVE('',#12139,#12138,#7031,.T.);
#15533=EDGE_CURVE('',#12138,#12140,#7032,.T.);
#15534=EDGE_CURVE('',#12139,#12141,#7033,.T.);
#15535=EDGE_CURVE('',#12140,#12141,#459,.T.);
#15536=EDGE_CURVE('',#12142,#12137,#7034,.T.);
#15537=EDGE_CURVE('',#12141,#12142,#460,.T.);
#15538=EDGE_CURVE('',#12143,#12144,#9959,.T.);
#15539=EDGE_CURVE('',#12143,#12145,#7035,.T.);
#15540=EDGE_CURVE('',#12145,#12144,#7036,.T.);
#15541=EDGE_CURVE('',#12144,#12146,#7037,.T.);
#15542=EDGE_CURVE('',#12145,#12147,#7038,.T.);
#15543=EDGE_CURVE('',#12146,#12147,#461,.T.);
#15544=EDGE_CURVE('',#12148,#12143,#7039,.T.);
#15545=EDGE_CURVE('',#12147,#12148,#462,.T.);
#15546=EDGE_CURVE('',#12149,#12150,#9960,.T.);
#15547=EDGE_CURVE('',#12149,#12151,#7040,.T.);
#15548=EDGE_CURVE('',#12151,#12150,#7041,.T.);
#15549=EDGE_CURVE('',#12150,#12152,#7042,.T.);
#15550=EDGE_CURVE('',#12151,#12153,#7043,.T.);
#15551=EDGE_CURVE('',#12152,#12153,#463,.T.);
#15552=EDGE_CURVE('',#12154,#12149,#7044,.T.);
#15553=EDGE_CURVE('',#12153,#12154,#464,.T.);
#15554=EDGE_CURVE('',#11955,#11947,#9961,.T.);
#15555=EDGE_CURVE('',#11961,#11953,#9962,.T.);
#15556=EDGE_CURVE('',#11967,#11959,#9963,.T.);
#15557=EDGE_CURVE('',#11973,#11965,#9964,.T.);
#15558=EDGE_CURVE('',#11979,#11971,#9965,.T.);
#15559=EDGE_CURVE('',#11985,#11977,#9966,.T.);
#15560=EDGE_CURVE('',#11991,#11983,#9967,.T.);
#15561=EDGE_CURVE('',#11997,#11989,#9968,.T.);
#15562=EDGE_CURVE('',#12003,#11995,#9969,.T.);
#15563=EDGE_CURVE('',#12009,#12001,#9970,.T.);
#15564=EDGE_CURVE('',#12015,#12007,#9971,.T.);
#15565=EDGE_CURVE('',#12021,#12013,#9972,.T.);
#15566=EDGE_CURVE('',#12027,#12019,#9973,.T.);
#15567=EDGE_CURVE('',#12033,#12025,#9974,.T.);
#15568=EDGE_CURVE('',#12039,#12031,#9975,.T.);
#15569=EDGE_CURVE('',#12045,#12037,#9976,.T.);
#15570=EDGE_CURVE('',#12052,#12043,#9977,.T.);
#15571=EDGE_CURVE('',#12047,#12155,#7045,.T.);
#15572=EDGE_CURVE('',#12155,#12155,#9978,.T.);
#15573=EDGE_CURVE('',#12058,#12050,#9979,.T.);
#15574=EDGE_CURVE('',#12064,#12056,#9980,.T.);
#15575=EDGE_CURVE('',#12070,#12062,#9981,.T.);
#15576=EDGE_CURVE('',#12076,#12068,#9982,.T.);
#15577=EDGE_CURVE('',#12082,#12074,#9983,.T.);
#15578=EDGE_CURVE('',#12088,#12080,#9984,.T.);
#15579=EDGE_CURVE('',#12094,#12086,#9985,.T.);
#15580=EDGE_CURVE('',#12100,#12092,#9986,.T.);
#15581=EDGE_CURVE('',#12106,#12098,#9987,.T.);
#15582=EDGE_CURVE('',#12112,#12104,#9988,.T.);
#15583=EDGE_CURVE('',#12118,#12110,#9989,.T.);
#15584=EDGE_CURVE('',#12124,#12116,#9990,.T.);
#15585=EDGE_CURVE('',#12130,#12122,#9991,.T.);
#15586=EDGE_CURVE('',#12136,#12128,#9992,.T.);
#15587=EDGE_CURVE('',#12142,#12134,#9993,.T.);
#15588=EDGE_CURVE('',#12148,#12140,#9994,.T.);
#15589=EDGE_CURVE('',#12154,#12146,#9995,.T.);
#15590=EDGE_CURVE('',#12156,#12152,#9996,.T.);
#15591=EDGE_CURVE('',#12156,#12157,#7046,.T.);
#15592=EDGE_CURVE('',#12157,#12158,#9997,.T.);
#15593=EDGE_CURVE('',#12158,#12159,#7047,.T.);
#15594=EDGE_CURVE('',#11949,#12159,#9998,.T.);
#15595=EDGE_CURVE('',#12160,#12158,#7048,.T.);
#15596=EDGE_CURVE('',#12160,#12161,#7049,.T.);
#15597=EDGE_CURVE('',#12159,#12161,#465,.T.);
#15598=EDGE_CURVE('',#12161,#12156,#466,.T.);
#15599=EDGE_CURVE('',#12157,#12160,#7050,.T.);
#15600=EDGE_CURVE('',#12162,#12162,#9999,.T.);
#15601=EDGE_CURVE('',#12162,#12051,#7051,.T.);
#15602=EDGE_CURVE('',#12163,#12164,#7052,.T.);
#15603=EDGE_CURVE('',#12164,#12164,#10000,.T.);
#15604=EDGE_CURVE('',#12165,#12166,#7053,.T.);
#15605=EDGE_CURVE('',#12165,#12167,#7054,.T.);
#15606=EDGE_CURVE('',#12167,#12168,#7055,.T.);
#15607=EDGE_CURVE('',#12166,#12168,#7056,.T.);
#15608=EDGE_CURVE('',#12169,#12165,#7057,.T.);
#15609=EDGE_CURVE('',#12169,#12170,#7058,.T.);
#15610=EDGE_CURVE('',#12170,#12167,#7059,.T.);
#15611=EDGE_CURVE('',#12171,#12169,#7060,.T.);
#15612=EDGE_CURVE('',#12171,#12172,#7061,.T.);
#15613=EDGE_CURVE('',#12172,#12170,#7062,.T.);
#15614=EDGE_CURVE('',#12173,#12171,#7063,.T.);
#15615=EDGE_CURVE('',#12173,#12174,#7064,.T.);
#15616=EDGE_CURVE('',#12174,#12172,#7065,.T.);
#15617=EDGE_CURVE('',#12175,#12173,#7066,.T.);
#15618=EDGE_CURVE('',#12175,#12176,#7067,.T.);
#15619=EDGE_CURVE('',#12176,#12174,#7068,.T.);
#15620=EDGE_CURVE('',#12166,#12175,#7069,.T.);
#15621=EDGE_CURVE('',#12168,#12176,#7070,.T.);
#15622=EDGE_CURVE('',#12177,#12177,#10001,.T.);
#15623=EDGE_CURVE('',#11889,#12177,#7071,.T.);
#15624=EDGE_CURVE('',#12178,#12178,#10002,.T.);
#15625=EDGE_CURVE('',#12178,#11941,#7072,.T.);
#21552=ORIENTED_EDGE('',*,*,#15184,.F.);
#21553=ORIENTED_EDGE('',*,*,#15185,.T.);
#21554=ORIENTED_EDGE('',*,*,#15186,.T.);
#21555=ORIENTED_EDGE('',*,*,#15187,.T.);
#21556=ORIENTED_EDGE('',*,*,#15188,.T.);
#21557=ORIENTED_EDGE('',*,*,#15187,.F.);
#21558=ORIENTED_EDGE('',*,*,#15189,.T.);
#21559=ORIENTED_EDGE('',*,*,#15190,.T.);
#21560=ORIENTED_EDGE('',*,*,#15191,.F.);
#21561=ORIENTED_EDGE('',*,*,#15192,.T.);
#21562=ORIENTED_EDGE('',*,*,#15184,.T.);
#21563=ORIENTED_EDGE('',*,*,#15193,.T.);
#21564=ORIENTED_EDGE('',*,*,#15194,.F.);
#21565=ORIENTED_EDGE('',*,*,#15195,.T.);
#21566=ORIENTED_EDGE('',*,*,#15191,.T.);
#21567=ORIENTED_EDGE('',*,*,#15196,.T.);
#21568=ORIENTED_EDGE('',*,*,#15197,.F.);
#21569=ORIENTED_EDGE('',*,*,#15198,.T.);
#21570=ORIENTED_EDGE('',*,*,#15194,.T.);
#21571=ORIENTED_EDGE('',*,*,#15199,.T.);
#21572=ORIENTED_EDGE('',*,*,#15200,.F.);
#21573=ORIENTED_EDGE('',*,*,#15201,.T.);
#21574=ORIENTED_EDGE('',*,*,#15197,.T.);
#21575=ORIENTED_EDGE('',*,*,#15202,.T.);
#21576=ORIENTED_EDGE('',*,*,#15203,.F.);
#21577=ORIENTED_EDGE('',*,*,#15204,.T.);
#21578=ORIENTED_EDGE('',*,*,#15200,.T.);
#21579=ORIENTED_EDGE('',*,*,#15205,.T.);
#21580=ORIENTED_EDGE('',*,*,#15206,.F.);
#21581=ORIENTED_EDGE('',*,*,#15207,.T.);
#21582=ORIENTED_EDGE('',*,*,#15203,.T.);
#21583=ORIENTED_EDGE('',*,*,#15208,.T.);
#21584=ORIENTED_EDGE('',*,*,#15209,.F.);
#21585=ORIENTED_EDGE('',*,*,#15210,.T.);
#21586=ORIENTED_EDGE('',*,*,#15206,.T.);
#21587=ORIENTED_EDGE('',*,*,#15211,.T.);
#21588=ORIENTED_EDGE('',*,*,#15212,.F.);
#21589=ORIENTED_EDGE('',*,*,#15213,.T.);
#21590=ORIENTED_EDGE('',*,*,#15209,.T.);
#21591=ORIENTED_EDGE('',*,*,#15214,.T.);
#21592=ORIENTED_EDGE('',*,*,#15215,.F.);
#21593=ORIENTED_EDGE('',*,*,#15216,.T.);
#21594=ORIENTED_EDGE('',*,*,#15212,.T.);
#21595=ORIENTED_EDGE('',*,*,#15217,.T.);
#21596=ORIENTED_EDGE('',*,*,#15218,.F.);
#21597=ORIENTED_EDGE('',*,*,#15219,.T.);
#21598=ORIENTED_EDGE('',*,*,#15215,.T.);
#21599=ORIENTED_EDGE('',*,*,#15220,.T.);
#21600=ORIENTED_EDGE('',*,*,#15221,.F.);
#21601=ORIENTED_EDGE('',*,*,#15222,.T.);
#21602=ORIENTED_EDGE('',*,*,#15218,.T.);
#21603=ORIENTED_EDGE('',*,*,#15223,.T.);
#21604=ORIENTED_EDGE('',*,*,#15224,.F.);
#21605=ORIENTED_EDGE('',*,*,#15225,.T.);
#21606=ORIENTED_EDGE('',*,*,#15226,.F.);
#21607=ORIENTED_EDGE('',*,*,#15227,.F.);
#21608=ORIENTED_EDGE('',*,*,#15228,.F.);
#21609=ORIENTED_EDGE('',*,*,#15229,.T.);
#21610=ORIENTED_EDGE('',*,*,#15224,.T.);
#21611=ORIENTED_EDGE('',*,*,#15230,.F.);
#21612=ORIENTED_EDGE('',*,*,#15231,.F.);
#21613=ORIENTED_EDGE('',*,*,#15232,.T.);
#21614=ORIENTED_EDGE('',*,*,#15228,.T.);
#21615=ORIENTED_EDGE('',*,*,#15233,.F.);
#21616=ORIENTED_EDGE('',*,*,#15234,.F.);
#21617=ORIENTED_EDGE('',*,*,#15235,.T.);
#21618=ORIENTED_EDGE('',*,*,#15231,.T.);
#21619=ORIENTED_EDGE('',*,*,#15236,.F.);
#21620=ORIENTED_EDGE('',*,*,#15237,.F.);
#21621=ORIENTED_EDGE('',*,*,#15238,.T.);
#21622=ORIENTED_EDGE('',*,*,#15234,.T.);
#21623=ORIENTED_EDGE('',*,*,#15239,.F.);
#21624=ORIENTED_EDGE('',*,*,#15240,.F.);
#21625=ORIENTED_EDGE('',*,*,#15241,.T.);
#21626=ORIENTED_EDGE('',*,*,#15237,.T.);
#21627=ORIENTED_EDGE('',*,*,#15242,.F.);
#21628=ORIENTED_EDGE('',*,*,#15243,.F.);
#21629=ORIENTED_EDGE('',*,*,#15244,.T.);
#21630=ORIENTED_EDGE('',*,*,#15240,.T.);
#21631=ORIENTED_EDGE('',*,*,#15245,.F.);
#21632=ORIENTED_EDGE('',*,*,#15246,.F.);
#21633=ORIENTED_EDGE('',*,*,#15247,.T.);
#21634=ORIENTED_EDGE('',*,*,#15243,.T.);
#21635=ORIENTED_EDGE('',*,*,#15248,.F.);
#21636=ORIENTED_EDGE('',*,*,#15249,.F.);
#21637=ORIENTED_EDGE('',*,*,#15250,.T.);
#21638=ORIENTED_EDGE('',*,*,#15246,.T.);
#21639=ORIENTED_EDGE('',*,*,#15251,.F.);
#21640=ORIENTED_EDGE('',*,*,#15252,.F.);
#21641=ORIENTED_EDGE('',*,*,#15253,.T.);
#21642=ORIENTED_EDGE('',*,*,#15249,.T.);
#21643=ORIENTED_EDGE('',*,*,#15254,.F.);
#21644=ORIENTED_EDGE('',*,*,#15255,.F.);
#21645=ORIENTED_EDGE('',*,*,#15256,.T.);
#21646=ORIENTED_EDGE('',*,*,#15252,.T.);
#21647=ORIENTED_EDGE('',*,*,#15257,.F.);
#21648=ORIENTED_EDGE('',*,*,#15258,.F.);
#21649=ORIENTED_EDGE('',*,*,#15259,.F.);
#21650=ORIENTED_EDGE('',*,*,#15260,.T.);
#21651=ORIENTED_EDGE('',*,*,#15255,.T.);
#21652=ORIENTED_EDGE('',*,*,#15261,.F.);
#21653=ORIENTED_EDGE('',*,*,#15226,.T.);
#21654=ORIENTED_EDGE('',*,*,#15262,.T.);
#21655=ORIENTED_EDGE('',*,*,#15263,.F.);
#21656=ORIENTED_EDGE('',*,*,#15264,.F.);
#21657=ORIENTED_EDGE('',*,*,#15265,.T.);
#21658=ORIENTED_EDGE('',*,*,#15265,.F.);
#21659=ORIENTED_EDGE('',*,*,#15266,.F.);
#21660=ORIENTED_EDGE('',*,*,#15223,.F.);
#21661=ORIENTED_EDGE('',*,*,#15220,.F.);
#21662=ORIENTED_EDGE('',*,*,#15217,.F.);
#21663=ORIENTED_EDGE('',*,*,#15214,.F.);
#21664=ORIENTED_EDGE('',*,*,#15211,.F.);
#21665=ORIENTED_EDGE('',*,*,#15208,.F.);
#21666=ORIENTED_EDGE('',*,*,#15205,.F.);
#21667=ORIENTED_EDGE('',*,*,#15202,.F.);
#21668=ORIENTED_EDGE('',*,*,#15199,.F.);
#21669=ORIENTED_EDGE('',*,*,#15196,.F.);
#21670=ORIENTED_EDGE('',*,*,#15193,.F.);
#21671=ORIENTED_EDGE('',*,*,#15190,.F.);
#21672=ORIENTED_EDGE('',*,*,#15267,.F.);
#21673=ORIENTED_EDGE('',*,*,#15268,.T.);
#21674=ORIENTED_EDGE('',*,*,#15261,.T.);
#21675=ORIENTED_EDGE('',*,*,#15257,.T.);
#21676=ORIENTED_EDGE('',*,*,#15254,.T.);
#21677=ORIENTED_EDGE('',*,*,#15251,.T.);
#21678=ORIENTED_EDGE('',*,*,#15248,.T.);
#21679=ORIENTED_EDGE('',*,*,#15245,.T.);
#21680=ORIENTED_EDGE('',*,*,#15242,.T.);
#21681=ORIENTED_EDGE('',*,*,#15239,.T.);
#21682=ORIENTED_EDGE('',*,*,#15236,.T.);
#21683=ORIENTED_EDGE('',*,*,#15233,.T.);
#21684=ORIENTED_EDGE('',*,*,#15230,.T.);
#21685=ORIENTED_EDGE('',*,*,#15227,.T.);
#21686=ORIENTED_EDGE('',*,*,#15186,.F.);
#21687=ORIENTED_EDGE('',*,*,#15269,.T.);
#21688=ORIENTED_EDGE('',*,*,#15259,.T.);
#21689=ORIENTED_EDGE('',*,*,#15270,.T.);
#21690=ORIENTED_EDGE('',*,*,#15267,.T.);
#21691=ORIENTED_EDGE('',*,*,#15189,.F.);
#21692=ORIENTED_EDGE('',*,*,#15258,.T.);
#21693=ORIENTED_EDGE('',*,*,#15268,.F.);
#21694=ORIENTED_EDGE('',*,*,#15270,.F.);
#21695=ORIENTED_EDGE('',*,*,#15262,.F.);
#21696=ORIENTED_EDGE('',*,*,#15225,.F.);
#21697=ORIENTED_EDGE('',*,*,#15229,.F.);
#21698=ORIENTED_EDGE('',*,*,#15232,.F.);
#21699=ORIENTED_EDGE('',*,*,#15235,.F.);
#21700=ORIENTED_EDGE('',*,*,#15238,.F.);
#21701=ORIENTED_EDGE('',*,*,#15241,.F.);
#21702=ORIENTED_EDGE('',*,*,#15244,.F.);
#21703=ORIENTED_EDGE('',*,*,#15247,.F.);
#21704=ORIENTED_EDGE('',*,*,#15250,.F.);
#21705=ORIENTED_EDGE('',*,*,#15253,.F.);
#21706=ORIENTED_EDGE('',*,*,#15256,.F.);
#21707=ORIENTED_EDGE('',*,*,#15260,.F.);
#21708=ORIENTED_EDGE('',*,*,#15269,.F.);
#21709=ORIENTED_EDGE('',*,*,#15185,.F.);
#21710=ORIENTED_EDGE('',*,*,#15192,.F.);
#21711=ORIENTED_EDGE('',*,*,#15195,.F.);
#21712=ORIENTED_EDGE('',*,*,#15198,.F.);
#21713=ORIENTED_EDGE('',*,*,#15201,.F.);
#21714=ORIENTED_EDGE('',*,*,#15204,.F.);
#21715=ORIENTED_EDGE('',*,*,#15207,.F.);
#21716=ORIENTED_EDGE('',*,*,#15210,.F.);
#21717=ORIENTED_EDGE('',*,*,#15213,.F.);
#21718=ORIENTED_EDGE('',*,*,#15216,.F.);
#21719=ORIENTED_EDGE('',*,*,#15219,.F.);
#21720=ORIENTED_EDGE('',*,*,#15222,.F.);
#21721=ORIENTED_EDGE('',*,*,#15271,.F.);
#21722=ORIENTED_EDGE('',*,*,#15221,.T.);
#21723=ORIENTED_EDGE('',*,*,#15266,.T.);
#21724=ORIENTED_EDGE('',*,*,#15272,.F.);
#21725=ORIENTED_EDGE('',*,*,#15271,.T.);
#21726=ORIENTED_EDGE('',*,*,#15273,.F.);
#21727=ORIENTED_EDGE('',*,*,#15274,.T.);
#21728=ORIENTED_EDGE('',*,*,#15275,.T.);
#21729=ORIENTED_EDGE('',*,*,#15276,.F.);
#21730=ORIENTED_EDGE('',*,*,#15275,.F.);
#21731=ORIENTED_EDGE('',*,*,#15277,.T.);
#21732=ORIENTED_EDGE('',*,*,#15278,.F.);
#21733=ORIENTED_EDGE('',*,*,#15279,.F.);
#21734=ORIENTED_EDGE('',*,*,#15280,.F.);
#21735=ORIENTED_EDGE('',*,*,#15277,.F.);
#21736=ORIENTED_EDGE('',*,*,#15274,.F.);
#21737=ORIENTED_EDGE('',*,*,#15281,.F.);
#21738=ORIENTED_EDGE('',*,*,#15282,.T.);
#21739=ORIENTED_EDGE('',*,*,#15283,.T.);
#21740=ORIENTED_EDGE('',*,*,#15284,.F.);
#21741=ORIENTED_EDGE('',*,*,#15283,.F.);
#21742=ORIENTED_EDGE('',*,*,#15285,.T.);
#21743=ORIENTED_EDGE('',*,*,#15286,.F.);
#21744=ORIENTED_EDGE('',*,*,#15287,.F.);
#21745=ORIENTED_EDGE('',*,*,#15288,.F.);
#21746=ORIENTED_EDGE('',*,*,#15285,.F.);
#21747=ORIENTED_EDGE('',*,*,#15282,.F.);
#21748=ORIENTED_EDGE('',*,*,#15289,.F.);
#21749=ORIENTED_EDGE('',*,*,#15290,.T.);
#21750=ORIENTED_EDGE('',*,*,#15291,.T.);
#21751=ORIENTED_EDGE('',*,*,#15292,.F.);
#21752=ORIENTED_EDGE('',*,*,#15291,.F.);
#21753=ORIENTED_EDGE('',*,*,#15293,.T.);
#21754=ORIENTED_EDGE('',*,*,#15294,.F.);
#21755=ORIENTED_EDGE('',*,*,#15295,.F.);
#21756=ORIENTED_EDGE('',*,*,#15296,.F.);
#21757=ORIENTED_EDGE('',*,*,#15293,.F.);
#21758=ORIENTED_EDGE('',*,*,#15290,.F.);
#21759=ORIENTED_EDGE('',*,*,#15297,.F.);
#21760=ORIENTED_EDGE('',*,*,#15298,.T.);
#21761=ORIENTED_EDGE('',*,*,#15299,.T.);
#21762=ORIENTED_EDGE('',*,*,#15300,.F.);
#21763=ORIENTED_EDGE('',*,*,#15299,.F.);
#21764=ORIENTED_EDGE('',*,*,#15301,.T.);
#21765=ORIENTED_EDGE('',*,*,#15302,.F.);
#21766=ORIENTED_EDGE('',*,*,#15303,.F.);
#21767=ORIENTED_EDGE('',*,*,#15304,.F.);
#21768=ORIENTED_EDGE('',*,*,#15301,.F.);
#21769=ORIENTED_EDGE('',*,*,#15298,.F.);
#21770=ORIENTED_EDGE('',*,*,#15305,.F.);
#21771=ORIENTED_EDGE('',*,*,#15306,.T.);
#21772=ORIENTED_EDGE('',*,*,#15307,.T.);
#21773=ORIENTED_EDGE('',*,*,#15308,.F.);
#21774=ORIENTED_EDGE('',*,*,#15307,.F.);
#21775=ORIENTED_EDGE('',*,*,#15309,.T.);
#21776=ORIENTED_EDGE('',*,*,#15310,.F.);
#21777=ORIENTED_EDGE('',*,*,#15311,.F.);
#21778=ORIENTED_EDGE('',*,*,#15312,.F.);
#21779=ORIENTED_EDGE('',*,*,#15309,.F.);
#21780=ORIENTED_EDGE('',*,*,#15306,.F.);
#21781=ORIENTED_EDGE('',*,*,#15313,.F.);
#21782=ORIENTED_EDGE('',*,*,#15314,.T.);
#21783=ORIENTED_EDGE('',*,*,#15315,.T.);
#21784=ORIENTED_EDGE('',*,*,#15316,.F.);
#21785=ORIENTED_EDGE('',*,*,#15315,.F.);
#21786=ORIENTED_EDGE('',*,*,#15317,.T.);
#21787=ORIENTED_EDGE('',*,*,#15318,.F.);
#21788=ORIENTED_EDGE('',*,*,#15319,.F.);
#21789=ORIENTED_EDGE('',*,*,#15320,.F.);
#21790=ORIENTED_EDGE('',*,*,#15317,.F.);
#21791=ORIENTED_EDGE('',*,*,#15314,.F.);
#21792=ORIENTED_EDGE('',*,*,#15321,.F.);
#21793=ORIENTED_EDGE('',*,*,#15322,.T.);
#21794=ORIENTED_EDGE('',*,*,#15323,.T.);
#21795=ORIENTED_EDGE('',*,*,#15324,.F.);
#21796=ORIENTED_EDGE('',*,*,#15323,.F.);
#21797=ORIENTED_EDGE('',*,*,#15325,.T.);
#21798=ORIENTED_EDGE('',*,*,#15326,.F.);
#21799=ORIENTED_EDGE('',*,*,#15327,.F.);
#21800=ORIENTED_EDGE('',*,*,#15328,.F.);
#21801=ORIENTED_EDGE('',*,*,#15325,.F.);
#21802=ORIENTED_EDGE('',*,*,#15322,.F.);
#21803=ORIENTED_EDGE('',*,*,#15329,.F.);
#21804=ORIENTED_EDGE('',*,*,#15330,.T.);
#21805=ORIENTED_EDGE('',*,*,#15331,.T.);
#21806=ORIENTED_EDGE('',*,*,#15332,.F.);
#21807=ORIENTED_EDGE('',*,*,#15331,.F.);
#21808=ORIENTED_EDGE('',*,*,#15333,.T.);
#21809=ORIENTED_EDGE('',*,*,#15334,.F.);
#21810=ORIENTED_EDGE('',*,*,#15335,.F.);
#21811=ORIENTED_EDGE('',*,*,#15336,.F.);
#21812=ORIENTED_EDGE('',*,*,#15333,.F.);
#21813=ORIENTED_EDGE('',*,*,#15330,.F.);
#21814=ORIENTED_EDGE('',*,*,#15337,.F.);
#21815=ORIENTED_EDGE('',*,*,#15338,.T.);
#21816=ORIENTED_EDGE('',*,*,#15339,.T.);
#21817=ORIENTED_EDGE('',*,*,#15340,.F.);
#21818=ORIENTED_EDGE('',*,*,#15339,.F.);
#21819=ORIENTED_EDGE('',*,*,#15341,.T.);
#21820=ORIENTED_EDGE('',*,*,#15342,.F.);
#21821=ORIENTED_EDGE('',*,*,#15343,.F.);
#21822=ORIENTED_EDGE('',*,*,#15344,.F.);
#21823=ORIENTED_EDGE('',*,*,#15341,.F.);
#21824=ORIENTED_EDGE('',*,*,#15338,.F.);
#21825=ORIENTED_EDGE('',*,*,#15345,.F.);
#21826=ORIENTED_EDGE('',*,*,#15346,.T.);
#21827=ORIENTED_EDGE('',*,*,#15347,.T.);
#21828=ORIENTED_EDGE('',*,*,#15348,.F.);
#21829=ORIENTED_EDGE('',*,*,#15347,.F.);
#21830=ORIENTED_EDGE('',*,*,#15349,.T.);
#21831=ORIENTED_EDGE('',*,*,#15350,.F.);
#21832=ORIENTED_EDGE('',*,*,#15351,.F.);
#21833=ORIENTED_EDGE('',*,*,#15352,.F.);
#21834=ORIENTED_EDGE('',*,*,#15349,.F.);
#21835=ORIENTED_EDGE('',*,*,#15346,.F.);
#21836=ORIENTED_EDGE('',*,*,#15353,.F.);
#21837=ORIENTED_EDGE('',*,*,#15354,.T.);
#21838=ORIENTED_EDGE('',*,*,#15355,.T.);
#21839=ORIENTED_EDGE('',*,*,#15356,.F.);
#21840=ORIENTED_EDGE('',*,*,#15355,.F.);
#21841=ORIENTED_EDGE('',*,*,#15357,.T.);
#21842=ORIENTED_EDGE('',*,*,#15358,.F.);
#21843=ORIENTED_EDGE('',*,*,#15359,.F.);
#21844=ORIENTED_EDGE('',*,*,#15360,.F.);
#21845=ORIENTED_EDGE('',*,*,#15357,.F.);
#21846=ORIENTED_EDGE('',*,*,#15354,.F.);
#21847=ORIENTED_EDGE('',*,*,#15361,.F.);
#21848=ORIENTED_EDGE('',*,*,#15362,.T.);
#21849=ORIENTED_EDGE('',*,*,#15363,.T.);
#21850=ORIENTED_EDGE('',*,*,#15364,.F.);
#21851=ORIENTED_EDGE('',*,*,#15363,.F.);
#21852=ORIENTED_EDGE('',*,*,#15365,.T.);
#21853=ORIENTED_EDGE('',*,*,#15366,.F.);
#21854=ORIENTED_EDGE('',*,*,#15367,.F.);
#21855=ORIENTED_EDGE('',*,*,#15368,.F.);
#21856=ORIENTED_EDGE('',*,*,#15365,.F.);
#21857=ORIENTED_EDGE('',*,*,#15362,.F.);
#21858=ORIENTED_EDGE('',*,*,#15369,.F.);
#21859=ORIENTED_EDGE('',*,*,#15370,.T.);
#21860=ORIENTED_EDGE('',*,*,#15371,.T.);
#21861=ORIENTED_EDGE('',*,*,#15372,.F.);
#21862=ORIENTED_EDGE('',*,*,#15371,.F.);
#21863=ORIENTED_EDGE('',*,*,#15373,.T.);
#21864=ORIENTED_EDGE('',*,*,#15374,.F.);
#21865=ORIENTED_EDGE('',*,*,#15375,.F.);
#21866=ORIENTED_EDGE('',*,*,#15376,.F.);
#21867=ORIENTED_EDGE('',*,*,#15373,.F.);
#21868=ORIENTED_EDGE('',*,*,#15370,.F.);
#21869=ORIENTED_EDGE('',*,*,#15377,.F.);
#21870=ORIENTED_EDGE('',*,*,#15378,.T.);
#21871=ORIENTED_EDGE('',*,*,#15379,.T.);
#21872=ORIENTED_EDGE('',*,*,#15380,.F.);
#21873=ORIENTED_EDGE('',*,*,#15379,.F.);
#21874=ORIENTED_EDGE('',*,*,#15381,.T.);
#21875=ORIENTED_EDGE('',*,*,#15382,.F.);
#21876=ORIENTED_EDGE('',*,*,#15383,.F.);
#21877=ORIENTED_EDGE('',*,*,#15384,.F.);
#21878=ORIENTED_EDGE('',*,*,#15381,.F.);
#21879=ORIENTED_EDGE('',*,*,#15378,.F.);
#21880=ORIENTED_EDGE('',*,*,#15385,.F.);
#21881=ORIENTED_EDGE('',*,*,#15386,.T.);
#21882=ORIENTED_EDGE('',*,*,#15387,.T.);
#21883=ORIENTED_EDGE('',*,*,#15388,.F.);
#21884=ORIENTED_EDGE('',*,*,#15387,.F.);
#21885=ORIENTED_EDGE('',*,*,#15389,.T.);
#21886=ORIENTED_EDGE('',*,*,#15390,.F.);
#21887=ORIENTED_EDGE('',*,*,#15391,.F.);
#21888=ORIENTED_EDGE('',*,*,#15392,.F.);
#21889=ORIENTED_EDGE('',*,*,#15389,.F.);
#21890=ORIENTED_EDGE('',*,*,#15386,.F.);
#21891=ORIENTED_EDGE('',*,*,#15393,.F.);
#21892=ORIENTED_EDGE('',*,*,#15394,.T.);
#21893=ORIENTED_EDGE('',*,*,#15395,.T.);
#21894=ORIENTED_EDGE('',*,*,#15396,.F.);
#21895=ORIENTED_EDGE('',*,*,#15395,.F.);
#21896=ORIENTED_EDGE('',*,*,#15397,.T.);
#21897=ORIENTED_EDGE('',*,*,#15398,.F.);
#21898=ORIENTED_EDGE('',*,*,#15399,.F.);
#21899=ORIENTED_EDGE('',*,*,#15400,.F.);
#21900=ORIENTED_EDGE('',*,*,#15397,.F.);
#21901=ORIENTED_EDGE('',*,*,#15394,.F.);
#21902=ORIENTED_EDGE('',*,*,#15401,.F.);
#21903=ORIENTED_EDGE('',*,*,#15402,.T.);
#21904=ORIENTED_EDGE('',*,*,#15403,.T.);
#21905=ORIENTED_EDGE('',*,*,#15404,.F.);
#21906=ORIENTED_EDGE('',*,*,#15403,.F.);
#21907=ORIENTED_EDGE('',*,*,#15405,.T.);
#21908=ORIENTED_EDGE('',*,*,#15406,.F.);
#21909=ORIENTED_EDGE('',*,*,#15407,.F.);
#21910=ORIENTED_EDGE('',*,*,#15408,.F.);
#21911=ORIENTED_EDGE('',*,*,#15405,.F.);
#21912=ORIENTED_EDGE('',*,*,#15402,.F.);
#21913=ORIENTED_EDGE('',*,*,#15409,.F.);
#21914=ORIENTED_EDGE('',*,*,#15410,.T.);
#21915=ORIENTED_EDGE('',*,*,#15411,.T.);
#21916=ORIENTED_EDGE('',*,*,#15412,.F.);
#21917=ORIENTED_EDGE('',*,*,#15413,.F.);
#21918=ORIENTED_EDGE('',*,*,#15411,.F.);
#21919=ORIENTED_EDGE('',*,*,#15414,.T.);
#21920=ORIENTED_EDGE('',*,*,#15415,.F.);
#21921=ORIENTED_EDGE('',*,*,#15416,.F.);
#21922=ORIENTED_EDGE('',*,*,#15417,.F.);
#21923=ORIENTED_EDGE('',*,*,#15414,.F.);
#21924=ORIENTED_EDGE('',*,*,#15410,.F.);
#21925=ORIENTED_EDGE('',*,*,#15418,.F.);
#21926=ORIENTED_EDGE('',*,*,#15419,.T.);
#21927=ORIENTED_EDGE('',*,*,#15420,.T.);
#21928=ORIENTED_EDGE('',*,*,#15421,.F.);
#21929=ORIENTED_EDGE('',*,*,#15420,.F.);
#21930=ORIENTED_EDGE('',*,*,#15422,.T.);
#21931=ORIENTED_EDGE('',*,*,#15423,.F.);
#21932=ORIENTED_EDGE('',*,*,#15424,.F.);
#21933=ORIENTED_EDGE('',*,*,#15425,.F.);
#21934=ORIENTED_EDGE('',*,*,#15422,.F.);
#21935=ORIENTED_EDGE('',*,*,#15419,.F.);
#21936=ORIENTED_EDGE('',*,*,#15426,.F.);
#21937=ORIENTED_EDGE('',*,*,#15427,.T.);
#21938=ORIENTED_EDGE('',*,*,#15428,.T.);
#21939=ORIENTED_EDGE('',*,*,#15429,.F.);
#21940=ORIENTED_EDGE('',*,*,#15428,.F.);
#21941=ORIENTED_EDGE('',*,*,#15430,.T.);
#21942=ORIENTED_EDGE('',*,*,#15431,.F.);
#21943=ORIENTED_EDGE('',*,*,#15432,.F.);
#21944=ORIENTED_EDGE('',*,*,#15433,.F.);
#21945=ORIENTED_EDGE('',*,*,#15430,.F.);
#21946=ORIENTED_EDGE('',*,*,#15427,.F.);
#21947=ORIENTED_EDGE('',*,*,#15434,.F.);
#21948=ORIENTED_EDGE('',*,*,#15435,.T.);
#21949=ORIENTED_EDGE('',*,*,#15436,.T.);
#21950=ORIENTED_EDGE('',*,*,#15437,.F.);
#21951=ORIENTED_EDGE('',*,*,#15436,.F.);
#21952=ORIENTED_EDGE('',*,*,#15438,.T.);
#21953=ORIENTED_EDGE('',*,*,#15439,.F.);
#21954=ORIENTED_EDGE('',*,*,#15440,.F.);
#21955=ORIENTED_EDGE('',*,*,#15441,.F.);
#21956=ORIENTED_EDGE('',*,*,#15438,.F.);
#21957=ORIENTED_EDGE('',*,*,#15435,.F.);
#21958=ORIENTED_EDGE('',*,*,#15442,.F.);
#21959=ORIENTED_EDGE('',*,*,#15443,.T.);
#21960=ORIENTED_EDGE('',*,*,#15444,.T.);
#21961=ORIENTED_EDGE('',*,*,#15445,.F.);
#21962=ORIENTED_EDGE('',*,*,#15444,.F.);
#21963=ORIENTED_EDGE('',*,*,#15446,.T.);
#21964=ORIENTED_EDGE('',*,*,#15447,.F.);
#21965=ORIENTED_EDGE('',*,*,#15448,.F.);
#21966=ORIENTED_EDGE('',*,*,#15449,.F.);
#21967=ORIENTED_EDGE('',*,*,#15446,.F.);
#21968=ORIENTED_EDGE('',*,*,#15443,.F.);
#21969=ORIENTED_EDGE('',*,*,#15450,.F.);
#21970=ORIENTED_EDGE('',*,*,#15451,.T.);
#21971=ORIENTED_EDGE('',*,*,#15452,.T.);
#21972=ORIENTED_EDGE('',*,*,#15453,.F.);
#21973=ORIENTED_EDGE('',*,*,#15452,.F.);
#21974=ORIENTED_EDGE('',*,*,#15454,.T.);
#21975=ORIENTED_EDGE('',*,*,#15455,.F.);
#21976=ORIENTED_EDGE('',*,*,#15456,.F.);
#21977=ORIENTED_EDGE('',*,*,#15457,.F.);
#21978=ORIENTED_EDGE('',*,*,#15454,.F.);
#21979=ORIENTED_EDGE('',*,*,#15451,.F.);
#21980=ORIENTED_EDGE('',*,*,#15458,.F.);
#21981=ORIENTED_EDGE('',*,*,#15459,.T.);
#21982=ORIENTED_EDGE('',*,*,#15460,.T.);
#21983=ORIENTED_EDGE('',*,*,#15461,.F.);
#21984=ORIENTED_EDGE('',*,*,#15460,.F.);
#21985=ORIENTED_EDGE('',*,*,#15462,.T.);
#21986=ORIENTED_EDGE('',*,*,#15463,.F.);
#21987=ORIENTED_EDGE('',*,*,#15464,.F.);
#21988=ORIENTED_EDGE('',*,*,#15465,.F.);
#21989=ORIENTED_EDGE('',*,*,#15462,.F.);
#21990=ORIENTED_EDGE('',*,*,#15459,.F.);
#21991=ORIENTED_EDGE('',*,*,#15466,.F.);
#21992=ORIENTED_EDGE('',*,*,#15467,.T.);
#21993=ORIENTED_EDGE('',*,*,#15468,.T.);
#21994=ORIENTED_EDGE('',*,*,#15469,.F.);
#21995=ORIENTED_EDGE('',*,*,#15468,.F.);
#21996=ORIENTED_EDGE('',*,*,#15470,.T.);
#21997=ORIENTED_EDGE('',*,*,#15471,.F.);
#21998=ORIENTED_EDGE('',*,*,#15472,.F.);
#21999=ORIENTED_EDGE('',*,*,#15473,.F.);
#22000=ORIENTED_EDGE('',*,*,#15470,.F.);
#22001=ORIENTED_EDGE('',*,*,#15467,.F.);
#22002=ORIENTED_EDGE('',*,*,#15474,.F.);
#22003=ORIENTED_EDGE('',*,*,#15475,.T.);
#22004=ORIENTED_EDGE('',*,*,#15476,.T.);
#22005=ORIENTED_EDGE('',*,*,#15477,.F.);
#22006=ORIENTED_EDGE('',*,*,#15476,.F.);
#22007=ORIENTED_EDGE('',*,*,#15478,.T.);
#22008=ORIENTED_EDGE('',*,*,#15479,.F.);
#22009=ORIENTED_EDGE('',*,*,#15480,.F.);
#22010=ORIENTED_EDGE('',*,*,#15481,.F.);
#22011=ORIENTED_EDGE('',*,*,#15478,.F.);
#22012=ORIENTED_EDGE('',*,*,#15475,.F.);
#22013=ORIENTED_EDGE('',*,*,#15482,.F.);
#22014=ORIENTED_EDGE('',*,*,#15483,.T.);
#22015=ORIENTED_EDGE('',*,*,#15484,.T.);
#22016=ORIENTED_EDGE('',*,*,#15485,.F.);
#22017=ORIENTED_EDGE('',*,*,#15484,.F.);
#22018=ORIENTED_EDGE('',*,*,#15486,.T.);
#22019=ORIENTED_EDGE('',*,*,#15487,.F.);
#22020=ORIENTED_EDGE('',*,*,#15488,.F.);
#22021=ORIENTED_EDGE('',*,*,#15489,.F.);
#22022=ORIENTED_EDGE('',*,*,#15486,.F.);
#22023=ORIENTED_EDGE('',*,*,#15483,.F.);
#22024=ORIENTED_EDGE('',*,*,#15490,.F.);
#22025=ORIENTED_EDGE('',*,*,#15491,.T.);
#22026=ORIENTED_EDGE('',*,*,#15492,.T.);
#22027=ORIENTED_EDGE('',*,*,#15493,.F.);
#22028=ORIENTED_EDGE('',*,*,#15492,.F.);
#22029=ORIENTED_EDGE('',*,*,#15494,.T.);
#22030=ORIENTED_EDGE('',*,*,#15495,.F.);
#22031=ORIENTED_EDGE('',*,*,#15496,.F.);
#22032=ORIENTED_EDGE('',*,*,#15497,.F.);
#22033=ORIENTED_EDGE('',*,*,#15494,.F.);
#22034=ORIENTED_EDGE('',*,*,#15491,.F.);
#22035=ORIENTED_EDGE('',*,*,#15498,.F.);
#22036=ORIENTED_EDGE('',*,*,#15499,.T.);
#22037=ORIENTED_EDGE('',*,*,#15500,.T.);
#22038=ORIENTED_EDGE('',*,*,#15501,.F.);
#22039=ORIENTED_EDGE('',*,*,#15500,.F.);
#22040=ORIENTED_EDGE('',*,*,#15502,.T.);
#22041=ORIENTED_EDGE('',*,*,#15503,.F.);
#22042=ORIENTED_EDGE('',*,*,#15504,.F.);
#22043=ORIENTED_EDGE('',*,*,#15505,.F.);
#22044=ORIENTED_EDGE('',*,*,#15502,.F.);
#22045=ORIENTED_EDGE('',*,*,#15499,.F.);
#22046=ORIENTED_EDGE('',*,*,#15506,.F.);
#22047=ORIENTED_EDGE('',*,*,#15507,.T.);
#22048=ORIENTED_EDGE('',*,*,#15508,.T.);
#22049=ORIENTED_EDGE('',*,*,#15509,.F.);
#22050=ORIENTED_EDGE('',*,*,#15508,.F.);
#22051=ORIENTED_EDGE('',*,*,#15510,.T.);
#22052=ORIENTED_EDGE('',*,*,#15511,.F.);
#22053=ORIENTED_EDGE('',*,*,#15512,.F.);
#22054=ORIENTED_EDGE('',*,*,#15513,.F.);
#22055=ORIENTED_EDGE('',*,*,#15510,.F.);
#22056=ORIENTED_EDGE('',*,*,#15507,.F.);
#22057=ORIENTED_EDGE('',*,*,#15514,.F.);
#22058=ORIENTED_EDGE('',*,*,#15515,.T.);
#22059=ORIENTED_EDGE('',*,*,#15516,.T.);
#22060=ORIENTED_EDGE('',*,*,#15517,.F.);
#22061=ORIENTED_EDGE('',*,*,#15516,.F.);
#22062=ORIENTED_EDGE('',*,*,#15518,.T.);
#22063=ORIENTED_EDGE('',*,*,#15519,.F.);
#22064=ORIENTED_EDGE('',*,*,#15520,.F.);
#22065=ORIENTED_EDGE('',*,*,#15521,.F.);
#22066=ORIENTED_EDGE('',*,*,#15518,.F.);
#22067=ORIENTED_EDGE('',*,*,#15515,.F.);
#22068=ORIENTED_EDGE('',*,*,#15522,.F.);
#22069=ORIENTED_EDGE('',*,*,#15523,.T.);
#22070=ORIENTED_EDGE('',*,*,#15524,.T.);
#22071=ORIENTED_EDGE('',*,*,#15525,.F.);
#22072=ORIENTED_EDGE('',*,*,#15524,.F.);
#22073=ORIENTED_EDGE('',*,*,#15526,.T.);
#22074=ORIENTED_EDGE('',*,*,#15527,.F.);
#22075=ORIENTED_EDGE('',*,*,#15528,.F.);
#22076=ORIENTED_EDGE('',*,*,#15529,.F.);
#22077=ORIENTED_EDGE('',*,*,#15526,.F.);
#22078=ORIENTED_EDGE('',*,*,#15523,.F.);
#22079=ORIENTED_EDGE('',*,*,#15530,.F.);
#22080=ORIENTED_EDGE('',*,*,#15531,.T.);
#22081=ORIENTED_EDGE('',*,*,#15532,.T.);
#22082=ORIENTED_EDGE('',*,*,#15533,.F.);
#22083=ORIENTED_EDGE('',*,*,#15532,.F.);
#22084=ORIENTED_EDGE('',*,*,#15534,.T.);
#22085=ORIENTED_EDGE('',*,*,#15535,.F.);
#22086=ORIENTED_EDGE('',*,*,#15536,.F.);
#22087=ORIENTED_EDGE('',*,*,#15537,.F.);
#22088=ORIENTED_EDGE('',*,*,#15534,.F.);
#22089=ORIENTED_EDGE('',*,*,#15531,.F.);
#22090=ORIENTED_EDGE('',*,*,#15538,.F.);
#22091=ORIENTED_EDGE('',*,*,#15539,.T.);
#22092=ORIENTED_EDGE('',*,*,#15540,.T.);
#22093=ORIENTED_EDGE('',*,*,#15541,.F.);
#22094=ORIENTED_EDGE('',*,*,#15540,.F.);
#22095=ORIENTED_EDGE('',*,*,#15542,.T.);
#22096=ORIENTED_EDGE('',*,*,#15543,.F.);
#22097=ORIENTED_EDGE('',*,*,#15544,.F.);
#22098=ORIENTED_EDGE('',*,*,#15545,.F.);
#22099=ORIENTED_EDGE('',*,*,#15542,.F.);
#22100=ORIENTED_EDGE('',*,*,#15539,.F.);
#22101=ORIENTED_EDGE('',*,*,#15546,.F.);
#22102=ORIENTED_EDGE('',*,*,#15547,.T.);
#22103=ORIENTED_EDGE('',*,*,#15548,.T.);
#22104=ORIENTED_EDGE('',*,*,#15549,.F.);
#22105=ORIENTED_EDGE('',*,*,#15548,.F.);
#22106=ORIENTED_EDGE('',*,*,#15550,.T.);
#22107=ORIENTED_EDGE('',*,*,#15551,.F.);
#22108=ORIENTED_EDGE('',*,*,#15552,.F.);
#22109=ORIENTED_EDGE('',*,*,#15553,.F.);
#22110=ORIENTED_EDGE('',*,*,#15550,.F.);
#22111=ORIENTED_EDGE('',*,*,#15547,.F.);
#22112=ORIENTED_EDGE('',*,*,#15279,.T.);
#22113=ORIENTED_EDGE('',*,*,#15273,.T.);
#22114=ORIENTED_EDGE('',*,*,#15276,.T.);
#22115=ORIENTED_EDGE('',*,*,#15554,.F.);
#22116=ORIENTED_EDGE('',*,*,#15287,.T.);
#22117=ORIENTED_EDGE('',*,*,#15281,.T.);
#22118=ORIENTED_EDGE('',*,*,#15284,.T.);
#22119=ORIENTED_EDGE('',*,*,#15555,.F.);
#22120=ORIENTED_EDGE('',*,*,#15295,.T.);
#22121=ORIENTED_EDGE('',*,*,#15289,.T.);
#22122=ORIENTED_EDGE('',*,*,#15292,.T.);
#22123=ORIENTED_EDGE('',*,*,#15556,.F.);
#22124=ORIENTED_EDGE('',*,*,#15303,.T.);
#22125=ORIENTED_EDGE('',*,*,#15297,.T.);
#22126=ORIENTED_EDGE('',*,*,#15300,.T.);
#22127=ORIENTED_EDGE('',*,*,#15557,.F.);
#22128=ORIENTED_EDGE('',*,*,#15311,.T.);
#22129=ORIENTED_EDGE('',*,*,#15305,.T.);
#22130=ORIENTED_EDGE('',*,*,#15308,.T.);
#22131=ORIENTED_EDGE('',*,*,#15558,.F.);
#22132=ORIENTED_EDGE('',*,*,#15319,.T.);
#22133=ORIENTED_EDGE('',*,*,#15313,.T.);
#22134=ORIENTED_EDGE('',*,*,#15316,.T.);
#22135=ORIENTED_EDGE('',*,*,#15559,.F.);
#22136=ORIENTED_EDGE('',*,*,#15327,.T.);
#22137=ORIENTED_EDGE('',*,*,#15321,.T.);
#22138=ORIENTED_EDGE('',*,*,#15324,.T.);
#22139=ORIENTED_EDGE('',*,*,#15560,.F.);
#22140=ORIENTED_EDGE('',*,*,#15335,.T.);
#22141=ORIENTED_EDGE('',*,*,#15329,.T.);
#22142=ORIENTED_EDGE('',*,*,#15332,.T.);
#22143=ORIENTED_EDGE('',*,*,#15561,.F.);
#22144=ORIENTED_EDGE('',*,*,#15343,.T.);
#22145=ORIENTED_EDGE('',*,*,#15337,.T.);
#22146=ORIENTED_EDGE('',*,*,#15340,.T.);
#22147=ORIENTED_EDGE('',*,*,#15562,.F.);
#22148=ORIENTED_EDGE('',*,*,#15351,.T.);
#22149=ORIENTED_EDGE('',*,*,#15345,.T.);
#22150=ORIENTED_EDGE('',*,*,#15348,.T.);
#22151=ORIENTED_EDGE('',*,*,#15563,.F.);
#22152=ORIENTED_EDGE('',*,*,#15359,.T.);
#22153=ORIENTED_EDGE('',*,*,#15353,.T.);
#22154=ORIENTED_EDGE('',*,*,#15356,.T.);
#22155=ORIENTED_EDGE('',*,*,#15564,.F.);
#22156=ORIENTED_EDGE('',*,*,#15367,.T.);
#22157=ORIENTED_EDGE('',*,*,#15361,.T.);
#22158=ORIENTED_EDGE('',*,*,#15364,.T.);
#22159=ORIENTED_EDGE('',*,*,#15565,.F.);
#22160=ORIENTED_EDGE('',*,*,#15375,.T.);
#22161=ORIENTED_EDGE('',*,*,#15369,.T.);
#22162=ORIENTED_EDGE('',*,*,#15372,.T.);
#22163=ORIENTED_EDGE('',*,*,#15566,.F.);
#22164=ORIENTED_EDGE('',*,*,#15383,.T.);
#22165=ORIENTED_EDGE('',*,*,#15377,.T.);
#22166=ORIENTED_EDGE('',*,*,#15380,.T.);
#22167=ORIENTED_EDGE('',*,*,#15567,.F.);
#22168=ORIENTED_EDGE('',*,*,#15391,.T.);
#22169=ORIENTED_EDGE('',*,*,#15385,.T.);
#22170=ORIENTED_EDGE('',*,*,#15388,.T.);
#22171=ORIENTED_EDGE('',*,*,#15568,.F.);
#22172=ORIENTED_EDGE('',*,*,#15399,.T.);
#22173=ORIENTED_EDGE('',*,*,#15393,.T.);
#22174=ORIENTED_EDGE('',*,*,#15396,.T.);
#22175=ORIENTED_EDGE('',*,*,#15569,.F.);
#22176=ORIENTED_EDGE('',*,*,#15407,.T.);
#22177=ORIENTED_EDGE('',*,*,#15401,.T.);
#22178=ORIENTED_EDGE('',*,*,#15404,.T.);
#22179=ORIENTED_EDGE('',*,*,#15570,.F.);
#22180=ORIENTED_EDGE('',*,*,#15416,.T.);
#22181=ORIENTED_EDGE('',*,*,#15409,.T.);
#22182=ORIENTED_EDGE('',*,*,#15571,.T.);
#22183=ORIENTED_EDGE('',*,*,#15572,.T.);
#22184=ORIENTED_EDGE('',*,*,#15571,.F.);
#22185=ORIENTED_EDGE('',*,*,#15412,.T.);
#22186=ORIENTED_EDGE('',*,*,#15413,.T.);
#22187=ORIENTED_EDGE('',*,*,#15573,.F.);
#22188=ORIENTED_EDGE('',*,*,#15424,.T.);
#22189=ORIENTED_EDGE('',*,*,#15418,.T.);
#22190=ORIENTED_EDGE('',*,*,#15421,.T.);
#22191=ORIENTED_EDGE('',*,*,#15574,.F.);
#22192=ORIENTED_EDGE('',*,*,#15432,.T.);
#22193=ORIENTED_EDGE('',*,*,#15426,.T.);
#22194=ORIENTED_EDGE('',*,*,#15429,.T.);
#22195=ORIENTED_EDGE('',*,*,#15575,.F.);
#22196=ORIENTED_EDGE('',*,*,#15440,.T.);
#22197=ORIENTED_EDGE('',*,*,#15434,.T.);
#22198=ORIENTED_EDGE('',*,*,#15437,.T.);
#22199=ORIENTED_EDGE('',*,*,#15576,.F.);
#22200=ORIENTED_EDGE('',*,*,#15448,.T.);
#22201=ORIENTED_EDGE('',*,*,#15442,.T.);
#22202=ORIENTED_EDGE('',*,*,#15445,.T.);
#22203=ORIENTED_EDGE('',*,*,#15577,.F.);
#22204=ORIENTED_EDGE('',*,*,#15456,.T.);
#22205=ORIENTED_EDGE('',*,*,#15450,.T.);
#22206=ORIENTED_EDGE('',*,*,#15453,.T.);
#22207=ORIENTED_EDGE('',*,*,#15578,.F.);
#22208=ORIENTED_EDGE('',*,*,#15464,.T.);
#22209=ORIENTED_EDGE('',*,*,#15458,.T.);
#22210=ORIENTED_EDGE('',*,*,#15461,.T.);
#22211=ORIENTED_EDGE('',*,*,#15579,.F.);
#22212=ORIENTED_EDGE('',*,*,#15472,.T.);
#22213=ORIENTED_EDGE('',*,*,#15466,.T.);
#22214=ORIENTED_EDGE('',*,*,#15469,.T.);
#22215=ORIENTED_EDGE('',*,*,#15580,.F.);
#22216=ORIENTED_EDGE('',*,*,#15480,.T.);
#22217=ORIENTED_EDGE('',*,*,#15474,.T.);
#22218=ORIENTED_EDGE('',*,*,#15477,.T.);
#22219=ORIENTED_EDGE('',*,*,#15581,.F.);
#22220=ORIENTED_EDGE('',*,*,#15488,.T.);
#22221=ORIENTED_EDGE('',*,*,#15482,.T.);
#22222=ORIENTED_EDGE('',*,*,#15485,.T.);
#22223=ORIENTED_EDGE('',*,*,#15582,.F.);
#22224=ORIENTED_EDGE('',*,*,#15496,.T.);
#22225=ORIENTED_EDGE('',*,*,#15490,.T.);
#22226=ORIENTED_EDGE('',*,*,#15493,.T.);
#22227=ORIENTED_EDGE('',*,*,#15583,.F.);
#22228=ORIENTED_EDGE('',*,*,#15504,.T.);
#22229=ORIENTED_EDGE('',*,*,#15498,.T.);
#22230=ORIENTED_EDGE('',*,*,#15501,.T.);
#22231=ORIENTED_EDGE('',*,*,#15584,.F.);
#22232=ORIENTED_EDGE('',*,*,#15512,.T.);
#22233=ORIENTED_EDGE('',*,*,#15506,.T.);
#22234=ORIENTED_EDGE('',*,*,#15509,.T.);
#22235=ORIENTED_EDGE('',*,*,#15585,.F.);
#22236=ORIENTED_EDGE('',*,*,#15520,.T.);
#22237=ORIENTED_EDGE('',*,*,#15514,.T.);
#22238=ORIENTED_EDGE('',*,*,#15517,.T.);
#22239=ORIENTED_EDGE('',*,*,#15586,.F.);
#22240=ORIENTED_EDGE('',*,*,#15528,.T.);
#22241=ORIENTED_EDGE('',*,*,#15522,.T.);
#22242=ORIENTED_EDGE('',*,*,#15525,.T.);
#22243=ORIENTED_EDGE('',*,*,#15587,.F.);
#22244=ORIENTED_EDGE('',*,*,#15536,.T.);
#22245=ORIENTED_EDGE('',*,*,#15530,.T.);
#22246=ORIENTED_EDGE('',*,*,#15533,.T.);
#22247=ORIENTED_EDGE('',*,*,#15588,.F.);
#22248=ORIENTED_EDGE('',*,*,#15544,.T.);
#22249=ORIENTED_EDGE('',*,*,#15538,.T.);
#22250=ORIENTED_EDGE('',*,*,#15541,.T.);
#22251=ORIENTED_EDGE('',*,*,#15589,.F.);
#22252=ORIENTED_EDGE('',*,*,#15552,.T.);
#22253=ORIENTED_EDGE('',*,*,#15546,.T.);
#22254=ORIENTED_EDGE('',*,*,#15549,.T.);
#22255=ORIENTED_EDGE('',*,*,#15590,.F.);
#22256=ORIENTED_EDGE('',*,*,#15591,.T.);
#22257=ORIENTED_EDGE('',*,*,#15592,.T.);
#22258=ORIENTED_EDGE('',*,*,#15593,.T.);
#22259=ORIENTED_EDGE('',*,*,#15594,.F.);
#22260=ORIENTED_EDGE('',*,*,#15593,.F.);
#22261=ORIENTED_EDGE('',*,*,#15595,.F.);
#22262=ORIENTED_EDGE('',*,*,#15596,.T.);
#22263=ORIENTED_EDGE('',*,*,#15597,.F.);
#22264=ORIENTED_EDGE('',*,*,#15598,.F.);
#22265=ORIENTED_EDGE('',*,*,#15596,.F.);
#22266=ORIENTED_EDGE('',*,*,#15599,.F.);
#22267=ORIENTED_EDGE('',*,*,#15591,.F.);
#22268=ORIENTED_EDGE('',*,*,#15592,.F.);
#22269=ORIENTED_EDGE('',*,*,#15599,.T.);
#22270=ORIENTED_EDGE('',*,*,#15595,.T.);
#22271=ORIENTED_EDGE('',*,*,#15600,.F.);
#22272=ORIENTED_EDGE('',*,*,#15601,.T.);
#22273=ORIENTED_EDGE('',*,*,#15417,.T.);
#22274=ORIENTED_EDGE('',*,*,#15570,.T.);
#22275=ORIENTED_EDGE('',*,*,#15406,.T.);
#22276=ORIENTED_EDGE('',*,*,#15408,.T.);
#22277=ORIENTED_EDGE('',*,*,#15569,.T.);
#22278=ORIENTED_EDGE('',*,*,#15398,.T.);
#22279=ORIENTED_EDGE('',*,*,#15400,.T.);
#22280=ORIENTED_EDGE('',*,*,#15568,.T.);
#22281=ORIENTED_EDGE('',*,*,#15390,.T.);
#22282=ORIENTED_EDGE('',*,*,#15392,.T.);
#22283=ORIENTED_EDGE('',*,*,#15567,.T.);
#22284=ORIENTED_EDGE('',*,*,#15382,.T.);
#22285=ORIENTED_EDGE('',*,*,#15384,.T.);
#22286=ORIENTED_EDGE('',*,*,#15566,.T.);
#22287=ORIENTED_EDGE('',*,*,#15374,.T.);
#22288=ORIENTED_EDGE('',*,*,#15376,.T.);
#22289=ORIENTED_EDGE('',*,*,#15565,.T.);
#22290=ORIENTED_EDGE('',*,*,#15366,.T.);
#22291=ORIENTED_EDGE('',*,*,#15368,.T.);
#22292=ORIENTED_EDGE('',*,*,#15564,.T.);
#22293=ORIENTED_EDGE('',*,*,#15358,.T.);
#22294=ORIENTED_EDGE('',*,*,#15360,.T.);
#22295=ORIENTED_EDGE('',*,*,#15563,.T.);
#22296=ORIENTED_EDGE('',*,*,#15350,.T.);
#22297=ORIENTED_EDGE('',*,*,#15352,.T.);
#22298=ORIENTED_EDGE('',*,*,#15562,.T.);
#22299=ORIENTED_EDGE('',*,*,#15342,.T.);
#22300=ORIENTED_EDGE('',*,*,#15344,.T.);
#22301=ORIENTED_EDGE('',*,*,#15561,.T.);
#22302=ORIENTED_EDGE('',*,*,#15334,.T.);
#22303=ORIENTED_EDGE('',*,*,#15336,.T.);
#22304=ORIENTED_EDGE('',*,*,#15560,.T.);
#22305=ORIENTED_EDGE('',*,*,#15326,.T.);
#22306=ORIENTED_EDGE('',*,*,#15328,.T.);
#22307=ORIENTED_EDGE('',*,*,#15559,.T.);
#22308=ORIENTED_EDGE('',*,*,#15318,.T.);
#22309=ORIENTED_EDGE('',*,*,#15320,.T.);
#22310=ORIENTED_EDGE('',*,*,#15558,.T.);
#22311=ORIENTED_EDGE('',*,*,#15310,.T.);
#22312=ORIENTED_EDGE('',*,*,#15312,.T.);
#22313=ORIENTED_EDGE('',*,*,#15557,.T.);
#22314=ORIENTED_EDGE('',*,*,#15302,.T.);
#22315=ORIENTED_EDGE('',*,*,#15304,.T.);
#22316=ORIENTED_EDGE('',*,*,#15556,.T.);
#22317=ORIENTED_EDGE('',*,*,#15294,.T.);
#22318=ORIENTED_EDGE('',*,*,#15296,.T.);
#22319=ORIENTED_EDGE('',*,*,#15555,.T.);
#22320=ORIENTED_EDGE('',*,*,#15286,.T.);
#22321=ORIENTED_EDGE('',*,*,#15288,.T.);
#22322=ORIENTED_EDGE('',*,*,#15554,.T.);
#22323=ORIENTED_EDGE('',*,*,#15278,.T.);
#22324=ORIENTED_EDGE('',*,*,#15280,.T.);
#22325=ORIENTED_EDGE('',*,*,#15594,.T.);
#22326=ORIENTED_EDGE('',*,*,#15597,.T.);
#22327=ORIENTED_EDGE('',*,*,#15598,.T.);
#22328=ORIENTED_EDGE('',*,*,#15590,.T.);
#22329=ORIENTED_EDGE('',*,*,#15551,.T.);
#22330=ORIENTED_EDGE('',*,*,#15553,.T.);
#22331=ORIENTED_EDGE('',*,*,#15589,.T.);
#22332=ORIENTED_EDGE('',*,*,#15543,.T.);
#22333=ORIENTED_EDGE('',*,*,#15545,.T.);
#22334=ORIENTED_EDGE('',*,*,#15588,.T.);
#22335=ORIENTED_EDGE('',*,*,#15535,.T.);
#22336=ORIENTED_EDGE('',*,*,#15537,.T.);
#22337=ORIENTED_EDGE('',*,*,#15587,.T.);
#22338=ORIENTED_EDGE('',*,*,#15527,.T.);
#22339=ORIENTED_EDGE('',*,*,#15529,.T.);
#22340=ORIENTED_EDGE('',*,*,#15586,.T.);
#22341=ORIENTED_EDGE('',*,*,#15519,.T.);
#22342=ORIENTED_EDGE('',*,*,#15521,.T.);
#22343=ORIENTED_EDGE('',*,*,#15585,.T.);
#22344=ORIENTED_EDGE('',*,*,#15511,.T.);
#22345=ORIENTED_EDGE('',*,*,#15513,.T.);
#22346=ORIENTED_EDGE('',*,*,#15584,.T.);
#22347=ORIENTED_EDGE('',*,*,#15503,.T.);
#22348=ORIENTED_EDGE('',*,*,#15505,.T.);
#22349=ORIENTED_EDGE('',*,*,#15583,.T.);
#22350=ORIENTED_EDGE('',*,*,#15495,.T.);
#22351=ORIENTED_EDGE('',*,*,#15497,.T.);
#22352=ORIENTED_EDGE('',*,*,#15582,.T.);
#22353=ORIENTED_EDGE('',*,*,#15487,.T.);
#22354=ORIENTED_EDGE('',*,*,#15489,.T.);
#22355=ORIENTED_EDGE('',*,*,#15581,.T.);
#22356=ORIENTED_EDGE('',*,*,#15479,.T.);
#22357=ORIENTED_EDGE('',*,*,#15481,.T.);
#22358=ORIENTED_EDGE('',*,*,#15580,.T.);
#22359=ORIENTED_EDGE('',*,*,#15471,.T.);
#22360=ORIENTED_EDGE('',*,*,#15473,.T.);
#22361=ORIENTED_EDGE('',*,*,#15579,.T.);
#22362=ORIENTED_EDGE('',*,*,#15463,.T.);
#22363=ORIENTED_EDGE('',*,*,#15465,.T.);
#22364=ORIENTED_EDGE('',*,*,#15578,.T.);
#22365=ORIENTED_EDGE('',*,*,#15455,.T.);
#22366=ORIENTED_EDGE('',*,*,#15457,.T.);
#22367=ORIENTED_EDGE('',*,*,#15577,.T.);
#22368=ORIENTED_EDGE('',*,*,#15447,.T.);
#22369=ORIENTED_EDGE('',*,*,#15449,.T.);
#22370=ORIENTED_EDGE('',*,*,#15576,.T.);
#22371=ORIENTED_EDGE('',*,*,#15439,.T.);
#22372=ORIENTED_EDGE('',*,*,#15441,.T.);
#22373=ORIENTED_EDGE('',*,*,#15575,.T.);
#22374=ORIENTED_EDGE('',*,*,#15431,.T.);
#22375=ORIENTED_EDGE('',*,*,#15433,.T.);
#22376=ORIENTED_EDGE('',*,*,#15574,.T.);
#22377=ORIENTED_EDGE('',*,*,#15423,.T.);
#22378=ORIENTED_EDGE('',*,*,#15425,.T.);
#22379=ORIENTED_EDGE('',*,*,#15573,.T.);
#22380=ORIENTED_EDGE('',*,*,#15415,.T.);
#22381=ORIENTED_EDGE('',*,*,#15601,.F.);
#22382=ORIENTED_EDGE('',*,*,#15602,.T.);
#22383=ORIENTED_EDGE('',*,*,#15603,.F.);
#22384=ORIENTED_EDGE('',*,*,#15602,.F.);
#22385=ORIENTED_EDGE('',*,*,#15604,.F.);
#22386=ORIENTED_EDGE('',*,*,#15605,.T.);
#22387=ORIENTED_EDGE('',*,*,#15606,.T.);
#22388=ORIENTED_EDGE('',*,*,#15607,.F.);
#22389=ORIENTED_EDGE('',*,*,#15608,.F.);
#22390=ORIENTED_EDGE('',*,*,#15609,.T.);
#22391=ORIENTED_EDGE('',*,*,#15610,.T.);
#22392=ORIENTED_EDGE('',*,*,#15605,.F.);
#22393=ORIENTED_EDGE('',*,*,#15611,.F.);
#22394=ORIENTED_EDGE('',*,*,#15612,.T.);
#22395=ORIENTED_EDGE('',*,*,#15613,.T.);
#22396=ORIENTED_EDGE('',*,*,#15609,.F.);
#22397=ORIENTED_EDGE('',*,*,#15614,.F.);
#22398=ORIENTED_EDGE('',*,*,#15615,.T.);
#22399=ORIENTED_EDGE('',*,*,#15616,.T.);
#22400=ORIENTED_EDGE('',*,*,#15612,.F.);
#22401=ORIENTED_EDGE('',*,*,#15617,.F.);
#22402=ORIENTED_EDGE('',*,*,#15618,.T.);
#22403=ORIENTED_EDGE('',*,*,#15619,.T.);
#22404=ORIENTED_EDGE('',*,*,#15615,.F.);
#22405=ORIENTED_EDGE('',*,*,#15620,.F.);
#22406=ORIENTED_EDGE('',*,*,#15607,.T.);
#22407=ORIENTED_EDGE('',*,*,#15621,.T.);
#22408=ORIENTED_EDGE('',*,*,#15618,.F.);
#22409=ORIENTED_EDGE('',*,*,#15621,.F.);
#22410=ORIENTED_EDGE('',*,*,#15606,.F.);
#22411=ORIENTED_EDGE('',*,*,#15610,.F.);
#22412=ORIENTED_EDGE('',*,*,#15613,.F.);
#22413=ORIENTED_EDGE('',*,*,#15616,.F.);
#22414=ORIENTED_EDGE('',*,*,#15619,.F.);
#22415=ORIENTED_EDGE('',*,*,#15603,.T.);
#22416=ORIENTED_EDGE('',*,*,#15622,.F.);
#22417=ORIENTED_EDGE('',*,*,#15188,.F.);
#22418=ORIENTED_EDGE('',*,*,#15623,.T.);
#22419=ORIENTED_EDGE('',*,*,#15622,.T.);
#22420=ORIENTED_EDGE('',*,*,#15623,.F.);
#22421=ORIENTED_EDGE('',*,*,#15624,.F.);
#22422=ORIENTED_EDGE('',*,*,#15625,.T.);
#22423=ORIENTED_EDGE('',*,*,#15263,.T.);
#22424=ORIENTED_EDGE('',*,*,#15272,.T.);
#22425=ORIENTED_EDGE('',*,*,#15264,.T.);
#22426=ORIENTED_EDGE('',*,*,#15625,.F.);
#22427=ORIENTED_EDGE('',*,*,#15572,.F.);
#22428=ORIENTED_EDGE('',*,*,#15624,.T.);
#22429=ORIENTED_EDGE('',*,*,#15600,.T.);
#22430=ORIENTED_EDGE('',*,*,#15604,.T.);
#22431=ORIENTED_EDGE('',*,*,#15620,.T.);
#22432=ORIENTED_EDGE('',*,*,#15617,.T.);
#22433=ORIENTED_EDGE('',*,*,#15614,.T.);
#22434=ORIENTED_EDGE('',*,*,#15611,.T.);
#22435=ORIENTED_EDGE('',*,*,#15608,.T.);
#23157=CONICAL_SURFACE('',#27007,0.2175,0.785398163397448);
#23158=CONICAL_SURFACE('',#27009,0.0461880215351701,1.00445035903315);
#23159=CONICAL_SURFACE('',#27020,0.11,0.78539816339745);
#23160=CONICAL_SURFACE('',#27021,0.13,0.785398163397449);
#24280=ADVANCED_FACE('',(#3527),#2331,.T.);
#24281=ADVANCED_FACE('',(#3528),#2332,.T.);
#24282=ADVANCED_FACE('',(#3529),#2333,.T.);
#24283=ADVANCED_FACE('',(#3530),#2334,.T.);
#24284=ADVANCED_FACE('',(#3531),#2335,.T.);
#24285=ADVANCED_FACE('',(#3532),#2336,.T.);
#24286=ADVANCED_FACE('',(#3533),#2337,.T.);
#24287=ADVANCED_FACE('',(#3534),#2338,.T.);
#24288=ADVANCED_FACE('',(#3535),#2339,.T.);
#24289=ADVANCED_FACE('',(#3536),#2340,.T.);
#24290=ADVANCED_FACE('',(#3537),#2341,.T.);
#24291=ADVANCED_FACE('',(#3538),#2342,.T.);
#24292=ADVANCED_FACE('',(#3539),#2343,.T.);
#24293=ADVANCED_FACE('',(#3540),#2344,.T.);
#24294=ADVANCED_FACE('',(#3541),#2345,.T.);
#24295=ADVANCED_FACE('',(#3542),#2346,.T.);
#24296=ADVANCED_FACE('',(#3543),#2347,.T.);
#24297=ADVANCED_FACE('',(#3544),#2348,.T.);
#24298=ADVANCED_FACE('',(#3545),#2349,.T.);
#24299=ADVANCED_FACE('',(#3546),#2350,.T.);
#24300=ADVANCED_FACE('',(#3547),#2351,.T.);
#24301=ADVANCED_FACE('',(#3548),#2352,.T.);
#24302=ADVANCED_FACE('',(#3549),#2353,.T.);
#24303=ADVANCED_FACE('',(#3550),#2354,.T.);
#24304=ADVANCED_FACE('',(#3551),#1798,.F.);
#24305=ADVANCED_FACE('',(#3552),#478,.F.);
#24306=ADVANCED_FACE('',(#3553),#1799,.T.);
#24307=ADVANCED_FACE('',(#3554),#2355,.T.);
#24308=ADVANCED_FACE('',(#3555),#479,.F.);
#24309=ADVANCED_FACE('',(#3556),#2356,.T.);
#24310=ADVANCED_FACE('',(#3557),#1800,.T.);
#24311=ADVANCED_FACE('',(#3558),#1801,.F.);
#24312=ADVANCED_FACE('',(#3559),#1802,.F.);
#24313=ADVANCED_FACE('',(#3560),#1803,.T.);
#24314=ADVANCED_FACE('',(#3561),#1804,.F.);
#24315=ADVANCED_FACE('',(#3562),#1805,.F.);
#24316=ADVANCED_FACE('',(#3563),#1806,.T.);
#24317=ADVANCED_FACE('',(#3564),#1807,.F.);
#24318=ADVANCED_FACE('',(#3565),#1808,.F.);
#24319=ADVANCED_FACE('',(#3566),#1809,.T.);
#24320=ADVANCED_FACE('',(#3567),#1810,.F.);
#24321=ADVANCED_FACE('',(#3568),#1811,.F.);
#24322=ADVANCED_FACE('',(#3569),#1812,.T.);
#24323=ADVANCED_FACE('',(#3570),#1813,.F.);
#24324=ADVANCED_FACE('',(#3571),#1814,.F.);
#24325=ADVANCED_FACE('',(#3572),#1815,.T.);
#24326=ADVANCED_FACE('',(#3573),#1816,.F.);
#24327=ADVANCED_FACE('',(#3574),#1817,.F.);
#24328=ADVANCED_FACE('',(#3575),#1818,.T.);
#24329=ADVANCED_FACE('',(#3576),#1819,.F.);
#24330=ADVANCED_FACE('',(#3577),#1820,.F.);
#24331=ADVANCED_FACE('',(#3578),#1821,.T.);
#24332=ADVANCED_FACE('',(#3579),#1822,.F.);
#24333=ADVANCED_FACE('',(#3580),#1823,.F.);
#24334=ADVANCED_FACE('',(#3581),#1824,.T.);
#24335=ADVANCED_FACE('',(#3582),#1825,.F.);
#24336=ADVANCED_FACE('',(#3583),#1826,.F.);
#24337=ADVANCED_FACE('',(#3584),#1827,.T.);
#24338=ADVANCED_FACE('',(#3585),#1828,.F.);
#24339=ADVANCED_FACE('',(#3586),#1829,.F.);
#24340=ADVANCED_FACE('',(#3587),#1830,.T.);
#24341=ADVANCED_FACE('',(#3588),#1831,.F.);
#24342=ADVANCED_FACE('',(#3589),#1832,.F.);
#24343=ADVANCED_FACE('',(#3590),#1833,.T.);
#24344=ADVANCED_FACE('',(#3591),#1834,.F.);
#24345=ADVANCED_FACE('',(#3592),#1835,.F.);
#24346=ADVANCED_FACE('',(#3593),#1836,.T.);
#24347=ADVANCED_FACE('',(#3594),#1837,.F.);
#24348=ADVANCED_FACE('',(#3595),#1838,.F.);
#24349=ADVANCED_FACE('',(#3596),#1839,.T.);
#24350=ADVANCED_FACE('',(#3597),#1840,.F.);
#24351=ADVANCED_FACE('',(#3598),#1841,.F.);
#24352=ADVANCED_FACE('',(#3599),#1842,.T.);
#24353=ADVANCED_FACE('',(#3600),#1843,.F.);
#24354=ADVANCED_FACE('',(#3601),#1844,.F.);
#24355=ADVANCED_FACE('',(#3602),#1845,.T.);
#24356=ADVANCED_FACE('',(#3603),#1846,.F.);
#24357=ADVANCED_FACE('',(#3604),#1847,.F.);
#24358=ADVANCED_FACE('',(#3605),#1848,.T.);
#24359=ADVANCED_FACE('',(#3606),#1849,.F.);
#24360=ADVANCED_FACE('',(#3607),#1850,.F.);
#24361=ADVANCED_FACE('',(#3608),#1851,.T.);
#24362=ADVANCED_FACE('',(#3609),#1852,.F.);
#24363=ADVANCED_FACE('',(#3610),#1853,.F.);
#24364=ADVANCED_FACE('',(#3611),#1854,.T.);
#24365=ADVANCED_FACE('',(#3612),#1855,.F.);
#24366=ADVANCED_FACE('',(#3613),#1856,.F.);
#24367=ADVANCED_FACE('',(#3614),#1857,.T.);
#24368=ADVANCED_FACE('',(#3615),#1858,.F.);
#24369=ADVANCED_FACE('',(#3616),#1859,.F.);
#24370=ADVANCED_FACE('',(#3617),#1860,.T.);
#24371=ADVANCED_FACE('',(#3618),#1861,.F.);
#24372=ADVANCED_FACE('',(#3619),#1862,.F.);
#24373=ADVANCED_FACE('',(#3620),#1863,.T.);
#24374=ADVANCED_FACE('',(#3621),#1864,.F.);
#24375=ADVANCED_FACE('',(#3622),#1865,.F.);
#24376=ADVANCED_FACE('',(#3623),#1866,.T.);
#24377=ADVANCED_FACE('',(#3624),#1867,.F.);
#24378=ADVANCED_FACE('',(#3625),#1868,.F.);
#24379=ADVANCED_FACE('',(#3626),#1869,.T.);
#24380=ADVANCED_FACE('',(#3627),#1870,.F.);
#24381=ADVANCED_FACE('',(#3628),#1871,.F.);
#24382=ADVANCED_FACE('',(#3629),#1872,.T.);
#24383=ADVANCED_FACE('',(#3630),#1873,.F.);
#24384=ADVANCED_FACE('',(#3631),#1874,.F.);
#24385=ADVANCED_FACE('',(#3632),#1875,.T.);
#24386=ADVANCED_FACE('',(#3633),#1876,.F.);
#24387=ADVANCED_FACE('',(#3634),#1877,.F.);
#24388=ADVANCED_FACE('',(#3635),#1878,.T.);
#24389=ADVANCED_FACE('',(#3636),#1879,.F.);
#24390=ADVANCED_FACE('',(#3637),#1880,.F.);
#24391=ADVANCED_FACE('',(#3638),#1881,.T.);
#24392=ADVANCED_FACE('',(#3639),#1882,.F.);
#24393=ADVANCED_FACE('',(#3640),#1883,.F.);
#24394=ADVANCED_FACE('',(#3641),#1884,.T.);
#24395=ADVANCED_FACE('',(#3642),#1885,.F.);
#24396=ADVANCED_FACE('',(#3643),#1886,.F.);
#24397=ADVANCED_FACE('',(#3644),#1887,.T.);
#24398=ADVANCED_FACE('',(#3645),#1888,.F.);
#24399=ADVANCED_FACE('',(#3646),#1889,.F.);
#24400=ADVANCED_FACE('',(#3647),#1890,.T.);
#24401=ADVANCED_FACE('',(#3648),#1891,.F.);
#24402=ADVANCED_FACE('',(#3649),#1892,.F.);
#24403=ADVANCED_FACE('',(#3650),#1893,.T.);
#24404=ADVANCED_FACE('',(#3651),#1894,.F.);
#24405=ADVANCED_FACE('',(#3652),#1895,.F.);
#24406=ADVANCED_FACE('',(#3653),#1896,.T.);
#24407=ADVANCED_FACE('',(#3654),#1897,.F.);
#24408=ADVANCED_FACE('',(#3655),#1898,.F.);
#24409=ADVANCED_FACE('',(#3656),#1899,.T.);
#24410=ADVANCED_FACE('',(#3657),#1900,.F.);
#24411=ADVANCED_FACE('',(#3658),#1901,.F.);
#24412=ADVANCED_FACE('',(#3659),#1902,.T.);
#24413=ADVANCED_FACE('',(#3660),#1903,.F.);
#24414=ADVANCED_FACE('',(#3661),#1904,.F.);
#24415=ADVANCED_FACE('',(#3662),#2357,.T.);
#24416=ADVANCED_FACE('',(#3663),#1905,.F.);
#24417=ADVANCED_FACE('',(#3664),#1906,.F.);
#24418=ADVANCED_FACE('',(#3665),#1907,.T.);
#24419=ADVANCED_FACE('',(#3666),#23157,.T.);
#24420=ADVANCED_FACE('',(#3667),#23158,.F.);
#24421=ADVANCED_FACE('',(#3668),#1908,.F.);
#24422=ADVANCED_FACE('',(#3669),#1909,.F.);
#24423=ADVANCED_FACE('',(#3670),#1910,.F.);
#24424=ADVANCED_FACE('',(#3671),#1911,.F.);
#24425=ADVANCED_FACE('',(#3672),#1912,.F.);
#24426=ADVANCED_FACE('',(#3673),#1913,.F.);
#24427=ADVANCED_FACE('',(#3674,#1269),#1914,.F.);
#24428=ADVANCED_FACE('',(#3675),#1915,.T.);
#24429=ADVANCED_FACE('',(#3676),#23159,.T.);
#24430=ADVANCED_FACE('',(#3677),#23160,.T.);
#24431=ADVANCED_FACE('',(#3678,#1270),#1916,.T.);
#24432=ADVANCED_FACE('',(#3679,#1271),#1917,.T.);
#24546=CLOSED_SHELL('',(#24280,#24281,#24282,#24283,#24284,#24285,#24286,
#24287,#24288,#24289,#24290,#24291,#24292,#24293,#24294,#24295,#24296,#24297,
#24298,#24299,#24300,#24301,#24302,#24303,#24304,#24305,#24306,#24307,#24308,
#24309,#24310,#24311,#24312,#24313,#24314,#24315,#24316,#24317,#24318,#24319,
#24320,#24321,#24322,#24323,#24324,#24325,#24326,#24327,#24328,#24329,#24330,
#24331,#24332,#24333,#24334,#24335,#24336,#24337,#24338,#24339,#24340,#24341,
#24342,#24343,#24344,#24345,#24346,#24347,#24348,#24349,#24350,#24351,#24352,
#24353,#24354,#24355,#24356,#24357,#24358,#24359,#24360,#24361,#24362,#24363,
#24364,#24365,#24366,#24367,#24368,#24369,#24370,#24371,#24372,#24373,#24374,
#24375,#24376,#24377,#24378,#24379,#24380,#24381,#24382,#24383,#24384,#24385,
#24386,#24387,#24388,#24389,#24390,#24391,#24392,#24393,#24394,#24395,#24396,
#24397,#24398,#24399,#24400,#24401,#24402,#24403,#24404,#24405,#24406,#24407,
#24408,#24409,#24410,#24411,#24412,#24413,#24414,#24415,#24416,#24417,#24418,
#24419,#24420,#24421,#24422,#24423,#24424,#24425,#24426,#24427,#24428,#24429,
#24430,#24431,#24432));
#26786=AXIS2_PLACEMENT_3D('',#48669,#32693,#32694);
#26787=AXIS2_PLACEMENT_3D('',#48670,#32695,#32696);
#26788=AXIS2_PLACEMENT_3D('',#48692,#32698,#32699);
#26789=AXIS2_PLACEMENT_3D('',#48695,#32701,#32702);
#26790=AXIS2_PLACEMENT_3D('',#48697,#32703,#32704);
#26791=AXIS2_PLACEMENT_3D('',#48711,#32705,#32706);
#26792=AXIS2_PLACEMENT_3D('',#48759,#32708,#32709);
#26793=AXIS2_PLACEMENT_3D('',#48807,#32711,#32712);
#26794=AXIS2_PLACEMENT_3D('',#48861,#32714,#32715);
#26795=AXIS2_PLACEMENT_3D('',#48909,#32717,#32718);
#26796=AXIS2_PLACEMENT_3D('',#48963,#32720,#32721);
#26797=AXIS2_PLACEMENT_3D('',#49011,#32723,#32724);
#26798=AXIS2_PLACEMENT_3D('',#49059,#32726,#32727);
#26799=AXIS2_PLACEMENT_3D('',#49113,#32729,#32730);
#26800=AXIS2_PLACEMENT_3D('',#49161,#32732,#32733);
#26801=AXIS2_PLACEMENT_3D('',#49209,#32735,#32736);
#26802=AXIS2_PLACEMENT_3D('',#49263,#32738,#32739);
#26803=AXIS2_PLACEMENT_3D('',#49278,#32741,#32742);
#26804=AXIS2_PLACEMENT_3D('',#49286,#32743,#32744);
#26805=AXIS2_PLACEMENT_3D('',#49311,#32746,#32747);
#26806=AXIS2_PLACEMENT_3D('',#49335,#32749,#32750);
#26807=AXIS2_PLACEMENT_3D('',#49360,#32752,#32753);
#26808=AXIS2_PLACEMENT_3D('',#49385,#32755,#32756);
#26809=AXIS2_PLACEMENT_3D('',#49409,#32758,#32759);
#26810=AXIS2_PLACEMENT_3D('',#49434,#32761,#32762);
#26811=AXIS2_PLACEMENT_3D('',#49459,#32764,#32765);
#26812=AXIS2_PLACEMENT_3D('',#49484,#32767,#32768);
#26813=AXIS2_PLACEMENT_3D('',#49509,#32770,#32771);
#26814=AXIS2_PLACEMENT_3D('',#49533,#32773,#32774);
#26815=AXIS2_PLACEMENT_3D('',#49538,#32776,#32777);
#26816=AXIS2_PLACEMENT_3D('',#49559,#32778,#32779);
#26817=AXIS2_PLACEMENT_3D('',#49611,#32780,#32781);
#26818=AXIS2_PLACEMENT_3D('',#49613,#32782,#32783);
#26819=AXIS2_PLACEMENT_3D('',#50045,#32784,#32785);
#26820=AXIS2_PLACEMENT_3D('',#50095,#32786,#32787);
#26821=AXIS2_PLACEMENT_3D('',#50096,#32788,#32789);
#26822=AXIS2_PLACEMENT_3D('',#50421,#32790,#32791);
#26823=AXIS2_PLACEMENT_3D('',#50422,#32792,#32793);
#26824=AXIS2_PLACEMENT_3D('',#50423,#32794,#32795);
#26825=AXIS2_PLACEMENT_3D('',#50426,#32796,#32797);
#26826=AXIS2_PLACEMENT_3D('',#50430,#32800,#32801);
#26827=AXIS2_PLACEMENT_3D('',#50438,#32804,#32805);
#26828=AXIS2_PLACEMENT_3D('',#50444,#32807,#32808);
#26829=AXIS2_PLACEMENT_3D('',#50447,#32809,#32810);
#26830=AXIS2_PLACEMENT_3D('',#50451,#32813,#32814);
#26831=AXIS2_PLACEMENT_3D('',#50459,#32817,#32818);
#26832=AXIS2_PLACEMENT_3D('',#50465,#32820,#32821);
#26833=AXIS2_PLACEMENT_3D('',#50468,#32822,#32823);
#26834=AXIS2_PLACEMENT_3D('',#50472,#32826,#32827);
#26835=AXIS2_PLACEMENT_3D('',#50480,#32830,#32831);
#26836=AXIS2_PLACEMENT_3D('',#50486,#32833,#32834);
#26837=AXIS2_PLACEMENT_3D('',#50489,#32835,#32836);
#26838=AXIS2_PLACEMENT_3D('',#50493,#32839,#32840);
#26839=AXIS2_PLACEMENT_3D('',#50501,#32843,#32844);
#26840=AXIS2_PLACEMENT_3D('',#50507,#32846,#32847);
#26841=AXIS2_PLACEMENT_3D('',#50510,#32848,#32849);
#26842=AXIS2_PLACEMENT_3D('',#50514,#32852,#32853);
#26843=AXIS2_PLACEMENT_3D('',#50522,#32856,#32857);
#26844=AXIS2_PLACEMENT_3D('',#50528,#32859,#32860);
#26845=AXIS2_PLACEMENT_3D('',#50531,#32861,#32862);
#26846=AXIS2_PLACEMENT_3D('',#50535,#32865,#32866);
#26847=AXIS2_PLACEMENT_3D('',#50543,#32869,#32870);
#26848=AXIS2_PLACEMENT_3D('',#50549,#32872,#32873);
#26849=AXIS2_PLACEMENT_3D('',#50552,#32874,#32875);
#26850=AXIS2_PLACEMENT_3D('',#50556,#32878,#32879);
#26851=AXIS2_PLACEMENT_3D('',#50564,#32882,#32883);
#26852=AXIS2_PLACEMENT_3D('',#50570,#32885,#32886);
#26853=AXIS2_PLACEMENT_3D('',#50573,#32887,#32888);
#26854=AXIS2_PLACEMENT_3D('',#50577,#32891,#32892);
#26855=AXIS2_PLACEMENT_3D('',#50585,#32895,#32896);
#26856=AXIS2_PLACEMENT_3D('',#50591,#32898,#32899);
#26857=AXIS2_PLACEMENT_3D('',#50594,#32900,#32901);
#26858=AXIS2_PLACEMENT_3D('',#50598,#32904,#32905);
#26859=AXIS2_PLACEMENT_3D('',#50606,#32908,#32909);
#26860=AXIS2_PLACEMENT_3D('',#50612,#32911,#32912);
#26861=AXIS2_PLACEMENT_3D('',#50615,#32913,#32914);
#26862=AXIS2_PLACEMENT_3D('',#50619,#32917,#32918);
#26863=AXIS2_PLACEMENT_3D('',#50627,#32921,#32922);
#26864=AXIS2_PLACEMENT_3D('',#50633,#32924,#32925);
#26865=AXIS2_PLACEMENT_3D('',#50636,#32926,#32927);
#26866=AXIS2_PLACEMENT_3D('',#50640,#32930,#32931);
#26867=AXIS2_PLACEMENT_3D('',#50648,#32934,#32935);
#26868=AXIS2_PLACEMENT_3D('',#50654,#32937,#32938);
#26869=AXIS2_PLACEMENT_3D('',#50657,#32939,#32940);
#26870=AXIS2_PLACEMENT_3D('',#50661,#32943,#32944);
#26871=AXIS2_PLACEMENT_3D('',#50669,#32947,#32948);
#26872=AXIS2_PLACEMENT_3D('',#50675,#32950,#32951);
#26873=AXIS2_PLACEMENT_3D('',#50678,#32952,#32953);
#26874=AXIS2_PLACEMENT_3D('',#50682,#32956,#32957);
#26875=AXIS2_PLACEMENT_3D('',#50690,#32960,#32961);
#26876=AXIS2_PLACEMENT_3D('',#50696,#32963,#32964);
#26877=AXIS2_PLACEMENT_3D('',#50699,#32965,#32966);
#26878=AXIS2_PLACEMENT_3D('',#50703,#32969,#32970);
#26879=AXIS2_PLACEMENT_3D('',#50711,#32973,#32974);
#26880=AXIS2_PLACEMENT_3D('',#50717,#32976,#32977);
#26881=AXIS2_PLACEMENT_3D('',#50720,#32978,#32979);
#26882=AXIS2_PLACEMENT_3D('',#50724,#32982,#32983);
#26883=AXIS2_PLACEMENT_3D('',#50732,#32986,#32987);
#26884=AXIS2_PLACEMENT_3D('',#50738,#32989,#32990);
#26885=AXIS2_PLACEMENT_3D('',#50741,#32991,#32992);
#26886=AXIS2_PLACEMENT_3D('',#50745,#32995,#32996);
#26887=AXIS2_PLACEMENT_3D('',#50753,#32999,#33000);
#26888=AXIS2_PLACEMENT_3D('',#50759,#33002,#33003);
#26889=AXIS2_PLACEMENT_3D('',#50762,#33004,#33005);
#26890=AXIS2_PLACEMENT_3D('',#50766,#33008,#33009);
#26891=AXIS2_PLACEMENT_3D('',#50774,#33012,#33013);
#26892=AXIS2_PLACEMENT_3D('',#50780,#33015,#33016);
#26893=AXIS2_PLACEMENT_3D('',#50783,#33017,#33018);
#26894=AXIS2_PLACEMENT_3D('',#50788,#33021,#33022);
#26895=AXIS2_PLACEMENT_3D('',#50789,#33023,#33024);
#26896=AXIS2_PLACEMENT_3D('',#50797,#33027,#33028);
#26897=AXIS2_PLACEMENT_3D('',#50803,#33030,#33031);
#26898=AXIS2_PLACEMENT_3D('',#50806,#33032,#33033);
#26899=AXIS2_PLACEMENT_3D('',#50810,#33036,#33037);
#26900=AXIS2_PLACEMENT_3D('',#50818,#33040,#33041);
#26901=AXIS2_PLACEMENT_3D('',#50824,#33043,#33044);
#26902=AXIS2_PLACEMENT_3D('',#50827,#33045,#33046);
#26903=AXIS2_PLACEMENT_3D('',#50831,#33049,#33050);
#26904=AXIS2_PLACEMENT_3D('',#50839,#33053,#33054);
#26905=AXIS2_PLACEMENT_3D('',#50845,#33056,#33057);
#26906=AXIS2_PLACEMENT_3D('',#50848,#33058,#33059);
#26907=AXIS2_PLACEMENT_3D('',#50852,#33062,#33063);
#26908=AXIS2_PLACEMENT_3D('',#50860,#33066,#33067);
#26909=AXIS2_PLACEMENT_3D('',#50866,#33069,#33070);
#26910=AXIS2_PLACEMENT_3D('',#50869,#33071,#33072);
#26911=AXIS2_PLACEMENT_3D('',#50873,#33075,#33076);
#26912=AXIS2_PLACEMENT_3D('',#50881,#33079,#33080);
#26913=AXIS2_PLACEMENT_3D('',#50887,#33082,#33083);
#26914=AXIS2_PLACEMENT_3D('',#50890,#33084,#33085);
#26915=AXIS2_PLACEMENT_3D('',#50894,#33088,#33089);
#26916=AXIS2_PLACEMENT_3D('',#50902,#33092,#33093);
#26917=AXIS2_PLACEMENT_3D('',#50908,#33095,#33096);
#26918=AXIS2_PLACEMENT_3D('',#50911,#33097,#33098);
#26919=AXIS2_PLACEMENT_3D('',#50915,#33101,#33102);
#26920=AXIS2_PLACEMENT_3D('',#50923,#33105,#33106);
#26921=AXIS2_PLACEMENT_3D('',#50929,#33108,#33109);
#26922=AXIS2_PLACEMENT_3D('',#50932,#33110,#33111);
#26923=AXIS2_PLACEMENT_3D('',#50936,#33114,#33115);
#26924=AXIS2_PLACEMENT_3D('',#50944,#33118,#33119);
#26925=AXIS2_PLACEMENT_3D('',#50950,#33121,#33122);
#26926=AXIS2_PLACEMENT_3D('',#50953,#33123,#33124);
#26927=AXIS2_PLACEMENT_3D('',#50957,#33127,#33128);
#26928=AXIS2_PLACEMENT_3D('',#50965,#33131,#33132);
#26929=AXIS2_PLACEMENT_3D('',#50971,#33134,#33135);
#26930=AXIS2_PLACEMENT_3D('',#50974,#33136,#33137);
#26931=AXIS2_PLACEMENT_3D('',#50978,#33140,#33141);
#26932=AXIS2_PLACEMENT_3D('',#50986,#33144,#33145);
#26933=AXIS2_PLACEMENT_3D('',#50992,#33147,#33148);
#26934=AXIS2_PLACEMENT_3D('',#50995,#33149,#33150);
#26935=AXIS2_PLACEMENT_3D('',#50999,#33153,#33154);
#26936=AXIS2_PLACEMENT_3D('',#51007,#33157,#33158);
#26937=AXIS2_PLACEMENT_3D('',#51013,#33160,#33161);
#26938=AXIS2_PLACEMENT_3D('',#51016,#33162,#33163);
#26939=AXIS2_PLACEMENT_3D('',#51020,#33166,#33167);
#26940=AXIS2_PLACEMENT_3D('',#51028,#33170,#33171);
#26941=AXIS2_PLACEMENT_3D('',#51034,#33173,#33174);
#26942=AXIS2_PLACEMENT_3D('',#51037,#33175,#33176);
#26943=AXIS2_PLACEMENT_3D('',#51041,#33179,#33180);
#26944=AXIS2_PLACEMENT_3D('',#51049,#33183,#33184);
#26945=AXIS2_PLACEMENT_3D('',#51055,#33186,#33187);
#26946=AXIS2_PLACEMENT_3D('',#51058,#33188,#33189);
#26947=AXIS2_PLACEMENT_3D('',#51062,#33192,#33193);
#26948=AXIS2_PLACEMENT_3D('',#51070,#33196,#33197);
#26949=AXIS2_PLACEMENT_3D('',#51076,#33199,#33200);
#26950=AXIS2_PLACEMENT_3D('',#51079,#33201,#33202);
#26951=AXIS2_PLACEMENT_3D('',#51083,#33205,#33206);
#26952=AXIS2_PLACEMENT_3D('',#51091,#33209,#33210);
#26953=AXIS2_PLACEMENT_3D('',#51097,#33212,#33213);
#26954=AXIS2_PLACEMENT_3D('',#51100,#33214,#33215);
#26955=AXIS2_PLACEMENT_3D('',#51104,#33218,#33219);
#26956=AXIS2_PLACEMENT_3D('',#51112,#33222,#33223);
#26957=AXIS2_PLACEMENT_3D('',#51118,#33225,#33226);
#26958=AXIS2_PLACEMENT_3D('',#51121,#33227,#33228);
#26959=AXIS2_PLACEMENT_3D('',#51125,#33231,#33232);
#26960=AXIS2_PLACEMENT_3D('',#51133,#33235,#33236);
#26961=AXIS2_PLACEMENT_3D('',#51139,#33238,#33239);
#26962=AXIS2_PLACEMENT_3D('',#51142,#33240,#33241);
#26963=AXIS2_PLACEMENT_3D('',#51146,#33244,#33245);
#26964=AXIS2_PLACEMENT_3D('',#51154,#33248,#33249);
#26965=AXIS2_PLACEMENT_3D('',#51160,#33251,#33252);
#26966=AXIS2_PLACEMENT_3D('',#51161,#33253,#33254);
#26967=AXIS2_PLACEMENT_3D('',#51162,#33255,#33256);
#26968=AXIS2_PLACEMENT_3D('',#51163,#33257,#33258);
#26969=AXIS2_PLACEMENT_3D('',#51164,#33259,#33260);
#26970=AXIS2_PLACEMENT_3D('',#51165,#33261,#33262);
#26971=AXIS2_PLACEMENT_3D('',#51166,#33263,#33264);
#26972=AXIS2_PLACEMENT_3D('',#51167,#33265,#33266);
#26973=AXIS2_PLACEMENT_3D('',#51168,#33267,#33268);
#26974=AXIS2_PLACEMENT_3D('',#51169,#33269,#33270);
#26975=AXIS2_PLACEMENT_3D('',#51170,#33271,#33272);
#26976=AXIS2_PLACEMENT_3D('',#51171,#33273,#33274);
#26977=AXIS2_PLACEMENT_3D('',#51172,#33275,#33276);
#26978=AXIS2_PLACEMENT_3D('',#51173,#33277,#33278);
#26979=AXIS2_PLACEMENT_3D('',#51174,#33279,#33280);
#26980=AXIS2_PLACEMENT_3D('',#51175,#33281,#33282);
#26981=AXIS2_PLACEMENT_3D('',#51176,#33283,#33284);
#26982=AXIS2_PLACEMENT_3D('',#51177,#33285,#33286);
#26983=AXIS2_PLACEMENT_3D('',#51180,#33288,#33289);
#26984=AXIS2_PLACEMENT_3D('',#51181,#33290,#33291);
#26985=AXIS2_PLACEMENT_3D('',#51182,#33292,#33293);
#26986=AXIS2_PLACEMENT_3D('',#51183,#33294,#33295);
#26987=AXIS2_PLACEMENT_3D('',#51184,#33296,#33297);
#26988=AXIS2_PLACEMENT_3D('',#51185,#33298,#33299);
#26989=AXIS2_PLACEMENT_3D('',#51186,#33300,#33301);
#26990=AXIS2_PLACEMENT_3D('',#51187,#33302,#33303);
#26991=AXIS2_PLACEMENT_3D('',#51188,#33304,#33305);
#26992=AXIS2_PLACEMENT_3D('',#51189,#33306,#33307);
#26993=AXIS2_PLACEMENT_3D('',#51190,#33308,#33309);
#26994=AXIS2_PLACEMENT_3D('',#51191,#33310,#33311);
#26995=AXIS2_PLACEMENT_3D('',#51192,#33312,#33313);
#26996=AXIS2_PLACEMENT_3D('',#51193,#33314,#33315);
#26997=AXIS2_PLACEMENT_3D('',#51194,#33316,#33317);
#26998=AXIS2_PLACEMENT_3D('',#51195,#33318,#33319);
#26999=AXIS2_PLACEMENT_3D('',#51196,#33320,#33321);
#27000=AXIS2_PLACEMENT_3D('',#51197,#33322,#33323);
#27001=AXIS2_PLACEMENT_3D('',#51199,#33324,#33325);
#27002=AXIS2_PLACEMENT_3D('',#51203,#33327,#33328);
#27003=AXIS2_PLACEMENT_3D('',#51206,#33330,#33331);
#27004=AXIS2_PLACEMENT_3D('',#51207,#33332,#33333);
#27005=AXIS2_PLACEMENT_3D('',#51215,#33336,#33337);
#27006=AXIS2_PLACEMENT_3D('',#51220,#33339,#33340);
#27007=AXIS2_PLACEMENT_3D('',#51221,#33341,#33342);
#27008=AXIS2_PLACEMENT_3D('',#51223,#33343,#33344);
#27009=AXIS2_PLACEMENT_3D('',#51225,#33346,#33347);
#27010=AXIS2_PLACEMENT_3D('',#51229,#33349,#33350);
#27011=AXIS2_PLACEMENT_3D('',#51230,#33351,#33352);
#27012=AXIS2_PLACEMENT_3D('',#51239,#33357,#33358);
#27013=AXIS2_PLACEMENT_3D('',#51245,#33362,#33363);
#27014=AXIS2_PLACEMENT_3D('',#51251,#33367,#33368);
#27015=AXIS2_PLACEMENT_3D('',#51257,#33372,#33373);
#27016=AXIS2_PLACEMENT_3D('',#51263,#33377,#33378);
#27017=AXIS2_PLACEMENT_3D('',#51266,#33381,#33382);
#27018=AXIS2_PLACEMENT_3D('',#51267,#33383,#33384);
#27019=AXIS2_PLACEMENT_3D('',#51269,#33385,#33386);
#27020=AXIS2_PLACEMENT_3D('',#51270,#33387,#33388);
#27021=AXIS2_PLACEMENT_3D('',#51272,#33390,#33391);
#27022=AXIS2_PLACEMENT_3D('',#51274,#33392,#33393);
#27023=AXIS2_PLACEMENT_3D('',#51276,#33395,#33396);
#27024=AXIS2_PLACEMENT_3D('',#51277,#33397,#33398);
#32693=DIRECTION('axis',(0.,0.,1.));
#32694=DIRECTION('refdir',(1.,0.,0.));
#32695=DIRECTION('center_axis',(0.,0.,1.));
#32696=DIRECTION('ref_axis',(1.,0.,0.));
#32697=DIRECTION('',(0.,0.,-1.));
#32698=DIRECTION('center_axis',(0.,0.,-1.));
#32699=DIRECTION('ref_axis',(1.,0.,0.));
#32700=DIRECTION('',(0.,0.,-1.));
#32701=DIRECTION('center_axis',(0.,0.,1.));
#32702=DIRECTION('ref_axis',(1.,0.,0.));
#32703=DIRECTION('center_axis',(0.,0.,-1.));
#32704=DIRECTION('ref_axis',(1.,0.,0.));
#32705=DIRECTION('center_axis',(0.,0.,1.));
#32706=DIRECTION('ref_axis',(1.,0.,0.));
#32707=DIRECTION('',(0.,0.,-1.));
#32708=DIRECTION('center_axis',(0.,0.,1.));
#32709=DIRECTION('ref_axis',(1.,0.,0.));
#32710=DIRECTION('',(0.,0.,-1.));
#32711=DIRECTION('center_axis',(0.,0.,1.));
#32712=DIRECTION('ref_axis',(1.,0.,0.));
#32713=DIRECTION('',(0.,0.,-1.));
#32714=DIRECTION('center_axis',(0.,0.,1.));
#32715=DIRECTION('ref_axis',(1.,0.,0.));
#32716=DIRECTION('',(0.,0.,-1.));
#32717=DIRECTION('center_axis',(0.,0.,1.));
#32718=DIRECTION('ref_axis',(1.,0.,0.));
#32719=DIRECTION('',(0.,0.,-1.));
#32720=DIRECTION('center_axis',(0.,0.,1.));
#32721=DIRECTION('ref_axis',(1.,0.,0.));
#32722=DIRECTION('',(0.,0.,-1.));
#32723=DIRECTION('center_axis',(0.,0.,1.));
#32724=DIRECTION('ref_axis',(1.,0.,0.));
#32725=DIRECTION('',(0.,0.,-1.));
#32726=DIRECTION('center_axis',(0.,0.,1.));
#32727=DIRECTION('ref_axis',(1.,0.,0.));
#32728=DIRECTION('',(0.,0.,-1.));
#32729=DIRECTION('center_axis',(0.,0.,1.));
#32730=DIRECTION('ref_axis',(1.,0.,0.));
#32731=DIRECTION('',(0.,0.,-1.));
#32732=DIRECTION('center_axis',(0.,0.,1.));
#32733=DIRECTION('ref_axis',(1.,0.,0.));
#32734=DIRECTION('',(0.,0.,-1.));
#32735=DIRECTION('center_axis',(0.,0.,1.));
#32736=DIRECTION('ref_axis',(1.,0.,0.));
#32737=DIRECTION('',(0.,0.,-1.));
#32738=DIRECTION('center_axis',(0.,0.,1.));
#32739=DIRECTION('ref_axis',(0.795872373896981,-0.605464420480332,0.));
#32740=DIRECTION('',(0.,0.,1.));
#32741=DIRECTION('center_axis',(0.,0.,1.));
#32742=DIRECTION('ref_axis',(1.,8.36459283980496E-14,0.));
#32743=DIRECTION('center_axis',(0.,0.,1.));
#32744=DIRECTION('ref_axis',(1.,8.36459283980496E-14,0.));
#32745=DIRECTION('',(0.,0.,1.));
#32746=DIRECTION('center_axis',(0.,0.,1.));
#32747=DIRECTION('ref_axis',(1.,8.36459283980496E-14,0.));
#32748=DIRECTION('',(0.,0.,1.));
#32749=DIRECTION('center_axis',(0.,0.,1.));
#32750=DIRECTION('ref_axis',(1.,8.36459283980496E-14,0.));
#32751=DIRECTION('',(0.,0.,1.));
#32752=DIRECTION('center_axis',(0.,0.,1.));
#32753=DIRECTION('ref_axis',(1.,8.36459283980496E-14,0.));
#32754=DIRECTION('',(0.,0.,1.));
#32755=DIRECTION('center_axis',(0.,0.,1.));
#32756=DIRECTION('ref_axis',(1.,8.36459283980496E-14,0.));
#32757=DIRECTION('',(0.,0.,1.));
#32758=DIRECTION('center_axis',(0.,0.,1.));
#32759=DIRECTION('ref_axis',(1.,8.36459283980496E-14,0.));
#32760=DIRECTION('',(0.,0.,1.));
#32761=DIRECTION('center_axis',(0.,0.,1.));
#32762=DIRECTION('ref_axis',(1.,8.36459283980496E-14,0.));
#32763=DIRECTION('',(0.,0.,1.));
#32764=DIRECTION('center_axis',(0.,0.,1.));
#32765=DIRECTION('ref_axis',(1.,8.36459283980496E-14,0.));
#32766=DIRECTION('',(0.,0.,1.));
#32767=DIRECTION('center_axis',(0.,0.,1.));
#32768=DIRECTION('ref_axis',(1.,8.36459283980496E-14,0.));
#32769=DIRECTION('',(0.,0.,1.));
#32770=DIRECTION('center_axis',(0.,0.,1.));
#32771=DIRECTION('ref_axis',(1.,8.36459283980496E-14,0.));
#32772=DIRECTION('',(0.,0.,1.));
#32773=DIRECTION('center_axis',(0.,0.,1.));
#32774=DIRECTION('ref_axis',(1.,8.36459283980496E-14,0.));
#32775=DIRECTION('',(0.,0.,1.));
#32776=DIRECTION('center_axis',(0.,0.,-1.));
#32777=DIRECTION('ref_axis',(1.,8.36459283980496E-14,0.));
#32778=DIRECTION('center_axis',(0.,0.,1.));
#32779=DIRECTION('ref_axis',(1.,0.,0.));
#32780=DIRECTION('center_axis',(0.,0.,1.));
#32781=DIRECTION('ref_axis',(1.,0.,0.));
#32782=DIRECTION('center_axis',(0.,0.,1.));
#32783=DIRECTION('ref_axis',(1.,0.,0.));
#32784=DIRECTION('center_axis',(0.,0.,1.));
#32785=DIRECTION('ref_axis',(1.,0.,0.));
#32786=DIRECTION('center_axis',(0.,0.,-1.));
#32787=DIRECTION('ref_axis',(1.,8.36459283980496E-14,0.));
#32788=DIRECTION('center_axis',(0.,0.,1.));
#32789=DIRECTION('ref_axis',(1.,8.36459283980496E-14,0.));
#32790=DIRECTION('center_axis',(0.,0.,1.));
#32791=DIRECTION('ref_axis',(-0.669920523853501,-0.74243281966778,0.));
#32792=DIRECTION('center_axis',(0.,0.,1.));
#32793=DIRECTION('ref_axis',(1.,0.,0.));
#32794=DIRECTION('center_axis',(0.,0.,1.));
#32795=DIRECTION('ref_axis',(0.984807753012208,-0.17364817766693,0.));
#32796=DIRECTION('center_axis',(0.,0.,-1.));
#32797=DIRECTION('ref_axis',(1.,0.,0.));
#32798=DIRECTION('',(-0.996089805327885,-0.0883464754353932,0.));
#32799=DIRECTION('',(0.905801965515954,-0.423701309022563,0.));
#32800=DIRECTION('center_axis',(-0.423701309022563,-0.905801965515954,0.));
#32801=DIRECTION('ref_axis',(0.905801965515954,-0.423701309022563,0.));
#32802=DIRECTION('',(0.,0.,1.));
#32803=DIRECTION('',(0.,0.,1.));
#32804=DIRECTION('center_axis',(-0.0883464754353932,0.996089805327885,0.));
#32805=DIRECTION('ref_axis',(-0.996089805327885,-0.0883464754353932,0.));
#32806=DIRECTION('',(0.,0.,-1.));
#32807=DIRECTION('center_axis',(0.,0.,1.));
#32808=DIRECTION('ref_axis',(0.939692620785908,-0.342020143325669,0.));
#32809=DIRECTION('center_axis',(0.,0.,-1.));
#32810=DIRECTION('ref_axis',(1.,0.,0.));
#32811=DIRECTION('',(-0.996298167445974,0.0859648855277176,0.));
#32812=DIRECTION('',(0.818465838146947,-0.574555194725812,0.));
#32813=DIRECTION('center_axis',(-0.574555194725812,-0.818465838146947,0.));
#32814=DIRECTION('ref_axis',(0.818465838146947,-0.574555194725812,0.));
#32815=DIRECTION('',(0.,0.,1.));
#32816=DIRECTION('',(0.,0.,1.));
#32817=DIRECTION('center_axis',(0.0859648855277176,0.996298167445974,0.));
#32818=DIRECTION('ref_axis',(-0.996298167445974,0.0859648855277176,0.));
#32819=DIRECTION('',(0.,0.,-1.));
#32820=DIRECTION('center_axis',(0.,0.,1.));
#32821=DIRECTION('ref_axis',(0.866025403784438,-0.5,0.));
#32822=DIRECTION('center_axis',(0.,0.,-1.));
#32823=DIRECTION('ref_axis',(1.,0.,0.));
#32824=DIRECTION('',(-0.966234513897416,0.257664246944399,0.));
#32825=DIRECTION('',(0.706261040449543,-0.707951511576272,0.));
#32826=DIRECTION('center_axis',(-0.707951511576272,-0.706261040449543,0.));
#32827=DIRECTION('ref_axis',(0.706261040449543,-0.707951511576272,0.));
#32828=DIRECTION('',(0.,0.,1.));
#32829=DIRECTION('',(0.,0.,1.));
#32830=DIRECTION('center_axis',(0.257664246944399,0.966234513897416,0.));
#32831=DIRECTION('ref_axis',(-0.966234513897416,0.257664246944399,0.));
#32832=DIRECTION('',(0.,0.,-1.));
#32833=DIRECTION('center_axis',(0.,0.,1.));
#32834=DIRECTION('ref_axis',(0.766044443118978,-0.64278760968654,0.));
#32835=DIRECTION('center_axis',(0.,0.,-1.));
#32836=DIRECTION('ref_axis',(1.,0.,0.));
#32837=DIRECTION('',(-0.906812313582341,0.421534610602074,0.));
#32838=DIRECTION('',(0.572596858423411,-0.819837079988238,0.));
#32839=DIRECTION('center_axis',(-0.819837079988238,-0.572596858423411,0.));
#32840=DIRECTION('ref_axis',(0.572596858423411,-0.819837079988238,0.));
#32841=DIRECTION('',(0.,0.,1.));
#32842=DIRECTION('',(0.,0.,1.));
#32843=DIRECTION('center_axis',(0.421534610602074,0.906812313582341,0.));
#32844=DIRECTION('ref_axis',(-0.906812313582341,0.421534610602074,0.));
#32845=DIRECTION('',(0.,0.,-1.));
#32846=DIRECTION('center_axis',(0.,0.,1.));
#32847=DIRECTION('ref_axis',(0.642787609686539,-0.766044443118978,0.));
#32848=DIRECTION('center_axis',(0.,0.,-1.));
#32849=DIRECTION('ref_axis',(1.,0.,0.));
#32850=DIRECTION('',(-0.819837079988238,0.572596858423411,0.));
#32851=DIRECTION('',(0.421534610602074,-0.906812313582341,0.));
#32852=DIRECTION('center_axis',(-0.906812313582341,-0.421534610602074,0.));
#32853=DIRECTION('ref_axis',(0.421534610602074,-0.906812313582341,0.));
#32854=DIRECTION('',(0.,0.,1.));
#32855=DIRECTION('',(0.,0.,1.));
#32856=DIRECTION('center_axis',(0.572596858423411,0.819837079988238,0.));
#32857=DIRECTION('ref_axis',(-0.819837079988238,0.572596858423411,0.));
#32858=DIRECTION('',(0.,0.,-1.));
#32859=DIRECTION('center_axis',(0.,0.,1.));
#32860=DIRECTION('ref_axis',(0.5,-0.866025403784438,0.));
#32861=DIRECTION('center_axis',(0.,0.,-1.));
#32862=DIRECTION('ref_axis',(1.,0.,0.));
#32863=DIRECTION('',(-0.707951511576272,0.706261040449544,0.));
#32864=DIRECTION('',(0.257664246944398,-0.966234513897416,0.));
#32865=DIRECTION('center_axis',(-0.966234513897416,-0.257664246944398,0.));
#32866=DIRECTION('ref_axis',(0.257664246944398,-0.966234513897416,0.));
#32867=DIRECTION('',(0.,0.,1.));
#32868=DIRECTION('',(0.,0.,1.));
#32869=DIRECTION('center_axis',(0.706261040449544,0.707951511576272,0.));
#32870=DIRECTION('ref_axis',(-0.707951511576272,0.706261040449544,0.));
#32871=DIRECTION('',(0.,0.,-1.));
#32872=DIRECTION('center_axis',(0.,0.,1.));
#32873=DIRECTION('ref_axis',(0.342020143325668,-0.939692620785909,0.));
#32874=DIRECTION('center_axis',(0.,0.,-1.));
#32875=DIRECTION('ref_axis',(1.,0.,0.));
#32876=DIRECTION('',(-0.57455519472581,0.818465838146948,0.));
#32877=DIRECTION('',(0.0859648855277162,-0.996298167445974,0.));
#32878=DIRECTION('center_axis',(-0.996298167445974,-0.0859648855277162,
0.));
#32879=DIRECTION('ref_axis',(0.0859648855277162,-0.996298167445974,0.));
#32880=DIRECTION('',(0.,0.,1.));
#32881=DIRECTION('',(0.,0.,1.));
#32882=DIRECTION('center_axis',(0.818465838146948,0.57455519472581,0.));
#32883=DIRECTION('ref_axis',(-0.57455519472581,0.818465838146948,0.));
#32884=DIRECTION('',(0.,0.,-1.));
#32885=DIRECTION('center_axis',(0.,0.,1.));
#32886=DIRECTION('ref_axis',(0.17364817766693,-0.984807753012208,0.));
#32887=DIRECTION('center_axis',(0.,0.,-1.));
#32888=DIRECTION('ref_axis',(1.,0.,0.));
#32889=DIRECTION('',(-0.423701309022563,0.905801965515955,0.));
#32890=DIRECTION('',(-0.0883464754353936,-0.996089805327885,0.));
#32891=DIRECTION('center_axis',(-0.996089805327885,0.0883464754353937,0.));
#32892=DIRECTION('ref_axis',(-0.0883464754353937,-0.996089805327885,0.));
#32893=DIRECTION('',(0.,0.,1.));
#32894=DIRECTION('',(0.,0.,1.));
#32895=DIRECTION('center_axis',(0.905801965515955,0.423701309022563,0.));
#32896=DIRECTION('ref_axis',(-0.423701309022563,0.905801965515955,0.));
#32897=DIRECTION('',(0.,0.,-1.));
#32898=DIRECTION('center_axis',(0.,0.,1.));
#32899=DIRECTION('ref_axis',(-1.94289029309402E-16,-1.,0.));
#32900=DIRECTION('center_axis',(0.,0.,-1.));
#32901=DIRECTION('ref_axis',(1.,0.,0.));
#32902=DIRECTION('',(-0.259973473447872,0.96561575852067,0.));
#32903=DIRECTION('',(-0.259973473447873,-0.96561575852067,0.));
#32904=DIRECTION('center_axis',(-0.96561575852067,0.259973473447873,0.));
#32905=DIRECTION('ref_axis',(-0.259973473447873,-0.96561575852067,0.));
#32906=DIRECTION('',(0.,0.,1.));
#32907=DIRECTION('',(0.,0.,1.));
#32908=DIRECTION('center_axis',(0.96561575852067,0.259973473447872,0.));
#32909=DIRECTION('ref_axis',(-0.259973473447872,0.96561575852067,0.));
#32910=DIRECTION('',(0.,0.,-1.));
#32911=DIRECTION('center_axis',(0.,0.,1.));
#32912=DIRECTION('ref_axis',(-0.17364817766693,-0.984807753012208,0.));
#32913=DIRECTION('center_axis',(0.,0.,-1.));
#32914=DIRECTION('ref_axis',(1.,0.,0.));
#32915=DIRECTION('',(-0.0883464754353933,0.996089805327885,0.));
#32916=DIRECTION('',(-0.423701309022563,-0.905801965515955,0.));
#32917=DIRECTION('center_axis',(-0.905801965515955,0.423701309022563,0.));
#32918=DIRECTION('ref_axis',(-0.423701309022563,-0.905801965515955,0.));
#32919=DIRECTION('',(0.,0.,1.));
#32920=DIRECTION('',(0.,0.,1.));
#32921=DIRECTION('center_axis',(0.996089805327885,0.0883464754353932,0.));
#32922=DIRECTION('ref_axis',(-0.0883464754353932,0.996089805327885,0.));
#32923=DIRECTION('',(0.,0.,-1.));
#32924=DIRECTION('center_axis',(0.,0.,1.));
#32925=DIRECTION('ref_axis',(-0.342020143325669,-0.939692620785908,0.));
#32926=DIRECTION('center_axis',(0.,0.,-1.));
#32927=DIRECTION('ref_axis',(1.,0.,0.));
#32928=DIRECTION('',(0.0859648855277175,0.996298167445974,0.));
#32929=DIRECTION('',(-0.574555194725811,-0.818465838146947,0.));
#32930=DIRECTION('center_axis',(-0.818465838146947,0.574555194725811,0.));
#32931=DIRECTION('ref_axis',(-0.574555194725811,-0.818465838146947,0.));
#32932=DIRECTION('',(0.,0.,1.));
#32933=DIRECTION('',(0.,0.,1.));
#32934=DIRECTION('center_axis',(0.996298167445974,-0.0859648855277175,0.));
#32935=DIRECTION('ref_axis',(0.0859648855277175,0.996298167445974,0.));
#32936=DIRECTION('',(0.,0.,-1.));
#32937=DIRECTION('center_axis',(0.,0.,1.));
#32938=DIRECTION('ref_axis',(-0.5,-0.866025403784438,0.));
#32939=DIRECTION('center_axis',(0.,0.,-1.));
#32940=DIRECTION('ref_axis',(1.,0.,0.));
#32941=DIRECTION('',(0.257664246944399,0.966234513897416,0.));
#32942=DIRECTION('',(-0.707951511576272,-0.706261040449543,0.));
#32943=DIRECTION('center_axis',(-0.706261040449543,0.707951511576272,0.));
#32944=DIRECTION('ref_axis',(-0.707951511576272,-0.706261040449543,0.));
#32945=DIRECTION('',(0.,0.,1.));
#32946=DIRECTION('',(0.,0.,1.));
#32947=DIRECTION('center_axis',(0.966234513897416,-0.257664246944399,0.));
#32948=DIRECTION('ref_axis',(0.257664246944399,0.966234513897416,0.));
#32949=DIRECTION('',(0.,0.,-1.));
#32950=DIRECTION('center_axis',(0.,0.,1.));
#32951=DIRECTION('ref_axis',(-0.642787609686539,-0.766044443118978,0.));
#32952=DIRECTION('center_axis',(0.,0.,-1.));
#32953=DIRECTION('ref_axis',(1.,0.,0.));
#32954=DIRECTION('',(0.421534610602074,0.906812313582341,0.));
#32955=DIRECTION('',(-0.819837079988238,-0.572596858423411,0.));
#32956=DIRECTION('center_axis',(-0.572596858423411,0.819837079988238,0.));
#32957=DIRECTION('ref_axis',(-0.819837079988238,-0.572596858423411,0.));
#32958=DIRECTION('',(0.,0.,1.));
#32959=DIRECTION('',(0.,0.,1.));
#32960=DIRECTION('center_axis',(0.906812313582341,-0.421534610602074,0.));
#32961=DIRECTION('ref_axis',(0.421534610602074,0.906812313582341,0.));
#32962=DIRECTION('',(0.,0.,-1.));
#32963=DIRECTION('center_axis',(0.,0.,1.));
#32964=DIRECTION('ref_axis',(-0.766044443118978,-0.642787609686539,0.));
#32965=DIRECTION('center_axis',(0.,0.,-1.));
#32966=DIRECTION('ref_axis',(1.,0.,0.));
#32967=DIRECTION('',(0.572596858423411,0.819837079988238,0.));
#32968=DIRECTION('',(-0.906812313582341,-0.421534610602074,0.));
#32969=DIRECTION('center_axis',(-0.421534610602074,0.906812313582341,0.));
#32970=DIRECTION('ref_axis',(-0.906812313582341,-0.421534610602074,0.));
#32971=DIRECTION('',(0.,0.,1.));
#32972=DIRECTION('',(0.,0.,1.));
#32973=DIRECTION('center_axis',(0.819837079988238,-0.572596858423411,0.));
#32974=DIRECTION('ref_axis',(0.572596858423411,0.819837079988238,0.));
#32975=DIRECTION('',(0.,0.,-1.));
#32976=DIRECTION('center_axis',(0.,0.,1.));
#32977=DIRECTION('ref_axis',(-0.866025403784439,-0.5,0.));
#32978=DIRECTION('center_axis',(0.,0.,-1.));
#32979=DIRECTION('ref_axis',(1.,0.,0.));
#32980=DIRECTION('',(0.706261040449544,0.707951511576271,0.));
#32981=DIRECTION('',(-0.966234513897416,-0.257664246944398,0.));
#32982=DIRECTION('center_axis',(-0.257664246944398,0.966234513897416,0.));
#32983=DIRECTION('ref_axis',(-0.966234513897416,-0.257664246944398,0.));
#32984=DIRECTION('',(0.,0.,1.));
#32985=DIRECTION('',(0.,0.,1.));
#32986=DIRECTION('center_axis',(0.707951511576271,-0.706261040449544,0.));
#32987=DIRECTION('ref_axis',(0.706261040449544,0.707951511576271,0.));
#32988=DIRECTION('',(0.,0.,-1.));
#32989=DIRECTION('center_axis',(0.,0.,1.));
#32990=DIRECTION('ref_axis',(-0.939692620785909,-0.342020143325669,0.));
#32991=DIRECTION('center_axis',(0.,0.,-1.));
#32992=DIRECTION('ref_axis',(1.,0.,0.));
#32993=DIRECTION('',(0.818465838146948,0.574555194725811,0.));
#32994=DIRECTION('',(-0.996298167445974,-0.0859648855277167,0.));
#32995=DIRECTION('center_axis',(-0.0859648855277167,0.996298167445974,0.));
#32996=DIRECTION('ref_axis',(-0.996298167445974,-0.0859648855277167,0.));
#32997=DIRECTION('',(0.,0.,1.));
#32998=DIRECTION('',(0.,0.,1.));
#32999=DIRECTION('center_axis',(0.574555194725811,-0.818465838146948,0.));
#33000=DIRECTION('ref_axis',(0.818465838146948,0.574555194725811,0.));
#33001=DIRECTION('',(0.,0.,-1.));
#33002=DIRECTION('center_axis',(0.,0.,1.));
#33003=DIRECTION('ref_axis',(-0.984807753012208,-0.17364817766693,0.));
#33004=DIRECTION('center_axis',(0.,0.,-1.));
#33005=DIRECTION('ref_axis',(1.,0.,0.));
#33006=DIRECTION('',(0.905801965515955,0.423701309022563,0.));
#33007=DIRECTION('',(-0.996089805327885,0.0883464754353936,0.));
#33008=DIRECTION('center_axis',(0.0883464754353936,0.996089805327885,0.));
#33009=DIRECTION('ref_axis',(-0.996089805327885,0.0883464754353936,0.));
#33010=DIRECTION('',(0.,0.,1.));
#33011=DIRECTION('',(0.,0.,1.));
#33012=DIRECTION('center_axis',(0.423701309022563,-0.905801965515955,0.));
#33013=DIRECTION('ref_axis',(0.905801965515955,0.423701309022563,0.));
#33014=DIRECTION('',(0.,0.,-1.));
#33015=DIRECTION('center_axis',(0.,0.,1.));
#33016=DIRECTION('ref_axis',(-1.,1.11022302462516E-16,0.));
#33017=DIRECTION('center_axis',(0.,0.,-1.));
#33018=DIRECTION('ref_axis',(1.,0.,0.));
#33019=DIRECTION('',(0.96561575852067,0.259973473447872,0.));
#33020=DIRECTION('',(-0.96561575852067,0.259973473447873,0.));
#33021=DIRECTION('center_axis',(0.,0.,-1.));
#33022=DIRECTION('ref_axis',(1.,0.,0.));
#33023=DIRECTION('center_axis',(0.259973473447873,0.96561575852067,0.));
#33024=DIRECTION('ref_axis',(-0.96561575852067,0.259973473447873,0.));
#33025=DIRECTION('',(0.,0.,1.));
#33026=DIRECTION('',(0.,0.,1.));
#33027=DIRECTION('center_axis',(0.259973473447872,-0.96561575852067,0.));
#33028=DIRECTION('ref_axis',(0.96561575852067,0.259973473447872,0.));
#33029=DIRECTION('',(0.,0.,-1.));
#33030=DIRECTION('center_axis',(0.,0.,1.));
#33031=DIRECTION('ref_axis',(-0.984807753012208,0.173648177666931,0.));
#33032=DIRECTION('center_axis',(0.,0.,-1.));
#33033=DIRECTION('ref_axis',(1.,0.,0.));
#33034=DIRECTION('',(0.996089805327885,0.0883464754353928,0.));
#33035=DIRECTION('',(-0.905801965515954,0.423701309022564,0.));
#33036=DIRECTION('center_axis',(0.423701309022564,0.905801965515954,0.));
#33037=DIRECTION('ref_axis',(-0.905801965515954,0.423701309022564,0.));
#33038=DIRECTION('',(0.,0.,1.));
#33039=DIRECTION('',(0.,0.,1.));
#33040=DIRECTION('center_axis',(0.0883464754353928,-0.996089805327885,0.));
#33041=DIRECTION('ref_axis',(0.996089805327885,0.0883464754353928,0.));
#33042=DIRECTION('',(0.,0.,-1.));
#33043=DIRECTION('center_axis',(0.,0.,1.));
#33044=DIRECTION('ref_axis',(-0.939692620785908,0.342020143325669,0.));
#33045=DIRECTION('center_axis',(0.,0.,-1.));
#33046=DIRECTION('ref_axis',(1.,0.,0.));
#33047=DIRECTION('',(0.996298167445974,-0.085964885527717,0.));
#33048=DIRECTION('',(-0.818465838146948,0.574555194725811,0.));
#33049=DIRECTION('center_axis',(0.574555194725811,0.818465838146948,0.));
#33050=DIRECTION('ref_axis',(-0.818465838146948,0.574555194725811,0.));
#33051=DIRECTION('',(0.,0.,1.));
#33052=DIRECTION('',(0.,0.,1.));
#33053=DIRECTION('center_axis',(-0.085964885527717,-0.996298167445974,0.));
#33054=DIRECTION('ref_axis',(0.996298167445974,-0.085964885527717,0.));
#33055=DIRECTION('',(0.,0.,-1.));
#33056=DIRECTION('center_axis',(0.,0.,1.));
#33057=DIRECTION('ref_axis',(-0.866025403784439,0.5,0.));
#33058=DIRECTION('center_axis',(0.,0.,-1.));
#33059=DIRECTION('ref_axis',(1.,0.,0.));
#33060=DIRECTION('',(0.966234513897416,-0.257664246944398,0.));
#33061=DIRECTION('',(-0.706261040449544,0.707951511576272,0.));
#33062=DIRECTION('center_axis',(0.707951511576272,0.706261040449544,0.));
#33063=DIRECTION('ref_axis',(-0.706261040449544,0.707951511576272,0.));
#33064=DIRECTION('',(0.,0.,1.));
#33065=DIRECTION('',(0.,0.,1.));
#33066=DIRECTION('center_axis',(-0.257664246944398,-0.966234513897416,0.));
#33067=DIRECTION('ref_axis',(0.966234513897416,-0.257664246944398,0.));
#33068=DIRECTION('',(0.,0.,-1.));
#33069=DIRECTION('center_axis',(0.,0.,1.));
#33070=DIRECTION('ref_axis',(-0.766044443118978,0.642787609686539,0.));
#33071=DIRECTION('center_axis',(0.,0.,-1.));
#33072=DIRECTION('ref_axis',(1.,0.,0.));
#33073=DIRECTION('',(0.906812313582341,-0.421534610602074,0.));
#33074=DIRECTION('',(-0.572596858423411,0.819837079988238,0.));
#33075=DIRECTION('center_axis',(0.819837079988238,0.572596858423411,0.));
#33076=DIRECTION('ref_axis',(-0.572596858423411,0.819837079988238,0.));
#33077=DIRECTION('',(0.,0.,1.));
#33078=DIRECTION('',(0.,0.,1.));
#33079=DIRECTION('center_axis',(-0.421534610602074,-0.906812313582341,0.));
#33080=DIRECTION('ref_axis',(0.906812313582341,-0.421534610602074,0.));
#33081=DIRECTION('',(0.,0.,-1.));
#33082=DIRECTION('center_axis',(0.,0.,1.));
#33083=DIRECTION('ref_axis',(-0.642787609686539,0.766044443118978,0.));
#33084=DIRECTION('center_axis',(0.,0.,-1.));
#33085=DIRECTION('ref_axis',(1.,0.,0.));
#33086=DIRECTION('',(0.819837079988238,-0.572596858423411,0.));
#33087=DIRECTION('',(-0.421534610602074,0.906812313582341,0.));
#33088=DIRECTION('center_axis',(0.906812313582341,0.421534610602074,0.));
#33089=DIRECTION('ref_axis',(-0.421534610602074,0.906812313582341,0.));
#33090=DIRECTION('',(0.,0.,1.));
#33091=DIRECTION('',(0.,0.,1.));
#33092=DIRECTION('center_axis',(-0.572596858423411,-0.819837079988238,0.));
#33093=DIRECTION('ref_axis',(0.819837079988238,-0.572596858423411,0.));
#33094=DIRECTION('',(0.,0.,-1.));
#33095=DIRECTION('center_axis',(0.,0.,1.));
#33096=DIRECTION('ref_axis',(-0.5,0.866025403784439,0.));
#33097=DIRECTION('center_axis',(0.,0.,-1.));
#33098=DIRECTION('ref_axis',(1.,0.,0.));
#33099=DIRECTION('',(0.707951511576272,-0.706261040449544,0.));
#33100=DIRECTION('',(-0.257664246944398,0.966234513897416,0.));
#33101=DIRECTION('center_axis',(0.966234513897416,0.257664246944398,0.));
#33102=DIRECTION('ref_axis',(-0.257664246944398,0.966234513897416,0.));
#33103=DIRECTION('',(0.,0.,1.));
#33104=DIRECTION('',(0.,0.,1.));
#33105=DIRECTION('center_axis',(-0.706261040449544,-0.707951511576272,0.));
#33106=DIRECTION('ref_axis',(0.707951511576272,-0.706261040449544,0.));
#33107=DIRECTION('',(0.,0.,-1.));
#33108=DIRECTION('center_axis',(0.,0.,1.));
#33109=DIRECTION('ref_axis',(-0.342020143325669,0.939692620785909,0.));
#33110=DIRECTION('center_axis',(0.,0.,-1.));
#33111=DIRECTION('ref_axis',(1.,0.,0.));
#33112=DIRECTION('',(0.574555194725811,-0.818465838146948,0.));
#33113=DIRECTION('',(-0.0859648855277167,0.996298167445974,0.));
#33114=DIRECTION('center_axis',(0.996298167445974,0.0859648855277167,0.));
#33115=DIRECTION('ref_axis',(-0.0859648855277167,0.996298167445974,0.));
#33116=DIRECTION('',(0.,0.,1.));
#33117=DIRECTION('',(0.,0.,1.));
#33118=DIRECTION('center_axis',(-0.818465838146948,-0.574555194725811,0.));
#33119=DIRECTION('ref_axis',(0.574555194725811,-0.818465838146948,0.));
#33120=DIRECTION('',(0.,0.,-1.));
#33121=DIRECTION('center_axis',(0.,0.,1.));
#33122=DIRECTION('ref_axis',(-0.17364817766693,0.984807753012208,0.));
#33123=DIRECTION('center_axis',(0.,0.,-1.));
#33124=DIRECTION('ref_axis',(1.,0.,0.));
#33125=DIRECTION('',(0.423701309022563,-0.905801965515955,0.));
#33126=DIRECTION('',(0.0883464754353932,0.996089805327885,0.));
#33127=DIRECTION('center_axis',(0.996089805327885,-0.0883464754353932,0.));
#33128=DIRECTION('ref_axis',(0.0883464754353932,0.996089805327885,0.));
#33129=DIRECTION('',(0.,0.,1.));
#33130=DIRECTION('',(0.,0.,1.));
#33131=DIRECTION('center_axis',(-0.905801965515955,-0.423701309022563,0.));
#33132=DIRECTION('ref_axis',(0.423701309022563,-0.905801965515955,0.));
#33133=DIRECTION('',(0.,0.,-1.));
#33134=DIRECTION('center_axis',(0.,0.,1.));
#33135=DIRECTION('ref_axis',(5.55111512312578E-17,1.,0.));
#33136=DIRECTION('center_axis',(0.,0.,-1.));
#33137=DIRECTION('ref_axis',(1.,0.,0.));
#33138=DIRECTION('',(0.259973473447872,-0.96561575852067,0.));
#33139=DIRECTION('',(0.259973473447872,0.96561575852067,0.));
#33140=DIRECTION('center_axis',(0.96561575852067,-0.259973473447873,0.));
#33141=DIRECTION('ref_axis',(0.259973473447873,0.96561575852067,0.));
#33142=DIRECTION('',(0.,0.,1.));
#33143=DIRECTION('',(0.,0.,1.));
#33144=DIRECTION('center_axis',(-0.96561575852067,-0.259973473447872,0.));
#33145=DIRECTION('ref_axis',(0.259973473447872,-0.96561575852067,0.));
#33146=DIRECTION('',(0.,0.,-1.));
#33147=DIRECTION('center_axis',(0.,0.,1.));
#33148=DIRECTION('ref_axis',(0.17364817766693,0.984807753012208,0.));
#33149=DIRECTION('center_axis',(0.,0.,-1.));
#33150=DIRECTION('ref_axis',(1.,0.,0.));
#33151=DIRECTION('',(0.0883464754353931,-0.996089805327885,0.));
#33152=DIRECTION('',(0.423701309022563,0.905801965515954,0.));
#33153=DIRECTION('center_axis',(0.905801965515954,-0.423701309022563,0.));
#33154=DIRECTION('ref_axis',(0.423701309022563,0.905801965515954,0.));
#33155=DIRECTION('',(0.,0.,1.));
#33156=DIRECTION('',(0.,0.,1.));
#33157=DIRECTION('center_axis',(-0.996089805327885,-0.0883464754353932,
0.));
#33158=DIRECTION('ref_axis',(0.0883464754353932,-0.996089805327885,0.));
#33159=DIRECTION('',(0.,0.,-1.));
#33160=DIRECTION('center_axis',(0.,0.,1.));
#33161=DIRECTION('ref_axis',(0.342020143325669,0.939692620785908,0.));
#33162=DIRECTION('center_axis',(0.,0.,-1.));
#33163=DIRECTION('ref_axis',(1.,0.,0.));
#33164=DIRECTION('',(-0.085964885527717,-0.996298167445974,0.));
#33165=DIRECTION('',(0.574555194725811,0.818465838146948,0.));
#33166=DIRECTION('center_axis',(0.818465838146948,-0.574555194725811,0.));
#33167=DIRECTION('ref_axis',(0.574555194725811,0.818465838146948,0.));
#33168=DIRECTION('',(0.,0.,1.));
#33169=DIRECTION('',(0.,0.,1.));
#33170=DIRECTION('center_axis',(-0.996298167445974,0.085964885527717,0.));
#33171=DIRECTION('ref_axis',(-0.085964885527717,-0.996298167445974,0.));
#33172=DIRECTION('',(0.,0.,-1.));
#33173=DIRECTION('center_axis',(0.,0.,1.));
#33174=DIRECTION('ref_axis',(0.5,0.866025403784439,0.));
#33175=DIRECTION('center_axis',(0.,0.,-1.));
#33176=DIRECTION('ref_axis',(1.,0.,0.));
#33177=DIRECTION('',(-0.257664246944398,-0.966234513897416,0.));
#33178=DIRECTION('',(0.707951511576272,0.706261040449544,0.));
#33179=DIRECTION('center_axis',(0.706261040449544,-0.707951511576272,0.));
#33180=DIRECTION('ref_axis',(0.707951511576272,0.706261040449544,0.));
#33181=DIRECTION('',(0.,0.,1.));
#33182=DIRECTION('',(0.,0.,1.));
#33183=DIRECTION('center_axis',(-0.966234513897416,0.257664246944398,0.));
#33184=DIRECTION('ref_axis',(-0.257664246944398,-0.966234513897416,0.));
#33185=DIRECTION('',(0.,0.,-1.));
#33186=DIRECTION('center_axis',(0.,0.,1.));
#33187=DIRECTION('ref_axis',(0.642787609686539,0.766044443118978,0.));
#33188=DIRECTION('center_axis',(0.,0.,-1.));
#33189=DIRECTION('ref_axis',(1.,0.,0.));
#33190=DIRECTION('',(-0.421534610602074,-0.906812313582341,0.));
#33191=DIRECTION('',(0.819837079988238,0.572596858423411,0.));
#33192=DIRECTION('center_axis',(0.572596858423411,-0.819837079988238,0.));
#33193=DIRECTION('ref_axis',(0.819837079988238,0.572596858423411,0.));
#33194=DIRECTION('',(0.,0.,1.));
#33195=DIRECTION('',(0.,0.,1.));
#33196=DIRECTION('center_axis',(-0.906812313582341,0.421534610602074,0.));
#33197=DIRECTION('ref_axis',(-0.421534610602074,-0.906812313582341,0.));
#33198=DIRECTION('',(0.,0.,-1.));
#33199=DIRECTION('center_axis',(0.,0.,1.));
#33200=DIRECTION('ref_axis',(0.766044443118978,0.642787609686539,0.));
#33201=DIRECTION('center_axis',(0.,0.,-1.));
#33202=DIRECTION('ref_axis',(1.,0.,0.));
#33203=DIRECTION('',(-0.572596858423411,-0.819837079988238,0.));
#33204=DIRECTION('',(0.906812313582341,0.421534610602074,0.));
#33205=DIRECTION('center_axis',(0.421534610602074,-0.906812313582341,0.));
#33206=DIRECTION('ref_axis',(0.906812313582341,0.421534610602074,0.));
#33207=DIRECTION('',(0.,0.,1.));
#33208=DIRECTION('',(0.,0.,1.));
#33209=DIRECTION('center_axis',(-0.819837079988238,0.572596858423411,0.));
#33210=DIRECTION('ref_axis',(-0.572596858423411,-0.819837079988238,0.));
#33211=DIRECTION('',(0.,0.,-1.));
#33212=DIRECTION('center_axis',(0.,0.,1.));
#33213=DIRECTION('ref_axis',(0.866025403784439,0.5,0.));
#33214=DIRECTION('center_axis',(0.,0.,-1.));
#33215=DIRECTION('ref_axis',(1.,0.,0.));
#33216=DIRECTION('',(-0.706261040449544,-0.707951511576272,0.));
#33217=DIRECTION('',(0.966234513897416,0.257664246944398,0.));
#33218=DIRECTION('center_axis',(0.257664246944398,-0.966234513897416,0.));
#33219=DIRECTION('ref_axis',(0.966234513897416,0.257664246944398,0.));
#33220=DIRECTION('',(0.,0.,1.));
#33221=DIRECTION('',(0.,0.,1.));
#33222=DIRECTION('center_axis',(-0.707951511576272,0.706261040449544,0.));
#33223=DIRECTION('ref_axis',(-0.706261040449544,-0.707951511576272,0.));
#33224=DIRECTION('',(0.,0.,-1.));
#33225=DIRECTION('center_axis',(0.,0.,1.));
#33226=DIRECTION('ref_axis',(0.939692620785909,0.342020143325669,0.));
#33227=DIRECTION('center_axis',(0.,0.,-1.));
#33228=DIRECTION('ref_axis',(1.,0.,0.));
#33229=DIRECTION('',(-0.818465838146948,-0.574555194725811,0.));
#33230=DIRECTION('',(0.996298167445974,0.0859648855277167,0.));
#33231=DIRECTION('center_axis',(0.0859648855277167,-0.996298167445974,0.));
#33232=DIRECTION('ref_axis',(0.996298167445974,0.0859648855277167,0.));
#33233=DIRECTION('',(0.,0.,1.));
#33234=DIRECTION('',(0.,0.,1.));
#33235=DIRECTION('center_axis',(-0.574555194725811,0.818465838146948,0.));
#33236=DIRECTION('ref_axis',(-0.818465838146948,-0.574555194725811,0.));
#33237=DIRECTION('',(0.,0.,-1.));
#33238=DIRECTION('center_axis',(0.,0.,1.));
#33239=DIRECTION('ref_axis',(0.984807753012208,0.17364817766693,0.));
#33240=DIRECTION('center_axis',(0.,0.,-1.));
#33241=DIRECTION('ref_axis',(1.,0.,0.));
#33242=DIRECTION('',(-0.905801965515955,-0.423701309022563,0.));
#33243=DIRECTION('',(0.996089805327885,-0.0883464754353932,0.));
#33244=DIRECTION('center_axis',(-0.0883464754353933,-0.996089805327885,
0.));
#33245=DIRECTION('ref_axis',(0.996089805327885,-0.0883464754353933,0.));
#33246=DIRECTION('',(0.,0.,1.));
#33247=DIRECTION('',(0.,0.,1.));
#33248=DIRECTION('center_axis',(-0.423701309022563,0.905801965515955,0.));
#33249=DIRECTION('ref_axis',(-0.905801965515954,-0.423701309022563,0.));
#33250=DIRECTION('',(0.,0.,-1.));
#33251=DIRECTION('center_axis',(0.,0.,1.));
#33252=DIRECTION('ref_axis',(1.,0.,0.));
#33253=DIRECTION('center_axis',(0.,0.,1.));
#33254=DIRECTION('ref_axis',(1.,0.,0.));
#33255=DIRECTION('center_axis',(0.,0.,1.));
#33256=DIRECTION('ref_axis',(1.,0.,0.));
#33257=DIRECTION('center_axis',(0.,0.,1.));
#33258=DIRECTION('ref_axis',(1.,0.,0.));
#33259=DIRECTION('center_axis',(0.,0.,1.));
#33260=DIRECTION('ref_axis',(1.,0.,0.));
#33261=DIRECTION('center_axis',(0.,0.,1.));
#33262=DIRECTION('ref_axis',(1.,0.,0.));
#33263=DIRECTION('center_axis',(0.,0.,1.));
#33264=DIRECTION('ref_axis',(1.,0.,0.));
#33265=DIRECTION('center_axis',(0.,0.,1.));
#33266=DIRECTION('ref_axis',(1.,0.,0.));
#33267=DIRECTION('center_axis',(0.,0.,1.));
#33268=DIRECTION('ref_axis',(1.,0.,0.));
#33269=DIRECTION('center_axis',(0.,0.,1.));
#33270=DIRECTION('ref_axis',(1.,0.,0.));
#33271=DIRECTION('center_axis',(0.,0.,1.));
#33272=DIRECTION('ref_axis',(1.,0.,0.));
#33273=DIRECTION('center_axis',(0.,0.,1.));
#33274=DIRECTION('ref_axis',(1.,0.,0.));
#33275=DIRECTION('center_axis',(0.,0.,1.));
#33276=DIRECTION('ref_axis',(1.,0.,0.));
#33277=DIRECTION('center_axis',(0.,0.,1.));
#33278=DIRECTION('ref_axis',(1.,0.,0.));
#33279=DIRECTION('center_axis',(0.,0.,1.));
#33280=DIRECTION('ref_axis',(1.,0.,0.));
#33281=DIRECTION('center_axis',(0.,0.,1.));
#33282=DIRECTION('ref_axis',(1.,0.,0.));
#33283=DIRECTION('center_axis',(0.,0.,1.));
#33284=DIRECTION('ref_axis',(1.,0.,0.));
#33285=DIRECTION('center_axis',(0.,0.,1.));
#33286=DIRECTION('ref_axis',(1.,0.,0.));
#33287=DIRECTION('',(0.,0.,-1.));
#33288=DIRECTION('center_axis',(0.,0.,1.));
#33289=DIRECTION('ref_axis',(1.,0.,0.));
#33290=DIRECTION('center_axis',(0.,0.,1.));
#33291=DIRECTION('ref_axis',(1.,0.,0.));
#33292=DIRECTION('center_axis',(0.,0.,1.));
#33293=DIRECTION('ref_axis',(1.,0.,0.));
#33294=DIRECTION('center_axis',(0.,0.,1.));
#33295=DIRECTION('ref_axis',(1.,0.,0.));
#33296=DIRECTION('center_axis',(0.,0.,1.));
#33297=DIRECTION('ref_axis',(1.,0.,0.));
#33298=DIRECTION('center_axis',(0.,0.,1.));
#33299=DIRECTION('ref_axis',(1.,0.,0.));
#33300=DIRECTION('center_axis',(0.,0.,1.));
#33301=DIRECTION('ref_axis',(1.,0.,0.));
#33302=DIRECTION('center_axis',(0.,0.,1.));
#33303=DIRECTION('ref_axis',(1.,0.,0.));
#33304=DIRECTION('center_axis',(0.,0.,1.));
#33305=DIRECTION('ref_axis',(1.,0.,0.));
#33306=DIRECTION('center_axis',(0.,0.,1.));
#33307=DIRECTION('ref_axis',(1.,0.,0.));
#33308=DIRECTION('center_axis',(0.,0.,1.));
#33309=DIRECTION('ref_axis',(1.,0.,0.));
#33310=DIRECTION('center_axis',(0.,0.,1.));
#33311=DIRECTION('ref_axis',(1.,0.,0.));
#33312=DIRECTION('center_axis',(0.,0.,1.));
#33313=DIRECTION('ref_axis',(1.,0.,0.));
#33314=DIRECTION('center_axis',(0.,0.,1.));
#33315=DIRECTION('ref_axis',(1.,0.,0.));
#33316=DIRECTION('center_axis',(0.,0.,1.));
#33317=DIRECTION('ref_axis',(1.,0.,0.));
#33318=DIRECTION('center_axis',(0.,0.,1.));
#33319=DIRECTION('ref_axis',(1.,0.,0.));
#33320=DIRECTION('center_axis',(0.,0.,1.));
#33321=DIRECTION('ref_axis',(1.,0.,0.));
#33322=DIRECTION('center_axis',(0.,0.,1.));
#33323=DIRECTION('ref_axis',(1.,0.,0.));
#33324=DIRECTION('center_axis',(0.,0.,1.));
#33325=DIRECTION('ref_axis',(1.,0.,0.));
#33326=DIRECTION('',(0.,0.,-1.));
#33327=DIRECTION('center_axis',(0.,0.,-1.));
#33328=DIRECTION('ref_axis',(1.,0.,0.));
#33329=DIRECTION('',(0.,0.,1.));
#33330=DIRECTION('center_axis',(0.,0.,1.));
#33331=DIRECTION('ref_axis',(1.,0.,0.));
#33332=DIRECTION('center_axis',(-0.259973473447872,-0.96561575852067,0.));
#33333=DIRECTION('ref_axis',(0.96561575852067,-0.259973473447872,0.));
#33334=DIRECTION('',(0.96561575852067,-0.259973473447872,0.));
#33335=DIRECTION('',(0.,0.,1.));
#33336=DIRECTION('center_axis',(-0.259973473447872,0.96561575852067,0.));
#33337=DIRECTION('ref_axis',(-0.96561575852067,-0.259973473447872,0.));
#33338=DIRECTION('',(-0.96561575852067,-0.259973473447872,0.));
#33339=DIRECTION('center_axis',(0.,0.,1.));
#33340=DIRECTION('ref_axis',(1.,0.,0.));
#33341=DIRECTION('center_axis',(0.,0.,-1.));
#33342=DIRECTION('ref_axis',(1.,0.,0.));
#33343=DIRECTION('center_axis',(0.,0.,1.));
#33344=DIRECTION('ref_axis',(1.,0.,0.));
#33345=DIRECTION('',(-0.707106781186548,-8.65956056235493E-17,-0.707106781186547));
#33346=DIRECTION('center_axis',(0.,0.,1.));
#33347=DIRECTION('ref_axis',(1.,0.,0.));
#33348=DIRECTION('',(-0.843867183172891,-1.03343924477817E-16,0.536552119708654));
#33349=DIRECTION('center_axis',(0.,0.,-1.));
#33350=DIRECTION('ref_axis',(1.,0.,0.));
#33351=DIRECTION('center_axis',(0.5,0.866025403784439,0.));
#33352=DIRECTION('ref_axis',(0.866025403784439,-0.5,0.));
#33353=DIRECTION('',(0.866025403784439,-0.5,0.));
#33354=DIRECTION('',(0.,0.,-1.));
#33355=DIRECTION('',(0.866025403784439,-0.5,0.));
#33356=DIRECTION('',(0.,0.,-1.));
#33357=DIRECTION('center_axis',(-0.5,0.866025403784439,0.));
#33358=DIRECTION('ref_axis',(0.866025403784439,0.5,0.));
#33359=DIRECTION('',(0.866025403784439,0.5,0.));
#33360=DIRECTION('',(0.,0.,-1.));
#33361=DIRECTION('',(0.866025403784439,0.5,0.));
#33362=DIRECTION('center_axis',(-1.,-1.20185167898973E-16,0.));
#33363=DIRECTION('ref_axis',(-1.20185167898973E-16,1.,0.));
#33364=DIRECTION('',(-1.20185167898973E-16,1.,0.));
#33365=DIRECTION('',(0.,0.,-1.));
#33366=DIRECTION('',(-1.20185167898973E-16,1.,0.));
#33367=DIRECTION('center_axis',(-0.5,-0.866025403784439,0.));
#33368=DIRECTION('ref_axis',(-0.866025403784439,0.5,0.));
#33369=DIRECTION('',(-0.866025403784439,0.5,0.));
#33370=DIRECTION('',(0.,0.,-1.));
#33371=DIRECTION('',(-0.866025403784439,0.5,0.));
#33372=DIRECTION('center_axis',(0.5,-0.866025403784439,0.));
#33373=DIRECTION('ref_axis',(-0.866025403784439,-0.5,0.));
#33374=DIRECTION('',(-0.866025403784439,-0.5,0.));
#33375=DIRECTION('',(0.,0.,-1.));
#33376=DIRECTION('',(-0.866025403784439,-0.5,0.));
#33377=DIRECTION('center_axis',(1.,-3.60555503696918E-16,0.));
#33378=DIRECTION('ref_axis',(-3.60555503696918E-16,-1.,0.));
#33379=DIRECTION('',(-3.60555503696918E-16,-1.,0.));
#33380=DIRECTION('',(-3.60555503696918E-16,-1.,0.));
#33381=DIRECTION('center_axis',(0.,0.,-1.));
#33382=DIRECTION('ref_axis',(-1.,0.,0.));
#33383=DIRECTION('center_axis',(0.,0.,-1.));
#33384=DIRECTION('ref_axis',(-1.,0.,0.));
#33385=DIRECTION('center_axis',(0.,0.,1.));
#33386=DIRECTION('ref_axis',(1.,0.,0.));
#33387=DIRECTION('center_axis',(0.,0.,1.));
#33388=DIRECTION('ref_axis',(1.,0.,0.));
#33389=DIRECTION('',(0.707106781186548,8.65956056235494E-17,-0.707106781186547));
#33390=DIRECTION('center_axis',(0.,0.,1.));
#33391=DIRECTION('ref_axis',(1.,0.,0.));
#33392=DIRECTION('center_axis',(0.,0.,1.));
#33393=DIRECTION('ref_axis',(1.,0.,0.));
#33394=DIRECTION('',(0.707106781186548,8.65956056235494E-17,-0.707106781186547));
#33395=DIRECTION('center_axis',(0.,0.,-1.));
#33396=DIRECTION('ref_axis',(-1.,0.,0.));
#33397=DIRECTION('center_axis',(0.,0.,1.));
#33398=DIRECTION('ref_axis',(1.,0.,0.));
#48669=CARTESIAN_POINT('',(0.,0.,0.));
#48670=CARTESIAN_POINT('Origin',(0.,0.,-0.29));
#48671=CARTESIAN_POINT('',(-0.121463520633891,0.000103202980665532,-0.514010734985006));
#48672=CARTESIAN_POINT('',(-0.121467053128752,9.34507928307322E-5,-0.520489265014994));
#48673=CARTESIAN_POINT('',(-0.1215,-1.48794586096403E-17,-0.29));
#48674=CARTESIAN_POINT('',(0.0681458046084935,-0.100801883029113,-0.5435));
#48675=CARTESIAN_POINT('Ctrl Pts',(-0.121463520633891,0.000103202980665532,
-0.514010734985006));
#48676=CARTESIAN_POINT('Ctrl Pts',(-0.121553801365528,0.0106198798703647,
-0.514630387130534));
#48677=CARTESIAN_POINT('Ctrl Pts',(-0.120298811423027,0.0211154705696016,
-0.515250039276062));
#48678=CARTESIAN_POINT('Ctrl Pts',(-0.117612982943742,0.0312312632791946,
-0.515869691421591));
#48679=CARTESIAN_POINT('Ctrl Pts',(-0.107390082218629,0.0697343715095162,
-0.518228234573805));
#48680=CARTESIAN_POINT('Ctrl Pts',(-0.0764379898774561,0.102735178047276,
-0.520586777726019));
#48681=CARTESIAN_POINT('Ctrl Pts',(-0.0386628242561016,0.115388802409532,
-0.522945320878233));
#48682=CARTESIAN_POINT('Ctrl Pts',(-0.000887658634747289,0.128042426771789,
-0.525303864030447));
#48683=CARTESIAN_POINT('Ctrl Pts',(0.0437105802667884,0.120348868958541,
-0.527662407182661));
#48684=CARTESIAN_POINT('Ctrl Pts',(0.075062366606055,0.0957822364039557,
-0.530020950334875));
#48685=CARTESIAN_POINT('Ctrl Pts',(0.106414152945322,0.0712156038493702,
-0.532379493487089));
#48686=CARTESIAN_POINT('Ctrl Pts',(0.124519486722319,0.0297758965534469,
-0.534738036639304));
#48687=CARTESIAN_POINT('Ctrl Pts',(0.121273756374489,-0.00993482915230421,
-0.537096579791518));
#48688=CARTESIAN_POINT('Ctrl Pts',(0.118336381625297,-0.0458728986959281,
-0.539231053194345));
#48689=CARTESIAN_POINT('Ctrl Pts',(0.0979120851199604,-0.0803948999064519,
-0.541365526597173));
#48690=CARTESIAN_POINT('Ctrl Pts',(0.0681458046084935,-0.100801883029113,
-0.5435));
#48691=CARTESIAN_POINT('',(-0.1215,-1.48794586096403E-17,-0.5435));
#48692=CARTESIAN_POINT('Origin',(0.,0.,-0.5435));
#48693=CARTESIAN_POINT('',(-0.1215,-1.48794586096403E-17,-0.5735));
#48694=CARTESIAN_POINT('',(-0.1215,-1.48794586096403E-17,-0.29));
#48695=CARTESIAN_POINT('Origin',(0.,0.,-0.5735));
#48696=CARTESIAN_POINT('',(0.121191192277757,-0.00865707307903507,-0.5435));
#48697=CARTESIAN_POINT('Origin',(0.,0.,-0.5435));
#48698=CARTESIAN_POINT('Ctrl Pts',(0.121191192277757,-0.00865707307903506,
-0.5435));
#48699=CARTESIAN_POINT('Ctrl Pts',(0.12404209412111,0.0312529739205125,
-0.541141456847786));
#48700=CARTESIAN_POINT('Ctrl Pts',(0.10563867747241,0.0723480656890973,
-0.538782913695572));
#48701=CARTESIAN_POINT('Ctrl Pts',(0.0740709879443734,0.0965411452271748,
-0.536424370543358));
#48702=CARTESIAN_POINT('Ctrl Pts',(0.0425032984163362,0.120734224765253,
-0.534065827391144));
#48703=CARTESIAN_POINT('Ctrl Pts',(-0.00222866399103803,0.128025292072823,
-0.53170728423893));
#48704=CARTESIAN_POINT('Ctrl Pts',(-0.039883232720534,0.11499262083988,
-0.529348741086716));
#48705=CARTESIAN_POINT('Ctrl Pts',(-0.07753780145003,0.101959949606938,
-0.526990197934502));
#48706=CARTESIAN_POINT('Ctrl Pts',(-0.108114976501648,0.0686035398334826,
-0.524631654782288));
#48707=CARTESIAN_POINT('Ctrl Pts',(-0.117926982101641,0.0299874699351204,
-0.522273111630074));
#48708=CARTESIAN_POINT('Ctrl Pts',(-0.120400700246994,0.0202519197628043,
-0.521678496091714));
#48709=CARTESIAN_POINT('Ctrl Pts',(-0.121554581285855,0.0101820648492457,
-0.521083880553354));
#48710=CARTESIAN_POINT('Ctrl Pts',(-0.121467053128752,9.34507928307322E-5,
-0.520489265014994));
#48711=CARTESIAN_POINT('Origin',(0.,0.,-0.29));
#48712=CARTESIAN_POINT('',(-0.121354988926872,-7.09400307492836E-5,-0.469010734985006));
#48713=CARTESIAN_POINT('',(-0.121347519425042,-6.58635799960141E-5,-0.475489265014995));
#48714=CARTESIAN_POINT('',(-0.1215,-1.48794586096403E-17,-0.29));
#48715=CARTESIAN_POINT('Ctrl Pts',(-0.121354988926872,-7.09400307492836E-5,
-0.469010734985006));
#48716=CARTESIAN_POINT('Ctrl Pts',(-0.121219195033693,0.0249081254717452,
-0.47047912821725));
#48717=CARTESIAN_POINT('Ctrl Pts',(-0.113699226119619,0.0499622036482225,
-0.471947521449495));
#48718=CARTESIAN_POINT('Ctrl Pts',(-0.0993881694574734,0.0702183410582727,
-0.473415914681739));
#48719=CARTESIAN_POINT('Ctrl Pts',(-0.0764016533456638,0.102753886121886,
-0.475774457833953));
#48720=CARTESIAN_POINT('Ctrl Pts',(-0.0358948086527237,0.12291122288382,
-0.478133000986166));
#48721=CARTESIAN_POINT('Ctrl Pts',(0.00392099239580886,0.121627591643135,
-0.48049154413838));
#48722=CARTESIAN_POINT('Ctrl Pts',(0.0437367934443413,0.12034396040245,
-0.482850087290594));
#48723=CARTESIAN_POINT('Ctrl Pts',(0.0828615508484662,0.0976193611591442,
-0.485208630442808));
#48724=CARTESIAN_POINT('Ctrl Pts',(0.103704668945383,0.0636709283798785,
-0.487567173595023));
#48725=CARTESIAN_POINT('Ctrl Pts',(0.1245477870423,0.0297224956006128,-0.489925716747237));
#48726=CARTESIAN_POINT('Ctrl Pts',(0.127109265832009,-0.0154497707146136,
-0.492284259899451));
#48727=CARTESIAN_POINT('Ctrl Pts',(0.110238229460948,-0.0515373638505048,
-0.494642803051665));
#48728=CARTESIAN_POINT('Ctrl Pts',(0.0933671930898881,-0.0876249569863961,
-0.497001346203878));
#48729=CARTESIAN_POINT('Ctrl Pts',(0.0570636415580583,-0.114627876942952,
-0.499359889356092));
#48730=CARTESIAN_POINT('Ctrl Pts',(0.0176479671399454,-0.120404648237461,
-0.501718432508307));
#48731=CARTESIAN_POINT('Ctrl Pts',(-0.0217677072781677,-0.12618141953197,
-0.504076975660521));
#48732=CARTESIAN_POINT('Ctrl Pts',(-0.0642955045825639,-0.110732042164432,
-0.506435518812735));
#48733=CARTESIAN_POINT('Ctrl Pts',(-0.0908125486802356,-0.0810046485192209,
-0.508794061964949));
#48734=CARTESIAN_POINT('Ctrl Pts',(-0.110362858566254,-0.0590874334734252,
-0.510532952971635));
#48735=CARTESIAN_POINT('Ctrl Pts',(-0.121210171471051,-0.0294090887069978,
-0.51227184397832));
#48736=CARTESIAN_POINT('Ctrl Pts',(-0.121463520633891,0.000103202980665532,
-0.514010734985006));
#48737=CARTESIAN_POINT('Ctrl Pts',(-0.121467053128752,9.34507928307322E-5,
-0.520489265014994));
#48738=CARTESIAN_POINT('Ctrl Pts',(-0.121207400759546,-0.029834433313122,
-0.51872533740114));
#48739=CARTESIAN_POINT('Ctrl Pts',(-0.110023188032426,-0.0599274002854349,
-0.516961409787286));
#48740=CARTESIAN_POINT('Ctrl Pts',(-0.0899618218360895,-0.0819479460585449,
-0.515197482173432));
#48741=CARTESIAN_POINT('Ctrl Pts',(-0.0631378198221754,-0.111391562130578,
-0.512838939021217));
#48742=CARTESIAN_POINT('Ctrl Pts',(-0.0204429796459781,-0.126403064251376,
-0.510480395869004));
#48743=CARTESIAN_POINT('Ctrl Pts',(0.0189116888966024,-0.120215378421974,
-0.508121852716789));
#48744=CARTESIAN_POINT('Ctrl Pts',(0.0582663574391833,-0.114027692592572,
-0.505763309564575));
#48745=CARTESIAN_POINT('Ctrl Pts',(0.0942808543481472,-0.0866408188129685,
-0.503404766412361));
#48746=CARTESIAN_POINT('Ctrl Pts',(0.110771590337775,-0.0503771654710377,
-0.501046223260147));
#48747=CARTESIAN_POINT('Ctrl Pts',(0.127262326327404,-0.0141135121291072,
-0.498687680107933));
#48748=CARTESIAN_POINT('Ctrl Pts',(0.124229301397696,0.031026920775151,
-0.496329136955719));
#48749=CARTESIAN_POINT('Ctrl Pts',(0.103031791863172,0.0647543130122383,
-0.493970593803505));
#48750=CARTESIAN_POINT('Ctrl Pts',(0.0818342823286479,0.0984817052493257,
-0.491612050651291));
#48751=CARTESIAN_POINT('Ctrl Pts',(0.0424722881893066,0.120796056819242,
-0.489253507499077));
#48752=CARTESIAN_POINT('Ctrl Pts',(0.00264496221188506,0.121662374236399,
-0.486894964346863));
#48753=CARTESIAN_POINT('Ctrl Pts',(-0.0371823637655362,0.122528691653556,
-0.484536421194649));
#48754=CARTESIAN_POINT('Ctrl Pts',(-0.0774750215810378,0.101946974917955,
-0.482177878042435));
#48755=CARTESIAN_POINT('Ctrl Pts',(-0.100118934895602,0.0691719947505057,
-0.479819334890221));
#48756=CARTESIAN_POINT('Ctrl Pts',(-0.113976320659153,0.0491147044198212,
-0.478375978265146));
#48757=CARTESIAN_POINT('Ctrl Pts',(-0.121224132521449,0.0244909546593463,
-0.47693262164007));
#48758=CARTESIAN_POINT('Ctrl Pts',(-0.121347519425042,-6.58635799960141E-5,
-0.475489265014995));
#48759=CARTESIAN_POINT('Origin',(0.,0.,-0.29));
#48760=CARTESIAN_POINT('',(-0.121689032810886,-1.25051776863616E-5,-0.424010734985006));
#48761=CARTESIAN_POINT('',(-0.121686438635927,-1.99743996858978E-5,-0.430489265014994));
#48762=CARTESIAN_POINT('',(-0.1215,-1.48794586096403E-17,-0.29));
#48763=CARTESIAN_POINT('Ctrl Pts',(-0.121689032810886,-1.25051776863616E-5,
-0.424010734985006));
#48764=CARTESIAN_POINT('Ctrl Pts',(-0.121630741701287,0.0391259959765282,
-0.426327869303966));
#48765=CARTESIAN_POINT('Ctrl Pts',(-0.101028394996106,0.0783173256670956,
-0.428645003622925));
#48766=CARTESIAN_POINT('Ctrl Pts',(-0.0687315757637827,0.10042212870287,
-0.430962137941885));
#48767=CARTESIAN_POINT('Ctrl Pts',(-0.0358575894715735,0.122921960242402,
-0.4333206810941));
#48768=CARTESIAN_POINT('Ctrl Pts',(0.00913258115290106,0.12771911164248,
-0.435679224246314));
#48769=CARTESIAN_POINT('Ctrl Pts',(0.0460116911221716,0.112656815349134,
-0.438037767398528));
#48770=CARTESIAN_POINT('Ctrl Pts',(0.0828908010914419,0.0975945190557874,
-0.440396310550742));
#48771=CARTESIAN_POINT('Ctrl Pts',(0.111658850405508,0.0626727750690164,
-0.442754853702956));
#48772=CARTESIAN_POINT('Ctrl Pts',(0.119381927578032,0.0235921491730332,
-0.44511339685517));
#48773=CARTESIAN_POINT('Ctrl Pts',(0.127105004750555,-0.01548847672295,
-0.447471940007384));
#48774=CARTESIAN_POINT('Ctrl Pts',(0.113783109781535,-0.0587279845281455,
-0.449830483159598));
#48775=CARTESIAN_POINT('Ctrl Pts',(0.0854056844396275,-0.0866862229885438,
-0.452189026311812));
#48776=CARTESIAN_POINT('Ctrl Pts',(0.05702825909772,-0.114644461448942,
-0.454547569464026));
#48777=CARTESIAN_POINT('Ctrl Pts',(0.0135953033829249,-0.127321430564543,
-0.45690611261624));
#48778=CARTESIAN_POINT('Ctrl Pts',(-0.025366075857601,-0.11901763363164,
-0.459264655768454));
#48779=CARTESIAN_POINT('Ctrl Pts',(-0.064327455098127,-0.110713836698737,
-0.461623198920668));
#48780=CARTESIAN_POINT('Ctrl Pts',(-0.0988172578643837,-0.08142927371733,
-0.463981742072882));
#48781=CARTESIAN_POINT('Ctrl Pts',(-0.113329065482173,-0.0443301155439809,
-0.466340285225096));
#48782=CARTESIAN_POINT('Ctrl Pts',(-0.118806041545752,-0.0303283311594296,
-0.467230435145066));
#48783=CARTESIAN_POINT('Ctrl Pts',(-0.121437308104386,-0.0152134186731973,
-0.468120585065036));
#48784=CARTESIAN_POINT('Ctrl Pts',(-0.121354988926872,-7.09400307492836E-5,
-0.469010734985006));
#48785=CARTESIAN_POINT('Ctrl Pts',(-0.121347519425042,-6.58635799960141E-5,
-0.475489265014995));
#48786=CARTESIAN_POINT('Ctrl Pts',(-0.121425755136045,-0.0156365609472264,
-0.474574078487856));
#48787=CARTESIAN_POINT('Ctrl Pts',(-0.118639669415141,-0.0311803490001526,
-0.473658891960718));
#48788=CARTESIAN_POINT('Ctrl Pts',(-0.112858015223634,-0.0455160728540226,
-0.472743705433579));
#48789=CARTESIAN_POINT('Ctrl Pts',(-0.0979580134234747,-0.0824609166918042,
-0.470385162281365));
#48790=CARTESIAN_POINT('Ctrl Pts',(-0.063162841009528,-0.11138236076807,
-0.46802661912915));
#48791=CARTESIAN_POINT('Ctrl Pts',(-0.0241164856398025,-0.119277153472215,
-0.465668075976936));
#48792=CARTESIAN_POINT('Ctrl Pts',(0.0149298697299233,-0.12717194617636,
-0.463309532824722));
#48793=CARTESIAN_POINT('Ctrl Pts',(0.0582274080554279,-0.114040087508383,
-0.460950989672509));
#48794=CARTESIAN_POINT('Ctrl Pts',(0.0863100510388977,-0.0857857662793123,
-0.458592446520295));
#48795=CARTESIAN_POINT('Ctrl Pts',(0.114392694022367,-0.0575314450502418,
-0.456233903368081));
#48796=CARTESIAN_POINT('Ctrl Pts',(0.127260441663802,-0.0141546612600778,
-0.453875360215866));
#48797=CARTESIAN_POINT('Ctrl Pts',(0.11912795666395,0.0248428088327164,
-0.451516817063652));
#48798=CARTESIAN_POINT('Ctrl Pts',(0.110995471664098,0.0638402789255106,
-0.449158273911438));
#48799=CARTESIAN_POINT('Ctrl Pts',(0.0818627540229589,0.0984584353209352,
-0.446799730759224));
#48800=CARTESIAN_POINT('Ctrl Pts',(0.0448277078769713,0.113133153866057,
-0.44444118760701));
#48801=CARTESIAN_POINT('Ctrl Pts',(0.00779266173098367,0.127807872411178,
-0.442082644454797));
#48802=CARTESIAN_POINT('Ctrl Pts',(-0.0371447129198525,0.122539153105997,
-0.439724101302582));
#48803=CARTESIAN_POINT('Ctrl Pts',(-0.0697809290729632,0.0996958028250744,
-0.437365558150368));
#48804=CARTESIAN_POINT('Ctrl Pts',(-0.101497709957742,0.0774960008585949,
-0.435073460438577));
#48805=CARTESIAN_POINT('Ctrl Pts',(-0.121596671566893,0.0386978527648168,
-0.432781362726786));
#48806=CARTESIAN_POINT('Ctrl Pts',(-0.121686438635927,-1.99743996858978E-5,
-0.430489265014994));
#48807=CARTESIAN_POINT('Origin',(0.,0.,-0.29));
#48808=CARTESIAN_POINT('',(-0.121383410361094,8.5849798153903E-5,-0.379010734985006));
#48809=CARTESIAN_POINT('',(-0.121393079482962,8.9638819514881E-5,-0.385489265014994));
#48810=CARTESIAN_POINT('',(-0.1215,-1.48794586096403E-17,-0.29));
#48811=CARTESIAN_POINT('Ctrl Pts',(-0.121383410361094,8.5849798153903E-5,
-0.379010734985006));
#48812=CARTESIAN_POINT('Ctrl Pts',(-0.121475175728008,0.0138114136519433,
-0.379818067238468));
#48813=CARTESIAN_POINT('Ctrl Pts',(-0.119322368561901,0.0275090559256997,
-0.380625399491929));
#48814=CARTESIAN_POINT('Ctrl Pts',(-0.114798393001489,0.0403727954403562,
-0.381432731745391));
#48815=CARTESIAN_POINT('Ctrl Pts',(-0.101582035630596,0.0779529671900597,
-0.383791274897605));
#48816=CARTESIAN_POINT('Ctrl Pts',(-0.0681287102894151,0.108416114494445,
-0.386149818049819));
#48817=CARTESIAN_POINT('Ctrl Pts',(-0.0294787857423598,0.118066230703992,
-0.388508361202033));
#48818=CARTESIAN_POINT('Ctrl Pts',(0.00917113880469548,0.127716346913539,
-0.390866904354247));
#48819=CARTESIAN_POINT('Ctrl Pts',(0.0530176625576257,0.116553432028247,
-0.393225447506461));
#48820=CARTESIAN_POINT('Ctrl Pts',(0.0823477114274472,0.0895962502971781,
-0.395583990658675));
#48821=CARTESIAN_POINT('Ctrl Pts',(0.111677760297269,0.0626390685661086,
-0.397942533810889));
#48822=CARTESIAN_POINT('Ctrl Pts',(0.126491334283982,0.0198876199892615,
-0.400301076963103));
#48823=CARTESIAN_POINT('Ctrl Pts',(0.120128359435606,-0.0194373588391155,
-0.402659620115317));
#48824=CARTESIAN_POINT('Ctrl Pts',(0.11376538458723,-0.0587623376674924,
-0.405018163267531));
#48825=CARTESIAN_POINT('Ctrl Pts',(0.0862258609037655,-0.0946608467473989,
-0.407376706419745));
#48826=CARTESIAN_POINT('Ctrl Pts',(0.049891355764218,-0.110993181039425,
-0.409735249571959));
#48827=CARTESIAN_POINT('Ctrl Pts',(0.0135568506246707,-0.127325515331451,
-0.412093792724173));
#48828=CARTESIAN_POINT('Ctrl Pts',(-0.0315726359709597,-0.124091674835596,
-0.414452335876387));
#48829=CARTESIAN_POINT('Ctrl Pts',(-0.0652072198369896,-0.102745569896818,
-0.416810879028601));
#48830=CARTESIAN_POINT('Ctrl Pts',(-0.0988418037030196,-0.0813994649580399,
-0.419169422180815));
#48831=CARTESIAN_POINT('Ctrl Pts',(-0.120981484839449,-0.0419410955763378,
-0.421527965333029));
#48832=CARTESIAN_POINT('Ctrl Pts',(-0.121672424427692,-0.00211065504599355,
-0.423886508485243));
#48833=CARTESIAN_POINT('Ctrl Pts',(-0.12168455522215,-0.00141135384015577,
-0.423927917318497));
#48834=CARTESIAN_POINT('Ctrl Pts',(-0.121690074514347,-0.000711937944640976,
-0.423969326151752));
#48835=CARTESIAN_POINT('Ctrl Pts',(-0.121689032810886,-1.25051776863616E-5,
-0.424010734985006));
#48836=CARTESIAN_POINT('Ctrl Pts',(-0.121686438635927,-1.99743996858978E-5,
-0.430489265014994));
#48837=CARTESIAN_POINT('Ctrl Pts',(-0.121689040886436,-0.00114236244838274,
-0.430422819574572));
#48838=CARTESIAN_POINT('Ctrl Pts',(-0.121674828258958,-0.0022646829987791,
-0.430356374134149));
#48839=CARTESIAN_POINT('Ctrl Pts',(-0.121643596330701,-0.00338652974087634,
-0.430289928693726));
#48840=CARTESIAN_POINT('Ctrl Pts',(-0.120534989779944,-0.0432075307692407,
-0.427931385541512));
#48841=CARTESIAN_POINT('Ctrl Pts',(-0.0979827190230435,-0.0824315515693056,
-0.425572842389298));
#48842=CARTESIAN_POINT('Ctrl Pts',(-0.0641261260412589,-0.103423753071392,
-0.423214299237084));
#48843=CARTESIAN_POINT('Ctrl Pts',(-0.030269533059474,-0.124415954573479,
-0.42085575608487));
#48844=CARTESIAN_POINT('Ctrl Pts',(0.0148913821471955,-0.127176336777588,
-0.418497212932656));
#48845=CARTESIAN_POINT('Ctrl Pts',(0.051052608431988,-0.110463856476749,
-0.416138669780442));
#48846=CARTESIAN_POINT('Ctrl Pts',(0.0872138347167803,-0.0937513761759113,
-0.413780126628228));
#48847=CARTESIAN_POINT('Ctrl Pts',(0.114375372079696,-0.0575660333701267,
-0.411421583476013));
#48848=CARTESIAN_POINT('Ctrl Pts',(0.120325591369617,-0.0181764894408694,
-0.409063040323799));
#48849=CARTESIAN_POINT('Ctrl Pts',(0.126275810659539,0.0212130544883879,
-0.406704497171585));
#48850=CARTESIAN_POINT('Ctrl Pts',(0.111014711876466,0.0638067995411181,
-0.404345954019372));
#48851=CARTESIAN_POINT('Ctrl Pts',(0.0814035736878408,0.0904549104188703,
-0.401987410867158));
#48852=CARTESIAN_POINT('Ctrl Pts',(0.0517924354992152,0.117103021296623,
-0.399628867714944));
#48853=CARTESIAN_POINT('Ctrl Pts',(0.00783125790503672,0.127805497999397,
-0.397270324562729));
#48854=CARTESIAN_POINT('Ctrl Pts',(-0.0307153379373213,0.117750586445704,
-0.394911781410515));
#48855=CARTESIAN_POINT('Ctrl Pts',(-0.0692619337796792,0.107695674892012,
-0.392553238258301));
#48856=CARTESIAN_POINT('Ctrl Pts',(-0.102393947870216,0.0768833750818523,
-0.390194695106087));
#48857=CARTESIAN_POINT('Ctrl Pts',(-0.115215470377363,0.0391666697696868,
-0.387836151953873));
#48858=CARTESIAN_POINT('Ctrl Pts',(-0.119468189360593,0.0266565682137656,
-0.38705385630758));
#48859=CARTESIAN_POINT('Ctrl Pts',(-0.121486437931333,0.0133868745156882,
-0.386271560661287));
#48860=CARTESIAN_POINT('Ctrl Pts',(-0.121393079482962,8.9638819514881E-5,
-0.385489265014994));
#48861=CARTESIAN_POINT('Origin',(0.,0.,-0.29));
#48862=CARTESIAN_POINT('',(-0.121426763094784,-9.9191016992628E-5,-0.334010734985006));
#48863=CARTESIAN_POINT('',(-0.121415770900973,-9.66275040455964E-5,-0.340489265014995));
#48864=CARTESIAN_POINT('',(-0.1215,-1.48794586096403E-17,-0.29));
#48865=CARTESIAN_POINT('Ctrl Pts',(-0.121426763094784,-9.9191016992628E-5,
-0.334010734985006));
#48866=CARTESIAN_POINT('Ctrl Pts',(-0.121203576807245,0.0280304944041191,
-0.335666808325183));
#48867=CARTESIAN_POINT('Ctrl Pts',(-0.111451175585138,0.0562998709178246,
-0.337322881665361));
#48868=CARTESIAN_POINT('Ctrl Pts',(-0.0935666813062145,0.0778068749824484,
-0.338978955005538));
#48869=CARTESIAN_POINT('Ctrl Pts',(-0.0680959787177338,0.108436676169773,
-0.341337498157752));
#48870=CARTESIAN_POINT('Ctrl Pts',(-0.0261310911381096,0.125350473202342,
-0.343696041309966));
#48871=CARTESIAN_POINT('Ctrl Pts',(0.0134608770154306,0.120943947492484,
-0.34605458446218));
#48872=CARTESIAN_POINT('Ctrl Pts',(0.0530528451689708,0.116537421782626,
-0.348413127614394));
#48873=CARTESIAN_POINT('Ctrl Pts',(0.0902718938964271,0.0908105733303415,
-0.350771670766608));
#48874=CARTESIAN_POINT('Ctrl Pts',(0.10838461298205,0.0553300037393775,
-0.353130213918822));
#48875=CARTESIAN_POINT('Ctrl Pts',(0.126497332067673,0.0198494341484135,
-0.355488757071036));
#48876=CARTESIAN_POINT('Ctrl Pts',(0.125503721511462,-0.02538485658123,
-0.35784730022325));
#48877=CARTESIAN_POINT('Ctrl Pts',(0.105850501298503,-0.0600358644506952,
-0.360205843375464));
#48878=CARTESIAN_POINT('Ctrl Pts',(0.0861972810855425,-0.0946868723201607,
-0.362564386527678));
#48879=CARTESIAN_POINT('Ctrl Pts',(0.0478844512158326,-0.118754597329448,
-0.364922929679892));
#48880=CARTESIAN_POINT('Ctrl Pts',(0.00813717786102508,-0.121418367560867,
-0.367281472832106));
#48881=CARTESIAN_POINT('Ctrl Pts',(-0.0316100954937825,-0.124082137792286,
-0.369640015984321));
#48882=CARTESIAN_POINT('Ctrl Pts',(-0.0727918123336877,-0.105341953245838,
-0.371998559136535));
#48883=CARTESIAN_POINT('Ctrl Pts',(-0.0968929760533375,-0.0736232628751029,
-0.374357102288749));
#48884=CARTESIAN_POINT('Ctrl Pts',(-0.112744281465937,-0.0527619196552203,
-0.375908313187501));
#48885=CARTESIAN_POINT('Ctrl Pts',(-0.12120709207742,-0.0262864946117645,
-0.377459524086254));
#48886=CARTESIAN_POINT('Ctrl Pts',(-0.121383410361094,8.5849798153903E-5,
-0.379010734985006));
#48887=CARTESIAN_POINT('Ctrl Pts',(-0.121393079482962,8.9638819514881E-5,
-0.385489265014994));
#48888=CARTESIAN_POINT('Ctrl Pts',(-0.121204971544359,-0.0267029615241794,
-0.383913017509073));
#48889=CARTESIAN_POINT('Ctrl Pts',(-0.112444114863846,-0.0536073774791074,
-0.382336770003152));
#48890=CARTESIAN_POINT('Ctrl Pts',(-0.0961155486467309,-0.0746353396772124,
-0.380760522497231));
#48891=CARTESIAN_POINT('Ctrl Pts',(-0.0716830734851945,-0.106099532997775,
-0.378401979345017));
#48892=CARTESIAN_POINT('Ctrl Pts',(-0.0303070922383648,-0.124406808824729,
-0.376043436192803));
#48893=CARTESIAN_POINT('Ctrl Pts',(0.00941005870800238,-0.121326350857264,
-0.373684893040589));
#48894=CARTESIAN_POINT('Ctrl Pts',(0.0491272096543692,-0.118245892889799,
-0.371326349888375));
#48895=CARTESIAN_POINT('Ctrl Pts',(0.0871855303002735,-0.0937777011279164,
-0.368967806736161));
#48896=CARTESIAN_POINT('Ctrl Pts',(0.106474279911884,-0.0589224943497298,
-0.366609263583947));
#48897=CARTESIAN_POINT('Ctrl Pts',(0.125763029523496,-0.0240672875715429,
-0.364250720431733));
#48898=CARTESIAN_POINT('Ctrl Pts',(0.126282208100813,0.0211749342229483,
-0.361892177279519));
#48899=CARTESIAN_POINT('Ctrl Pts',(0.107798396801026,0.0564636012642046,
-0.359533634127305));
#48900=CARTESIAN_POINT('Ctrl Pts',(0.0893145855012401,0.0917522683054609,
-0.357175090975091));
#48901=CARTESIAN_POINT('Ctrl Pts',(0.0518277843243512,0.117087380593482,
-0.354816547822877));
#48902=CARTESIAN_POINT('Ctrl Pts',(0.0121917830058918,0.121078458230895,
-0.352458004670663));
#48903=CARTESIAN_POINT('Ctrl Pts',(-0.0274442183125677,0.125069535868307,
-0.350099461518449));
#48904=CARTESIAN_POINT('Ctrl Pts',(-0.0692294197725976,0.107716578855109,
-0.347740918366234));
#48905=CARTESIAN_POINT('Ctrl Pts',(-0.0943775025079859,0.076821348865989,
-0.34538237521402));
#48906=CARTESIAN_POINT('Ctrl Pts',(-0.111768512152077,0.0554559331263187,
-0.343751338481012));
#48907=CARTESIAN_POINT('Ctrl Pts',(-0.121203097283924,0.0276141512297166,
-0.342120301748003));
#48908=CARTESIAN_POINT('Ctrl Pts',(-0.121415770900973,-9.66275040455964E-5,
-0.340489265014995));
#48909=CARTESIAN_POINT('Origin',(0.,0.,-0.29));
#48910=CARTESIAN_POINT('',(-0.121671190739018,4.27946393402705E-5,-0.289010734985006));
#48911=CARTESIAN_POINT('',(-0.12167703567116,3.58475784977506E-5,-0.295489265014995));
#48912=CARTESIAN_POINT('',(-0.1215,-1.48794586096403E-17,-0.29));
#48913=CARTESIAN_POINT('Ctrl Pts',(-0.121671190739018,4.27946393402705E-5,
-0.289010734985006));
#48914=CARTESIAN_POINT('Ctrl Pts',(-0.121682586494413,0.00251441956358687,
-0.289157006259685));
#48915=CARTESIAN_POINT('Ctrl Pts',(-0.121613663427898,0.00498539735850438,
-0.289303277534364));
#48916=CARTESIAN_POINT('Ctrl Pts',(-0.121462386894709,0.00745132303565125,
-0.289449548809043));
#48917=CARTESIAN_POINT('Ctrl Pts',(-0.119023136725957,0.0472130064725989,
-0.291808091961257));
#48918=CARTESIAN_POINT('Ctrl Pts',(-0.0951721719288084,0.0856611507430487,
-0.294166635113471));
#48919=CARTESIAN_POINT('Ctrl Pts',(-0.0606327106317513,0.105509753324465,
-0.296525178265685));
#48920=CARTESIAN_POINT('Ctrl Pts',(-0.0260932493346944,0.125358355905882,
-0.298883721417899));
#48921=CARTESIAN_POINT('Ctrl Pts',(0.0191347084622706,0.126607416798265,
-0.301242264570113));
#48922=CARTESIAN_POINT('Ctrl Pts',(0.0547170060032727,0.108695367422808,
-0.303600807722327));
#48923=CARTESIAN_POINT('Ctrl Pts',(0.0902993035442753,0.0907833180473516,
-0.305959350874541));
#48924=CARTESIAN_POINT('Ctrl Pts',(0.116235940829315,0.0537101584040538,
-0.308317894026755));
#48925=CARTESIAN_POINT('Ctrl Pts',(0.120865996738776,0.0141437080527541,
-0.310676437178969));
#48926=CARTESIAN_POINT('Ctrl Pts',(0.125496052648237,-0.0254227422985456,
-0.313034980331183));
#48927=CARTESIAN_POINT('Ctrl Pts',(0.10881952718212,-0.0674824833578473,
-0.315393523483397));
#48928=CARTESIAN_POINT('Ctrl Pts',(0.078334063379927,-0.0931257652829706,
-0.317752066635612));
#48929=CARTESIAN_POINT('Ctrl Pts',(0.0478485995777338,-0.118769047208094,
-0.320110609787826));
#48930=CARTESIAN_POINT('Ctrl Pts',(0.00355419743946411,-0.127995869999039,
-0.32246915294004));
#48931=CARTESIAN_POINT('Ctrl Pts',(-0.0346347060280981,-0.116657922077687,
-0.324827696092254));
#48932=CARTESIAN_POINT('Ctrl Pts',(-0.0728236094956603,-0.105319974156336,
-0.327186239244468));
#48933=CARTESIAN_POINT('Ctrl Pts',(-0.104907014292515,-0.0734172555226875,
-0.329544782396682));
#48934=CARTESIAN_POINT('Ctrl Pts',(-0.116460457892274,-0.0352929935348227,
-0.331903325548896));
#48935=CARTESIAN_POINT('Ctrl Pts',(-0.119901541998062,-0.0239380420142126,
-0.332605795360932));
#48936=CARTESIAN_POINT('Ctrl Pts',(-0.121521433799066,-0.0120311836111781,
-0.333308265172969));
#48937=CARTESIAN_POINT('Ctrl Pts',(-0.121426763094784,-9.9191016992628E-5,
-0.334010734985006));
#48938=CARTESIAN_POINT('Ctrl Pts',(-0.121415770900973,-9.66275040455964E-5,
-0.340489265014995));
#48939=CARTESIAN_POINT('Ctrl Pts',(-0.121510631683975,-0.012456722774741,
-0.339761758595789));
#48940=CARTESIAN_POINT('Ctrl Pts',(-0.119770783742297,-0.0247907548322472,
-0.339034252176584));
#48941=CARTESIAN_POINT('Ctrl Pts',(-0.116083927801042,-0.0365123859409015,
-0.338306745757379));
#48942=CARTESIAN_POINT('Ctrl Pts',(-0.104131306347963,-0.0745133877936318,
-0.335948202605165));
#48943=CARTESIAN_POINT('Ctrl Pts',(-0.0717150994310587,-0.106077888534051,
-0.33358965945295));
#48944=CARTESIAN_POINT('Ctrl Pts',(-0.0334093949576405,-0.117014721079873,
-0.331231116300736));
#48945=CARTESIAN_POINT('Ctrl Pts',(0.00489630951577786,-0.127951553625695,
-0.328872573148522));
#48946=CARTESIAN_POINT('Ctrl Pts',(0.0490915115457099,-0.11826071797692,
-0.326514029996308));
#48947=CARTESIAN_POINT('Ctrl Pts',(0.0793063737628009,-0.0922991424745387,
-0.324155486844094));
#48948=CARTESIAN_POINT('Ctrl Pts',(0.109521235979892,-0.0663375669721578,
-0.32179694369188));
#48949=CARTESIAN_POINT('Ctrl Pts',(0.125755758384142,-0.0241052516161715,
-0.319438400539666));
#48950=CARTESIAN_POINT('Ctrl Pts',(0.12071101925804,0.0154104656178542,
-0.317079857387452));
#48951=CARTESIAN_POINT('Ctrl Pts',(0.115666280131938,0.0549261828518797,
-0.314721314235238));
#48952=CARTESIAN_POINT('Ctrl Pts',(0.0893422794754841,0.0917253019639447,
-0.312362771083024));
#48953=CARTESIAN_POINT('Ctrl Pts',(0.0535740941272359,0.109263209999201,
-0.31000422793081));
#48954=CARTESIAN_POINT('Ctrl Pts',(0.0178059087789875,0.126801118034458,
-0.307645684778596));
#48955=CARTESIAN_POINT('Ctrl Pts',(-0.0274064612610546,0.125077814992907,
-0.305287141626382));
#48956=CARTESIAN_POINT('Ctrl Pts',(-0.0617358673776313,0.104868085231056,
-0.302928598474168));
#48957=CARTESIAN_POINT('Ctrl Pts',(-0.0960652734942078,0.0846583554692045,
-0.300570055321954));
#48958=CARTESIAN_POINT('Ctrl Pts',(-0.119511715687319,0.0459621989870536,
-0.29821151216974));
#48959=CARTESIAN_POINT('Ctrl Pts',(-0.121533846212305,0.00617712277116327,
-0.295852969017526));
#48960=CARTESIAN_POINT('Ctrl Pts',(-0.121637788479221,0.00413207624217357,
-0.295731734350015));
#48961=CARTESIAN_POINT('Ctrl Pts',(-0.121685123389425,0.00208415256740887,
-0.295610499682505));
#48962=CARTESIAN_POINT('Ctrl Pts',(-0.12167703567116,3.58475784977506E-5,
-0.295489265014995));
#48963=CARTESIAN_POINT('Origin',(0.,0.,-0.29));
#48964=CARTESIAN_POINT('',(-0.121328086182402,4.76889891967633E-5,-0.244010734985006));
#48965=CARTESIAN_POINT('',(-0.121333512465724,5.36033326936202E-5,-0.250489265014994));
#48966=CARTESIAN_POINT('',(-0.1215,-1.48794586096403E-17,-0.29));
#48967=CARTESIAN_POINT('Ctrl Pts',(-0.121328086182402,4.76889891967633E-5,
-0.244010734985006));
#48968=CARTESIAN_POINT('Ctrl Pts',(-0.121389094799374,0.0169834435373647,
-0.245005747346401));
#48969=CARTESIAN_POINT('Ctrl Pts',(-0.118076715360543,0.0338963940472306,
-0.246000759707796));
#48970=CARTESIAN_POINT('Ctrl Pts',(-0.111273178531525,0.0492637126557456,
-0.24699577206919));
#48971=CARTESIAN_POINT('Ctrl Pts',(-0.0951463083322207,0.085689877272637,
-0.249354315221404));
#48972=CARTESIAN_POINT('Ctrl Pts',(-0.0594039044238847,0.113431702779544,
-0.251712858373618));
#48973=CARTESIAN_POINT('Ctrl Pts',(-0.0201154883879651,0.120016668725902,
-0.254071401525832));
#48974=CARTESIAN_POINT('Ctrl Pts',(0.0191729276479541,0.126601634672261,
-0.256429944678046));
#48975=CARTESIAN_POINT('Ctrl Pts',(0.0620073558114569,0.112029741058072,
-0.25878848783026));
#48976=CARTESIAN_POINT('Ctrl Pts',(0.0891297526433666,0.0828524039414163,
-0.261147030982474));
#48977=CARTESIAN_POINT('Ctrl Pts',(0.116252149475276,0.0536750668247602,
-0.263505574134689));
#48978=CARTESIAN_POINT('Ctrl Pts',(0.127662514975593,0.00989228620563701,
-0.265864117286902));
#48979=CARTESIAN_POINT('Ctrl Pts',(0.118230832844077,-0.028811522176682,
-0.268222660439116));
#48980=CARTESIAN_POINT('Ctrl Pts',(0.108799150712561,-0.067515330559001,
-0.270581203591331));
#48981=CARTESIAN_POINT('Ctrl Pts',(0.0785254209492124,-0.101140166704516,
-0.272939746743545));
#48982=CARTESIAN_POINT('Ctrl Pts',(0.0410204895125326,-0.114568551903633,
-0.275298289895759));
#48983=CARTESIAN_POINT('Ctrl Pts',(0.00351555807585251,-0.12799693710275,
-0.277656833047973));
#48984=CARTESIAN_POINT('Ctrl Pts',(-0.0412205750341589,-0.121228871355469,
-0.280015376200187));
#48985=CARTESIAN_POINT('Ctrl Pts',(-0.0730748738189873,-0.0973072271801054,
-0.282373919352401));
#48986=CARTESIAN_POINT('Ctrl Pts',(-0.102953644243061,-0.0748691468660444,
-0.284586191229936));
#48987=CARTESIAN_POINT('Ctrl Pts',(-0.121498836261088,-0.0373391610708751,
-0.286798463107471));
#48988=CARTESIAN_POINT('Ctrl Pts',(-0.121671190739018,4.27946393402705E-5,
-0.289010734985006));
#48989=CARTESIAN_POINT('Ctrl Pts',(-0.12167703567116,3.58475784977506E-5,
-0.295489265014995));
#48990=CARTESIAN_POINT('Ctrl Pts',(-0.121527781987638,-0.0377643149085251,
-0.293251956530291));
#48991=CARTESIAN_POINT('Ctrl Pts',(-0.102503604523412,-0.0756943390720712,
-0.291014648045587));
#48992=CARTESIAN_POINT('Ctrl Pts',(-0.0720503805424354,-0.0980682175048509,
-0.288777339560883));
#48993=CARTESIAN_POINT('Ctrl Pts',(-0.0399469654907172,-0.121654485615344,
-0.286418796408669));
#48994=CARTESIAN_POINT('Ctrl Pts',(0.00485768346958088,-0.127953025886699,
-0.284060253256455));
#48995=CARTESIAN_POINT('Ctrl Pts',(0.0422197261182076,-0.114132060996872,
-0.281701710104241));
#48996=CARTESIAN_POINT('Ctrl Pts',(0.0795817687668341,-0.100311096107045,
-0.279343166952027));
#48997=CARTESIAN_POINT('Ctrl Pts',(0.109501205103789,-0.0663706260560358,
-0.276984623799813));
#48998=CARTESIAN_POINT('Ctrl Pts',(0.118526476885983,-0.0275700362329285,
-0.274626080647599));
#48999=CARTESIAN_POINT('Ctrl Pts',(0.127551748668178,0.011230553590179,
-0.272267537495385));
#49000=CARTESIAN_POINT('Ctrl Pts',(0.115682855895611,0.0548912631853853,
-0.269908994343171));
#49001=CARTESIAN_POINT('Ctrl Pts',(0.0882559653534158,0.0837825590467683,
-0.267550451190957));
#49002=CARTESIAN_POINT('Ctrl Pts',(0.0608290748112208,0.112673854908151,
-0.265191908038743));
#49003=CARTESIAN_POINT('Ctrl Pts',(0.017844186499398,0.126795737035712,
-0.262833364886529));
#49004=CARTESIAN_POINT('Ctrl Pts',(-0.0213730103482152,0.11979911122185,
-0.260474821734315));
#49005=CARTESIAN_POINT('Ctrl Pts',(-0.0605902071958284,0.112802485407989,
-0.258116278582101));
#49006=CARTESIAN_POINT('Ctrl Pts',(-0.0960397125792319,0.0846873516527053,
-0.255757735429887));
#49007=CARTESIAN_POINT('Ctrl Pts',(-0.111783689936811,0.0480940670457318,
-0.253399192277673));
#49008=CARTESIAN_POINT('Ctrl Pts',(-0.118258566725731,0.0330446926881158,
-0.252429216523447));
#49009=CARTESIAN_POINT('Ctrl Pts',(-0.121400544301244,0.0165613642508264,
-0.251459240769221));
#49010=CARTESIAN_POINT('Ctrl Pts',(-0.121333512465724,5.36033326936202E-5,
-0.250489265014994));
#49011=CARTESIAN_POINT('Origin',(0.,0.,-0.29));
#49012=CARTESIAN_POINT('',(-0.121516972739373,-0.000104509287172358,-0.199010734985006));
#49013=CARTESIAN_POINT('',(-0.121504492117652,-0.000105281444988491,-0.205489265014994));
#49014=CARTESIAN_POINT('',(-0.1215,-1.48794586096403E-17,-0.29));
#49015=CARTESIAN_POINT('Ctrl Pts',(-0.121516972739373,-0.000104509287172358,
-0.199010734985006));
#49016=CARTESIAN_POINT('Ctrl Pts',(-0.121237398482098,0.0311537138205197,
-0.200854488433116));
#49017=CARTESIAN_POINT('Ctrl Pts',(-0.108897454112275,0.0626080735884432,
-0.202698241881227));
#49018=CARTESIAN_POINT('Ctrl Pts',(-0.0871671833886449,0.0849147559896284,
-0.204541995329337));
#49019=CARTESIAN_POINT('Ctrl Pts',(-0.0593696591244869,0.113449630367679,
-0.206900538481551));
#49020=CARTESIAN_POINT('Ctrl Pts',(-0.0162060704891954,0.127015504311929,
-0.209259081633765));
#49021=CARTESIAN_POINT('Ctrl Pts',(0.0229175509337778,0.119513260790107,
-0.211617624785979));
#49022=CARTESIAN_POINT('Ctrl Pts',(0.0620411723567516,0.112011017268286,
-0.213976167938193));
#49023=CARTESIAN_POINT('Ctrl Pts',(0.0971248265674069,0.083440656280392,
-0.216334711090408));
#49024=CARTESIAN_POINT('Ctrl Pts',(0.112395160997276,0.0466472017324166,
-0.218693254242622));
#49025=CARTESIAN_POINT('Ctrl Pts',(0.127665495427144,0.00985374718444192,
-0.221051797394836));
#49026=CARTESIAN_POINT('Ctrl Pts',(0.123122510076227,-0.0351628009236139,
-0.22341034054705));
#49027=CARTESIAN_POINT('Ctrl Pts',(0.100808697702601,-0.0681633340777489,
-0.225768883699264));
#49028=CARTESIAN_POINT('Ctrl Pts',(0.078494885328975,-0.101163867231884,
-0.228127426851478));
#49029=CARTESIAN_POINT('Ctrl Pts',(0.0384102459326391,-0.122148385432099,
-0.230485970003692));
#49030=CARTESIAN_POINT('Ctrl Pts',(-0.00142346180680877,-0.121682403829303,
-0.232844513155906));
#49031=CARTESIAN_POINT('Ctrl Pts',(-0.0412571695462569,-0.121216422226508,
-0.23520305630812));
#49032=CARTESIAN_POINT('Ctrl Pts',(-0.080839945628817,-0.099299940820702,
-0.237561599460334));
#49033=CARTESIAN_POINT('Ctrl Pts',(-0.10237566542496,-0.0657864482543611,
-0.239920142612548));
#49034=CARTESIAN_POINT('Ctrl Pts',(-0.114825985452785,-0.046411488343535,
-0.241283673403367));
#49035=CARTESIAN_POINT('Ctrl Pts',(-0.121244482067543,-0.0231604878015092,
-0.242647204194187));
#49036=CARTESIAN_POINT('Ctrl Pts',(-0.121328086182402,4.76889891967633E-5,
-0.244010734985006));
#49037=CARTESIAN_POINT('Ctrl Pts',(-0.121333512465724,5.36033326936202E-5,
-0.250489265014994));
#49038=CARTESIAN_POINT('Ctrl Pts',(-0.121237553137851,-0.0235780581029944,
-0.249100697617007));
#49039=CARTESIAN_POINT('Ctrl Pts',(-0.114565270411393,-0.0472597897861873,
-0.247712130219019));
#49040=CARTESIAN_POINT('Ctrl Pts',(-0.101680121938708,-0.0668564538650969,
-0.246323562821031));
#49041=CARTESIAN_POINT('Ctrl Pts',(-0.0797941272512696,-0.100142254710288,
-0.243965019668817));
#49042=CARTESIAN_POINT('Ctrl Pts',(-0.0399836885446386,-0.121642420942007,
-0.241606476516603));
#49043=CARTESIAN_POINT('Ctrl Pts',(-0.000147285887556907,-0.121690636154816,
-0.239247933364389));
#49044=CARTESIAN_POINT('Ctrl Pts',(0.0396891167695248,-0.121738851367624,
-0.236889390212175));
#49045=CARTESIAN_POINT('Ctrl Pts',(0.0795514833770574,-0.100335115561522,
-0.234530847059961));
#49046=CARTESIAN_POINT('Ctrl Pts',(0.101517987464407,-0.06710239073282,
-0.232172303907747));
#49047=CARTESIAN_POINT('Ctrl Pts',(0.123484491551756,-0.033869665904118,
-0.229813760755532));
#49048=CARTESIAN_POINT('Ctrl Pts',(0.127555133118923,0.0111920479471833,
-0.227455217603318));
#49049=CARTESIAN_POINT('Ctrl Pts',(0.111899781694571,0.0478233361193179,
-0.225096674451104));
#49050=CARTESIAN_POINT('Ctrl Pts',(0.0962444302702202,0.0844546242914523,
-0.22273813129889));
#49051=CARTESIAN_POINT('Ctrl Pts',(0.0608630858543512,0.11265548678442,
-0.220379588146676));
#49052=CARTESIAN_POINT('Ctrl Pts',(0.021662940339392,0.119747023498675,
-0.218021044994462));
#49053=CARTESIAN_POINT('Ctrl Pts',(-0.0175372051755671,0.12683856021293,
-0.215662501842248));
#49054=CARTESIAN_POINT('Ctrl Pts',(-0.0605561517896168,0.112820771148474,
-0.213303958690034));
#49055=CARTESIAN_POINT('Ctrl Pts',(-0.0880528979067979,0.0839959510396251,
-0.21094541553782));
#49056=CARTESIAN_POINT('Ctrl Pts',(-0.109256154326964,0.0617685918667089,
-0.209126698696878));
#49057=CARTESIAN_POINT('Ctrl Pts',(-0.121229535898851,0.0307366148535648,
-0.207307981855936));
#49058=CARTESIAN_POINT('Ctrl Pts',(-0.121504492117652,-0.000105281444988491,
-0.205489265014994));
#49059=CARTESIAN_POINT('Origin',(0.,0.,-0.29));
#49060=CARTESIAN_POINT('',(-0.121603817730479,8.52412621186009E-5,-0.154010734985006));
#49061=CARTESIAN_POINT('',(-0.12161467894854,8.07629804098239E-5,-0.160489265014994));
#49062=CARTESIAN_POINT('',(-0.1215,-1.48794586096403E-17,-0.29));
#49063=CARTESIAN_POINT('Ctrl Pts',(-0.121603817730479,8.52412621186009E-5,
-0.154010734985006));
#49064=CARTESIAN_POINT('Ctrl Pts',(-0.121649091313963,0.00573644262637322,
-0.154344686367618));
#49065=CARTESIAN_POINT('Ctrl Pts',(-0.121288511086501,0.0113818407630408,
-0.15467863775023));
#49066=CARTESIAN_POINT('Ctrl Pts',(-0.120502055093573,0.0169672735145346,
-0.155012589132842));
#49067=CARTESIAN_POINT('Ctrl Pts',(-0.114947682531521,0.0564145848720949,
-0.157371132285057));
#49068=CARTESIAN_POINT('Ctrl Pts',(-0.0881508852131287,0.0928708592047098,
-0.159729675437271));
#49069=CARTESIAN_POINT('Ctrl Pts',(-0.0521593058589881,0.109945624876804,
-0.162088218589485));
#49070=CARTESIAN_POINT('Ctrl Pts',(-0.0161677265048477,0.127020390548898,
-0.164446761741699));
#49071=CARTESIAN_POINT('Ctrl Pts',(0.0290186348850403,0.124713647560471,
-0.166805304893913));
#49072=CARTESIAN_POINT('Ctrl Pts',(0.0630843229848925,0.104062490133902,
-0.169163848046127));
#49073=CARTESIAN_POINT('Ctrl Pts',(0.0971500110847444,0.0834113327073327,
-0.171522391198341));
#49074=CARTESIAN_POINT('Ctrl Pts',(0.12009502589456,0.0444157608426204,
-0.173880934350555));
#49075=CARTESIAN_POINT('Ctrl Pts',(0.121603457732842,0.00460789670778811,
-0.176239477502769));
#49076=CARTESIAN_POINT('Ctrl Pts',(0.123111889571124,-0.0351999674270442,
-0.178598020654983));
#49077=CARTESIAN_POINT('Ctrl Pts',(0.103183738437872,-0.0758201238319969,
-0.180956563807197));
#49078=CARTESIAN_POINT('Ctrl Pts',(0.0707785543245695,-0.0989900494454684,
-0.183315106959411));
#49079=CARTESIAN_POINT('Ctrl Pts',(0.0383733702112669,-0.12215997505894,
-0.185673650111625));
#49080=CARTESIAN_POINT('Ctrl Pts',(-0.00650884688208582,-0.12787966988093,
-0.188032193263839));
#49081=CARTESIAN_POINT('Ctrl Pts',(-0.0436893826726646,-0.113577601176793,
-0.190390736416053));
#49082=CARTESIAN_POINT('Ctrl Pts',(-0.0808699184632431,-0.0992755324726549,
-0.192749279568267));
#49083=CARTESIAN_POINT('Ctrl Pts',(-0.110348772951047,-0.0649517002423889,
-0.195107822720481));
#49084=CARTESIAN_POINT('Ctrl Pts',(-0.118872470248437,-0.0260378467213308,
-0.197466365872695));
#49085=CARTESIAN_POINT('Ctrl Pts',(-0.120732903289687,-0.0175442768153356,
-0.197981155576799));
#49086=CARTESIAN_POINT('Ctrl Pts',(-0.121595031955655,-0.00883203814462564,
-0.198495945280902));
#49087=CARTESIAN_POINT('Ctrl Pts',(-0.121516972739373,-0.000104509287172358,
-0.199010734985006));
#49088=CARTESIAN_POINT('Ctrl Pts',(-0.121504492117652,-0.000105281444988491,
-0.205489265014994));
#49089=CARTESIAN_POINT('Ctrl Pts',(-0.12158610383313,-0.00925968455859438,
-0.204949438703722));
#49090=CARTESIAN_POINT('Ctrl Pts',(-0.120637079500945,-0.0183973414836741,
-0.20440961239245));
#49091=CARTESIAN_POINT('Ctrl Pts',(-0.118592867240787,-0.0272830434597006,
-0.203869786081178));
#49092=CARTESIAN_POINT('Ctrl Pts',(-0.109661544837283,-0.0661053666969373,
-0.201511242928964));
#49093=CARTESIAN_POINT('Ctrl Pts',(-0.0798243544099606,-0.10011816201817,
-0.19915269977675));
#49094=CARTESIAN_POINT('Ctrl Pts',(-0.0424958770457137,-0.114029527120612,
-0.196794156624536));
#49095=CARTESIAN_POINT('Ctrl Pts',(-0.00516739968146744,-0.127940892223055,
-0.194435613472322));
#49096=CARTESIAN_POINT('Ctrl Pts',(0.0396523646197032,-0.121750827106708,
-0.192077070320108));
#49097=CARTESIAN_POINT('Ctrl Pts',(0.071812779889887,-0.0982423394719399,
-0.189718527167894));
#49098=CARTESIAN_POINT('Ctrl Pts',(0.103973195160071,-0.0747338518371711,
-0.18735998401568));
#49099=CARTESIAN_POINT('Ctrl Pts',(0.123474261399268,-0.0339069416839796,
-0.185001440863466));
#49100=CARTESIAN_POINT('Ctrl Pts',(0.121548442840219,0.00588291285951405,
-0.182642897711252));
#49101=CARTESIAN_POINT('Ctrl Pts',(0.11962262428117,0.0456727674030071,
-0.180284354559038));
#49102=CARTESIAN_POINT('Ctrl Pts',(0.0962699209238745,0.0844255663368025,
-0.177925811406823));
#49103=CARTESIAN_POINT('Ctrl Pts',(0.0619895362165354,0.10471833661211,
-0.175567268254609));
#49104=CARTESIAN_POINT('Ctrl Pts',(0.027709151509196,0.125011106887417,
-0.173208725102395));
#49105=CARTESIAN_POINT('Ctrl Pts',(-0.0174989145481876,0.126843848504235,
-0.170850181950181));
#49106=CARTESIAN_POINT('Ctrl Pts',(-0.0533094483675094,0.109392574391408,
-0.168491638797967));
#49107=CARTESIAN_POINT('Ctrl Pts',(-0.0891199821868312,0.0919413002785813,
-0.166133095645753));
#49108=CARTESIAN_POINT('Ctrl Pts',(-0.115532983768091,0.0552060104361086,
-0.163774552493539));
#49109=CARTESIAN_POINT('Ctrl Pts',(-0.120673362134684,0.015702620529911,
-0.161416009341325));
#49110=CARTESIAN_POINT('Ctrl Pts',(-0.121346633186486,0.0105285872243599,
-0.161107094565881));
#49111=CARTESIAN_POINT('Ctrl Pts',(-0.121654973238394,0.00530706727299804,
-0.160798179790438));
#49112=CARTESIAN_POINT('Ctrl Pts',(-0.12161467894854,8.07629804098239E-5,
-0.160489265014994));
#49113=CARTESIAN_POINT('Origin',(0.,0.,-0.29));
#49114=CARTESIAN_POINT('',(-0.121309037101631,-9.33618319136557E-7,-0.109010734985006));
#49115=CARTESIAN_POINT('',(-0.121309301434334,5.79271293234657E-6,-0.115489265014994));
#49116=CARTESIAN_POINT('',(-0.1215,-1.48794586096403E-17,-0.29));
#49117=CARTESIAN_POINT('Ctrl Pts',(-0.121309046518887,-9.33572278136174E-7,
-0.109010734985006));
#49118=CARTESIAN_POINT('Ctrl Pts',(-0.121307664074448,0.0201371841581811,
-0.110193427454334));
#49119=CARTESIAN_POINT('Ctrl Pts',(-0.116556959955105,0.0402759190252943,
-0.111376119923662));
#49120=CARTESIAN_POINT('Ctrl Pts',(-0.107060609773819,0.0578503306347235,
-0.11255881239299));
#49121=CARTESIAN_POINT('Ctrl Pts',(-0.0881228450784662,0.0928974872122608,
-0.114917355545204));
#49122=CARTESIAN_POINT('Ctrl Pts',(-0.0503121501341162,0.11774660260711,
-0.117275898697418));
#49123=CARTESIAN_POINT('Ctrl Pts',(-0.0106279342068158,0.121225736562482,
-0.119634441849632));
#49124=CARTESIAN_POINT('Ctrl Pts',(0.0290562817204846,0.124704870517854,
-0.121992985001846));
#49125=CARTESIAN_POINT('Ctrl Pts',(0.0706140186307353,0.106814023033748,
-0.12435152815406));
#49126=CARTESIAN_POINT('Ctrl Pts',(0.0953612236640026,0.0755967668366386,
-0.126710071306274));
#49127=CARTESIAN_POINT('Ctrl Pts',(0.12010842869727,0.0443795106395292,
-0.129068614458488));
#49128=CARTESIAN_POINT('Ctrl Pts',(0.128045101853553,-0.000164154270584499,
-0.131427157610702));
#49129=CARTESIAN_POINT('Ctrl Pts',(0.115602973532799,-0.0380077133606588,
-0.133785700762916));
#49130=CARTESIAN_POINT('Ctrl Pts',(0.103160845212044,-0.0758512724507334,
-0.13614424391513));
#49131=CARTESIAN_POINT('Ctrl Pts',(0.0703399154142509,-0.106994725720769,
-0.138502787067344));
#49132=CARTESIAN_POINT('Ctrl Pts',(0.0318962323681036,-0.117436211625325,
-0.140861330219558));
#49133=CARTESIAN_POINT('Ctrl Pts',(-0.00654745067804376,-0.127877697529882,
-0.143219873371772));
#49134=CARTESIAN_POINT('Ctrl Pts',(-0.0506138869725449,-0.117617216068959,
-0.145578416523986));
#49135=CARTESIAN_POINT('Ctrl Pts',(-0.08049113121694,-0.0912678011472448,
-0.1479369596762));
#49136=CARTESIAN_POINT('Ctrl Pts',(-0.106137989846092,-0.0686492586226994,
-0.149961551445802));
#49137=CARTESIAN_POINT('Ctrl Pts',(-0.121329345069859,-0.0341753618260928,
-0.151986143215404));
#49138=CARTESIAN_POINT('Ctrl Pts',(-0.121603817730479,8.52412621186009E-5,
-0.154010734985006));
#49139=CARTESIAN_POINT('Ctrl Pts',(-0.12161467894854,8.07629804098239E-5,
-0.160489265014994));
#49140=CARTESIAN_POINT('Ctrl Pts',(-0.121347329095214,-0.0345954080390664,
-0.158439636638224));
#49141=CARTESIAN_POINT('Ctrl Pts',(-0.105732288041653,-0.0694821968403921,
-0.156390008261453));
#49142=CARTESIAN_POINT('Ctrl Pts',(-0.0795295660295233,-0.0921068985596655,
-0.154340379884683));
#49143=CARTESIAN_POINT('Ctrl Pts',(-0.0493776364058448,-0.11814153777312,
-0.151981836732469));
#49144=CARTESIAN_POINT('Ctrl Pts',(-0.00520602200656287,-0.127939326230107,
-0.149623293580255));
#49145=CARTESIAN_POINT('Ctrl Pts',(0.0331260445435072,-0.117095250825184,
-0.147264750428041));
#49146=CARTESIAN_POINT('Ctrl Pts',(0.0714581110935774,-0.106251175420261,
-0.144906207275827));
#49147=CARTESIAN_POINT('Ctrl Pts',(0.103950629794436,-0.0747652361534276,
-0.142547664123613));
#49148=CARTESIAN_POINT('Ctrl Pts',(0.115995203675548,-0.0367932786294693,
-0.140189120971399));
#49149=CARTESIAN_POINT('Ctrl Pts',(0.12803977755666,0.00117867889448893,
-0.137830577819185));
#49150=CARTESIAN_POINT('Ctrl Pts',(0.119636406618026,0.0456366546755723,
-0.135472034666971));
#49151=CARTESIAN_POINT('Ctrl Pts',(0.0945631842556541,0.0765926686457221,
-0.133113491514757));
#49152=CARTESIAN_POINT('Ctrl Pts',(0.0694899618932821,0.107548682615872,
-0.130754948362543));
#49153=CARTESIAN_POINT('Ctrl Pts',(0.0277468881071721,0.125002734775089,
-0.128396405210329));
#49154=CARTESIAN_POINT('Ctrl Pts',(-0.0118986579771398,0.121107614763766,
-0.126037862058114));
#49155=CARTESIAN_POINT('Ctrl Pts',(-0.0515442040614505,0.117212494752444,
-0.1236793189059));
#49156=CARTESIAN_POINT('Ctrl Pts',(-0.0890922224439633,0.091968202570584,
-0.121320775753686));
#49157=CARTESIAN_POINT('Ctrl Pts',(-0.107661401631213,0.056724380465849,
-0.118962232601472));
#49158=CARTESIAN_POINT('Ctrl Pts',(-0.116775807327555,0.03942547405146,
-0.117804576739313));
#49159=CARTESIAN_POINT('Ctrl Pts',(-0.121317847477761,0.0197174895250484,
-0.116646920877154));
#49160=CARTESIAN_POINT('Ctrl Pts',(-0.121309301434334,5.79271293234657E-6,
-0.115489265014994));
#49161=CARTESIAN_POINT('Origin',(0.,0.,-0.29));
#49162=CARTESIAN_POINT('',(-0.121606852599128,-8.52915087747597E-5,-0.0640107349850058));
#49163=CARTESIAN_POINT('',(-0.121595695105322,-8.84116883933851E-5,-0.0704892650149944));
#49164=CARTESIAN_POINT('',(-0.1215,-1.48794586096403E-17,-0.29));
#49165=CARTESIAN_POINT('Ctrl Pts',(-0.121606852599128,-8.52915087747597E-5,
-0.0640107349850058));
#49166=CARTESIAN_POINT('Ctrl Pts',(-0.121334152356696,0.0342887112479717,
-0.0660421685410495));
#49167=CARTESIAN_POINT('Ctrl Pts',(-0.106027699321683,0.0688771005653459,
-0.0680736020970932));
#49168=CARTESIAN_POINT('Ctrl Pts',(-0.0802292283098266,0.0914986392585654,
-0.0701050356531369));
#49169=CARTESIAN_POINT('Ctrl Pts',(-0.0502765838033985,0.11776278903531,
-0.072463578805351));
#49170=CARTESIAN_POINT('Ctrl Pts',(-0.00618094275775686,0.127895902119566,
-0.074822121957565));
#49171=CARTESIAN_POINT('Ctrl Pts',(0.0322326537889043,0.117344037501139,
-0.077180665109779));
#49172=CARTESIAN_POINT('Ctrl Pts',(0.0706462503355655,0.106792172882712,
-0.079539208261993));
#49173=CARTESIAN_POINT('Ctrl Pts',(0.103377802383246,0.0755553305616026,
-0.081897751414207));
#49174=CARTESIAN_POINT('Ctrl Pts',(0.115711427039349,0.0376764002307086,
-0.0842562945664211));
#49175=CARTESIAN_POINT('Ctrl Pts',(0.128045051695452,-0.000202530100185408,
-0.0866148377186352));
#49176=CARTESIAN_POINT('Ctrl Pts',(0.119980748959977,-0.0447235484408638,
-0.0889733808708493));
#49177=CARTESIAN_POINT('Ctrl Pts',(0.0951441795036263,-0.0758698249428511,
-0.0913319240230634));
#49178=CARTESIAN_POINT('Ctrl Pts',(0.0703076100472756,-0.107016101444838,
-0.0936904671752774));
#49179=CARTESIAN_POINT('Ctrl Pts',(0.028698773870049,-0.124787636108134,
-0.0960490103274914));
#49180=CARTESIAN_POINT('Ctrl Pts',(-0.0109753077276821,-0.121194745221755,
-0.0984075534797054));
#49181=CARTESIAN_POINT('Ctrl Pts',(-0.050649389325413,-0.117601854335375,
-0.100766096631919));
#49182=CARTESIAN_POINT('Ctrl Pts',(-0.0883887163436492,-0.0926445378993189,
-0.103124639784134));
#49183=CARTESIAN_POINT('Ctrl Pts',(-0.107225962629589,-0.0575432808011788,
-0.105483182936348));
#49184=CARTESIAN_POINT('Ctrl Pts',(-0.116617263733503,-0.0400435640415918,
-0.106659033619234));
#49185=CARTESIAN_POINT('Ctrl Pts',(-0.121310420965989,-0.0200225538154995,
-0.10783488430212));
#49186=CARTESIAN_POINT('Ctrl Pts',(-0.121309046518887,-9.33572278136174E-7,
-0.109010734985006));
#49187=CARTESIAN_POINT('Ctrl Pts',(-0.121309301434334,5.79271293234657E-6,
-0.115489265014994));
#49188=CARTESIAN_POINT('Ctrl Pts',(-0.121300436247998,-0.0204420164683971,
-0.11428837772494));
#49189=CARTESIAN_POINT('Ctrl Pts',(-0.116394765147926,-0.0408938203752012,
-0.113087490434885));
#49190=CARTESIAN_POINT('Ctrl Pts',(-0.106616599719654,-0.0586645870706639,
-0.11188660314483));
#49191=CARTESIAN_POINT('Ctrl Pts',(-0.087412278628859,-0.0935663804748282,
-0.109528059992616));
#49192=CARTESIAN_POINT('Ctrl Pts',(-0.0494132964552827,-0.118126615255547,
-0.107169516840402));
#49193=CARTESIAN_POINT('Ctrl Pts',(-0.00970371956802299,-0.121303210962312,
-0.104810973688188));
#49194=CARTESIAN_POINT('Ctrl Pts',(0.0300058573192376,-0.124479806669077,
-0.102452430535974));
#49195=CARTESIAN_POINT('Ctrl Pts',(0.0714260289201816,-0.106272763301887,
-0.10009388738376));
#49196=CARTESIAN_POINT('Ctrl Pts',(0.0959345983609506,-0.0748677950423748,
-0.097735344231546));
#49197=CARTESIAN_POINT('Ctrl Pts',(0.120443167801719,-0.0434628267828625,
-0.095376801079332));
#49198=CARTESIAN_POINT('Ctrl Pts',(0.128040135082313,0.00114006636897254,
-0.0930182579271179));
#49199=CARTESIAN_POINT('Ctrl Pts',(0.11530994589185,0.0388876791290693,
-0.0906597147749039));
#49200=CARTESIAN_POINT('Ctrl Pts',(0.102579756701387,0.0766352918891664,
-0.0883011716226898));
#49201=CARTESIAN_POINT('Ctrl Pts',(0.0695224110398688,0.107527624257525,
-0.0859426284704758));
#49202=CARTESIAN_POINT('Ctrl Pts',(0.0310002742191683,0.117675849709285,
-0.0835840853182618));
#49203=CARTESIAN_POINT('Ctrl Pts',(-0.00752186260153201,0.127824075161045,
-0.0812255421660478));
#49204=CARTESIAN_POINT('Ctrl Pts',(-0.0515087905814142,0.117228193696207,
-0.0788669990138337));
#49205=CARTESIAN_POINT('Ctrl Pts',(-0.0811843604808662,0.0906517723674608,
-0.0765084558616196));
#49206=CARTESIAN_POINT('Ctrl Pts',(-0.106429170119603,0.0680433877737934,
-0.0745020589127445));
#49207=CARTESIAN_POINT('Ctrl Pts',(-0.121317148211621,0.033870219567978,
-0.0724956619638695));
#49208=CARTESIAN_POINT('Ctrl Pts',(-0.121595695105322,-8.84116883933851E-5,
-0.0704892650149944));
#49209=CARTESIAN_POINT('Origin',(0.,0.,-0.29));
#49210=CARTESIAN_POINT('',(-0.121508540285962,0.000130861710946541,-0.0190107349850059));
#49211=CARTESIAN_POINT('',(-0.121526217441981,0.000102663445846418,-0.0254892650149941));
#49212=CARTESIAN_POINT('',(-0.1215,-1.48794586096403E-17,-0.29));
#49213=CARTESIAN_POINT('Ctrl Pts',(-0.121508540285962,0.000130861710946541,
-0.0190107349850059));
#49214=CARTESIAN_POINT('Ctrl Pts',(-0.121590276950577,0.0089502089992317,
-0.0195323664755513));
#49215=CARTESIAN_POINT('Ctrl Pts',(-0.120706038295682,0.0177562809340787,
-0.0200539979660966));
#49216=CARTESIAN_POINT('Ctrl Pts',(-0.118797094411048,0.0263429264125233,
-0.020575629456642));
#49217=CARTESIAN_POINT('Ctrl Pts',(-0.110165854524904,0.0651672195404196,
-0.0229341726088561));
#49218=CARTESIAN_POINT('Ctrl Pts',(-0.080585821771702,0.0995056183337115,
-0.0252927157610701));
#49219=CARTESIAN_POINT('Ctrl Pts',(-0.0433635147056392,0.113725897500623,
-0.0276512589132841));
#49220=CARTESIAN_POINT('Ctrl Pts',(-0.00614120763957639,0.127946176667534,
-0.0300098020654982));
#49221=CARTESIAN_POINT('Ctrl Pts',(0.0387233737393477,0.122048336208064,
-0.0323683452177122));
#49222=CARTESIAN_POINT('Ctrl Pts',(0.0710617426615871,0.0987737492725815,
-0.0347268883699262));
#49223=CARTESIAN_POINT('Ctrl Pts',(0.103400111583827,0.0754991623370986,
-0.0370854315221403));
#49224=CARTESIAN_POINT('Ctrl Pts',(0.123212268049381,0.0348478289256035,
-0.0394439746743542));
#49225=CARTESIAN_POINT('Ctrl Pts',(0.121589879662122,-0.00494942974450984,
-0.0418025178265683));
#49226=CARTESIAN_POINT('Ctrl Pts',(0.119967491274862,-0.0447466884146232,
-0.0441610609787823));
#49227=CARTESIAN_POINT('Ctrl Pts',(0.0969105580347855,-0.0836898723433555,
-0.0465196041309965));
#49228=CARTESIAN_POINT('Ctrl Pts',(0.0627857651119705,-0.104246522245439,
-0.0488781472832105));
#49229=CARTESIAN_POINT('Ctrl Pts',(0.0286609721891549,-0.124803172147523,
-0.0512366904354246));
#49230=CARTESIAN_POINT('Ctrl Pts',(-0.0165316804163984,-0.126973288022959,
-0.0535952335876386));
#49231=CARTESIAN_POINT('Ctrl Pts',(-0.0524741460072976,-0.109793759220386,
-0.0559537767398526));
#49232=CARTESIAN_POINT('Ctrl Pts',(-0.0884166115981963,-0.0926142304178135,
-0.0583123198920666));
#49233=CARTESIAN_POINT('Ctrl Pts',(-0.11510889017444,-0.0560850569372318,
-0.0606708630442807));
#49234=CARTESIAN_POINT('Ctrl Pts',(-0.120550205478954,-0.0166228769623238,
-0.0630294061964947));
#49235=CARTESIAN_POINT('Ctrl Pts',(-0.121304868988174,-0.0111498129043366,
-0.0633565157926651));
#49236=CARTESIAN_POINT('Ctrl Pts',(-0.121650763888233,-0.00562033159269298,
-0.0636836253888354));
#49237=CARTESIAN_POINT('Ctrl Pts',(-0.121606852599128,-8.52915087747597E-5,
-0.0640107349850058));
#49238=CARTESIAN_POINT('Ctrl Pts',(-0.121595695105322,-8.84116883933851E-5,
-0.0704892650149944));
#49239=CARTESIAN_POINT('Ctrl Pts',(-0.121644583353046,-0.00604854987252561,
-0.0701371188116555));
#49240=CARTESIAN_POINT('Ctrl Pts',(-0.121243437305456,-0.0120020793815115,
-0.0697849726083166));
#49241=CARTESIAN_POINT('Ctrl Pts',(-0.12036926516354,-0.0178853149891245,
-0.0694328264049777));
#49242=CARTESIAN_POINT('Ctrl Pts',(-0.11451438812774,-0.0572890198243118,
-0.0670742832527636));
#49243=CARTESIAN_POINT('Ctrl Pts',(-0.087440422237116,-0.0935394683020307,
-0.0647157401005495));
#49244=CARTESIAN_POINT('Ctrl Pts',(-0.0513198022297531,-0.110339675010818,
-0.0623571969483354));
#49245=CARTESIAN_POINT('Ctrl Pts',(-0.0151991822223908,-0.127139881719604,
-0.0599986537961213));
#49246=CARTESIAN_POINT('Ctrl Pts',(0.0299680919017115,-0.124489846659459,
-0.0576401106439072));
#49247=CARTESIAN_POINT('Ctrl Pts',(0.0638754863487052,-0.103579203383963,
-0.0552815674916932));
#49248=CARTESIAN_POINT('Ctrl Pts',(0.0977828807956984,-0.0826685601084671,
-0.0529230243394792));
#49249=CARTESIAN_POINT('Ctrl Pts',(0.120430395565585,-0.0434973086176221,
-0.0505644811872652));
#49250=CARTESIAN_POINT('Ctrl Pts',(0.121635229050253,-0.00367997854823185,
-0.0482059380350512));
#49251=CARTESIAN_POINT('Ctrl Pts',(0.122840062534921,0.0361373515211595,
-0.0458473948828371));
#49252=CARTESIAN_POINT('Ctrl Pts',(0.10260221473437,0.0766007601690952,
-0.043488851730623));
#49253=CARTESIAN_POINT('Ctrl Pts',(0.0700216994762484,0.0995246985894165,
-0.041130308578409));
#49254=CARTESIAN_POINT('Ctrl Pts',(0.0374411842181272,0.122448637009737,
-0.0387717654261949));
#49255=CARTESIAN_POINT('Ctrl Pts',(-0.00748199849756367,0.127833105202444,
-0.0364132222739809));
#49256=CARTESIAN_POINT('Ctrl Pts',(-0.0445530473550404,0.11324493435664,
-0.0340546791217669));
#49257=CARTESIAN_POINT('Ctrl Pts',(-0.0816240962125166,0.098656763510837,
-0.0316961359695529));
#49258=CARTESIAN_POINT('Ctrl Pts',(-0.110843011211779,0.0640959536265228,
-0.0293375928173388));
#49259=CARTESIAN_POINT('Ctrl Pts',(-0.119068742960021,0.0251242850883948,
-0.0269790496651247));
#49260=CARTESIAN_POINT('Ctrl Pts',(-0.120800683414184,0.0169187404179371,
-0.0264824547817479));
#49261=CARTESIAN_POINT('Ctrl Pts',(-0.121601955132731,0.00851765378525109,
-0.025985859898371));
#49262=CARTESIAN_POINT('Ctrl Pts',(-0.121526217441981,0.000102663445846418,
-0.0254892650149941));
#49263=CARTESIAN_POINT('Origin',(0.,0.,-0.656687266823562));
#49264=CARTESIAN_POINT('',(-0.0959092728420695,-6.72679739015819E-5,-0.0491872668235618));
#49265=CARTESIAN_POINT('',(-0.0958456772541386,8.09689275490001E-5,-0.0403127331764372));
#49266=CARTESIAN_POINT('',(-0.095825,-8.02710626669594E-15,-0.656687266823562));
#49267=CARTESIAN_POINT('',(-0.0256835729485001,0.0924624001170202,-0.0134999999999999));
#49268=CARTESIAN_POINT('Ctrl Pts',(-0.0959092728420695,-6.72679739015716E-5,
-0.0491872668235618));
#49269=CARTESIAN_POINT('Ctrl Pts',(-0.0959439049348964,-0.00443266069852132,
-0.0488601572273916));
#49270=CARTESIAN_POINT('Ctrl Pts',(-0.0937041356633229,-0.0402376474948893,
-0.0461745044790073));
#49271=CARTESIAN_POINT('Ctrl Pts',(-0.0486809400150489,-0.101853223691883,
-0.041130308578409));
#49272=CARTESIAN_POINT('Ctrl Pts',(0.0582471077856237,-0.0967186223643828,
-0.0340546791217668));
#49273=CARTESIAN_POINT('Ctrl Pts',(0.112800950445628,-0.0045771260688116,
-0.0269790496651248));
#49274=CARTESIAN_POINT('Ctrl Pts',(0.0674088876487516,0.0885600284958335,
-0.0201274899578691));
#49275=CARTESIAN_POINT('Ctrl Pts',(0.00179055959947813,0.0999014741116878,
-0.0156344734028275));
#49276=CARTESIAN_POINT('Ctrl Pts',(-0.0256835729485001,0.0924624001170201,
-0.0134999999999999));
#49277=CARTESIAN_POINT('',(0.0789701248920219,0.054278448757665,-0.0135));
#49278=CARTESIAN_POINT('Origin',(0.,0.,-0.0135));
#49279=CARTESIAN_POINT('Ctrl Pts',(-0.0958456772541386,8.09689275489984E-5,
-0.0403127331764372));
#49280=CARTESIAN_POINT('Ctrl Pts',(-0.0956217123444332,-0.0248031083775501,
-0.0384507849076002));
#49281=CARTESIAN_POINT('Ctrl Pts',(-0.073072965252975,-0.0815574531722432,
-0.0342302934865492));
#49282=CARTESIAN_POINT('Ctrl Pts',(0.022090743255976,-0.110784791206306,
-0.0276512589132841));
#49283=CARTESIAN_POINT('Ctrl Pts',(0.104628794236781,-0.0423248975405764,
-0.0205756294566421));
#49284=CARTESIAN_POINT('Ctrl Pts',(0.0968448185910171,0.0282724219436266,
-0.0158585431522139));
#49285=CARTESIAN_POINT('Ctrl Pts',(0.0789701248920212,0.0542784487576661,
-0.0134999999999998));
#49286=CARTESIAN_POINT('Origin',(0.,0.,-0.656687266823562));
#49287=CARTESIAN_POINT('',(-0.095674398211295,-7.36292708573769E-7,-0.094187266823562));
#49288=CARTESIAN_POINT('',(-0.0959004731149589,-6.97288069272384E-5,-0.0853127331764372));
#49289=CARTESIAN_POINT('',(-0.095825,-8.02710626669594E-15,-0.656687266823562));
#49290=CARTESIAN_POINT('Ctrl Pts',(-0.095674398211295,-7.36292708577307E-7,
-0.094187266823562));
#49291=CARTESIAN_POINT('Ctrl Pts',(-0.0956754822145337,-0.0157914503651906,
-0.093011416140676));
#49292=CARTESIAN_POINT('Ctrl Pts',(-0.0845497034522949,-0.0632540260551953,
-0.0894770223055759));
#49293=CARTESIAN_POINT('Ctrl Pts',(-0.0101819483175724,-0.112434012668085,
-0.0835840853182618));
#49294=CARTESIAN_POINT('Ctrl Pts',(0.0882666128350871,-0.0703856840480749,
-0.0765084558616196));
#49295=CARTESIAN_POINT('Ctrl Pts',(0.107347151344391,0.0349532439147777,
-0.0694328264049776));
#49296=CARTESIAN_POINT('Ctrl Pts',(0.0299026828266366,0.108861155406636,
-0.0623571969483354));
#49297=CARTESIAN_POINT('Ctrl Pts',(-0.0696064437572946,0.08599410531552,
-0.0556086770878635));
#49298=CARTESIAN_POINT('Ctrl Pts',(-0.0956941987619804,0.0270429280274596,
-0.0512187003796056));
#49299=CARTESIAN_POINT('Ctrl Pts',(-0.0959092728420695,-6.72679739015716E-5,
-0.0491872668235618));
#49300=CARTESIAN_POINT('Ctrl Pts',(-0.0959004731149589,-6.97288069272505E-5,
-0.0853127331764372));
#49301=CARTESIAN_POINT('Ctrl Pts',(-0.0959390304510746,-0.00477038923074731,
-0.0849605869730985));
#49302=CARTESIAN_POINT('Ctrl Pts',(-0.0935036780836808,-0.0409141884060264,
-0.0822498976175458));
#49303=CARTESIAN_POINT('Ctrl Pts',(-0.0476100055917889,-0.102363117493165,
-0.0771806651097791));
#49304=CARTESIAN_POINT('Ctrl Pts',(0.0592579954685063,-0.0960930036749314,
-0.0701050356531369));
#49305=CARTESIAN_POINT('Ctrl Pts',(0.112843133809849,-0.00341188826479888,
-0.0630294061964947));
#49306=CARTESIAN_POINT('Ctrl Pts',(0.064959386513852,0.0923265347892355,
-0.0559537767398527));
#49307=CARTESIAN_POINT('Ctrl Pts',(-0.04133108222025,0.105066452432841,
-0.0488781472832105));
#49308=CARTESIAN_POINT('Ctrl Pts',(-0.0922720603096074,0.0448122828611172,
-0.0436644660954054));
#49309=CARTESIAN_POINT('Ctrl Pts',(-0.0959054102929546,0.00671772982692123,
-0.0408093280598143));
#49310=CARTESIAN_POINT('Ctrl Pts',(-0.0958456772541386,8.09689275489984E-5,
-0.0403127331764372));
#49311=CARTESIAN_POINT('Origin',(0.,0.,-0.656687266823562));
#49312=CARTESIAN_POINT('',(-0.0959068792923712,6.72283452001022E-5,-0.139187266823562));
#49313=CARTESIAN_POINT('',(-0.0956745992588073,4.56861494406435E-6,-0.130312733176437));
#49314=CARTESIAN_POINT('',(-0.095825,-8.02710626669594E-15,-0.656687266823562));
#49315=CARTESIAN_POINT('Ctrl Pts',(-0.0959068792923711,6.7228345200105E-5,
-0.139187266823562));
#49316=CARTESIAN_POINT('Ctrl Pts',(-0.0956904073359593,-0.0269535312509126,
-0.13716267505396));
#49317=CARTESIAN_POINT('Ctrl Pts',(-0.0697518127439643,-0.0858162475683075,
-0.132779540132144));
#49318=CARTESIAN_POINT('Ctrl Pts',(0.0295905909193192,-0.108947251043571,
-0.126037862058114));
#49319=CARTESIAN_POINT('Ctrl Pts',(0.107246531607553,-0.0352603026583548,
-0.118962232601472));
#49320=CARTESIAN_POINT('Ctrl Pts',(0.0884679709853073,0.0701322082061288,
-0.11188660314483));
#49321=CARTESIAN_POINT('Ctrl Pts',(-0.00985968677826821,0.112462836852163,
-0.104810973688188));
#49322=CARTESIAN_POINT('Ctrl Pts',(-0.084454582307197,0.0634392161651233,
-0.0989111949144321));
#49323=CARTESIAN_POINT('Ctrl Pts',(-0.0956733079006921,0.0158818573823644,
-0.09536995929289));
#49324=CARTESIAN_POINT('Ctrl Pts',(-0.095674398211295,-7.36292708577307E-7,
-0.094187266823562));
#49325=CARTESIAN_POINT('Ctrl Pts',(-0.0956745992588073,4.56861494405394E-6,
-0.130312733176437));
#49326=CARTESIAN_POINT('Ctrl Pts',(-0.0956676074359193,-0.01612227348218,
-0.129111845886383));
#49327=CARTESIAN_POINT('Ctrl Pts',(-0.0841998304209556,-0.0639315786664402,
-0.125552415444114));
#49328=CARTESIAN_POINT('Ctrl Pts',(-0.00900227708678451,-0.112534711150002,
-0.119634441849632));
#49329=CARTESIAN_POINT('Ctrl Pts',(0.0889998943616218,-0.0694559474299769,
-0.11255881239299));
#49330=CARTESIAN_POINT('Ctrl Pts',(0.106974694106382,0.0360767003792724,
-0.105483182936348));
#49331=CARTESIAN_POINT('Ctrl Pts',(0.0287593818097131,0.109169484310085,
-0.0984075534797054));
#49332=CARTESIAN_POINT('Ctrl Pts',(-0.0701361529300369,0.0853468303619958,
-0.0916840702264021));
#49333=CARTESIAN_POINT('Ctrl Pts',(-0.0956807878796623,0.0267128707004158,
-0.0873191301253126));
#49334=CARTESIAN_POINT('Ctrl Pts',(-0.0959004731149589,-6.97288069272505E-5,
-0.0853127331764372));
#49335=CARTESIAN_POINT('Origin',(0.,0.,-0.656687266823562));
#49336=CARTESIAN_POINT('',(-0.0958383861131722,-8.24247114732218E-5,-0.184187266823562));
#49337=CARTESIAN_POINT('',(-0.0959154453518014,6.36963999718059E-5,-0.175312733176437));
#49338=CARTESIAN_POINT('',(-0.095825,-8.02710626669594E-15,-0.656687266823562));
#49339=CARTESIAN_POINT('Ctrl Pts',(-0.0958383861131722,-8.24247114732208E-5,
-0.184187266823562));
#49340=CARTESIAN_POINT('Ctrl Pts',(-0.0958999501000052,-0.00696567946674315,
-0.183672477119459));
#49341=CARTESIAN_POINT('Ctrl Pts',(-0.0921047845740635,-0.0453177134055506,
-0.180799144263141));
#49342=CARTESIAN_POINT('Ctrl Pts',(-0.040531265065401,-0.105367564795535,
-0.17556726825461));
#49343=CARTESIAN_POINT('Ctrl Pts',(0.0656622769832545,-0.0918344843926382,
-0.168491638797967));
#49344=CARTESIAN_POINT('Ctrl Pts',(0.112813266670755,0.00427481159513008,
-0.161416009341325));
#49345=CARTESIAN_POINT('Ctrl Pts',(0.0585242285435791,0.0965402603342907,
-0.154340379884683));
#49346=CARTESIAN_POINT('Ctrl Pts',(-0.0483889339301513,0.10199812815814,
-0.147264750428041));
#49347=CARTESIAN_POINT('Ctrl Pts',(-0.0936497336964331,0.0404221079648366,
-0.142213712741001));
#49348=CARTESIAN_POINT('Ctrl Pts',(-0.0959425858037904,0.00452423551170105,
-0.139521218206174));
#49349=CARTESIAN_POINT('Ctrl Pts',(-0.0959068792923711,6.7228345200105E-5,
-0.139187266823562));
#49350=CARTESIAN_POINT('Ctrl Pts',(-0.0959154453518014,6.36963999718103E-5,
-0.175312733176437));
#49351=CARTESIAN_POINT('Ctrl Pts',(-0.0957045910333214,-0.0272848146118881,
-0.173263104799667));
#49352=CARTESIAN_POINT('Ctrl Pts',(-0.0692178185861295,-0.0864609918133612,
-0.168854933270683));
#49353=CARTESIAN_POINT('Ctrl Pts',(0.0307315052759879,-0.108630938394162,
-0.162088218589485));
#49354=CARTESIAN_POINT('Ctrl Pts',(0.107610409091042,-0.0341336512276352,
-0.155012589132842));
#49355=CARTESIAN_POINT('Ctrl Pts',(0.087727618468951,0.0710561149260017,
-0.147936959676201));
#49356=CARTESIAN_POINT('Ctrl Pts',(-0.0110385554953438,0.112353264263208,
-0.140861330219558));
#49357=CARTESIAN_POINT('Ctrl Pts',(-0.0848008734968956,0.0627613659991513,
-0.134986588052971));
#49358=CARTESIAN_POINT('Ctrl Pts',(-0.0956813393790671,0.0155508513064774,
-0.131470389038597));
#49359=CARTESIAN_POINT('Ctrl Pts',(-0.0956745992588073,4.56861494405394E-6,
-0.130312733176437));
#49360=CARTESIAN_POINT('Origin',(0.,0.,-0.656687266823562));
#49361=CARTESIAN_POINT('',(-0.0956894144726637,3.76115011439749E-5,-0.229187266823562));
#49362=CARTESIAN_POINT('',(-0.0958285428573996,-8.30336993179887E-5,-0.220312733176437));
#49363=CARTESIAN_POINT('',(-0.095825,-8.02710626669594E-15,-0.656687266823562));
#49364=CARTESIAN_POINT('Ctrl Pts',(-0.0956894144726637,3.76115011439743E-5,
-0.229187266823562));
#49365=CARTESIAN_POINT('Ctrl Pts',(-0.0956234773178782,-0.0182662859553927,
-0.227823736032743));
#49366=CARTESIAN_POINT('Ctrl Pts',(-0.0818051360670546,-0.0683232197199062,
-0.22410166208971));
#49367=CARTESIAN_POINT('Ctrl Pts',(-0.00132056587373289,-0.112886506095197,
-0.218021044994462));
#49368=CARTESIAN_POINT('Ctrl Pts',(0.0935216704263627,-0.0632360997609839,
-0.21094541553782));
#49369=CARTESIAN_POINT('Ctrl Pts',(0.104270598111585,0.04327527610209,-0.203869786081178));
#49370=CARTESIAN_POINT('Ctrl Pts',(0.0212609397230408,0.110874161081468,
-0.196794156624536));
#49371=CARTESIAN_POINT('Ctrl Pts',(-0.0734359464271463,0.0811118993918514,
-0.190233316871997));
#49372=CARTESIAN_POINT('Ctrl Pts',(-0.0956178906135575,0.0245704084514466,
-0.186031020271673));
#49373=CARTESIAN_POINT('Ctrl Pts',(-0.0958383861131722,-8.24247114732208E-5,
-0.184187266823562));
#49374=CARTESIAN_POINT('Ctrl Pts',(-0.0958285428573997,-8.30336993179982E-5,
-0.220312733176437));
#49375=CARTESIAN_POINT('Ctrl Pts',(-0.0958929086404081,-0.00730295697800942,
-0.219772906865166));
#49376=CARTESIAN_POINT('Ctrl Pts',(-0.0918742640892126,-0.045996375015137,
-0.21687453740168));
#49377=CARTESIAN_POINT('Ctrl Pts',(-0.0394240328282805,-0.105786822938669,
-0.211617624785979));
#49378=CARTESIAN_POINT('Ctrl Pts',(0.0666217428299838,-0.0911408231911627,
-0.204541995329337));
#49379=CARTESIAN_POINT('Ctrl Pts',(0.112762228567538,0.00545766237499973,
-0.197466365872695));
#49380=CARTESIAN_POINT('Ctrl Pts',(0.0575085792042569,0.0971486983708248,
-0.190390736416053));
#49381=CARTESIAN_POINT('Ctrl Pts',(-0.0494559375846015,0.101485055541974,
-0.183315106959411));
#49382=CARTESIAN_POINT('Ctrl Pts',(-0.0938473597137678,0.0397453190179913,
-0.178289105879539));
#49383=CARTESIAN_POINT('Ctrl Pts',(-0.0959472247783466,0.00418559441509606,
-0.175621647951881));
#49384=CARTESIAN_POINT('Ctrl Pts',(-0.0959154453518014,6.36963999718103E-5,
-0.175312733176437));
#49385=CARTESIAN_POINT('Origin',(0.,0.,-0.656687266823562));
#49386=CARTESIAN_POINT('',(-0.0959600152474598,3.37514099930798E-5,-0.274187266823562));
#49387=CARTESIAN_POINT('',(-0.0956936940907658,4.2276044067896E-5,-0.265312733176437));
#49388=CARTESIAN_POINT('',(-0.095825,-8.02710626669594E-15,-0.656687266823562));
#49389=CARTESIAN_POINT('Ctrl Pts',(-0.0959600152474598,3.3751409993089E-5,
-0.274187266823562));
#49390=CARTESIAN_POINT('Ctrl Pts',(-0.0958240821787534,-0.0294487663342971,
-0.271974994946027));
#49391=CARTESIAN_POINT('Ctrl Pts',(-0.0656044598416009,-0.0906043475731541,
-0.267404179916278));
#49392=CARTESIAN_POINT('Ctrl Pts',(0.038055294715108,-0.106286883935013,
-0.260474821734315));
#49393=CARTESIAN_POINT('Ctrl Pts',(0.10968443433419,-0.0267288611289883,
-0.253399192277673));
#49394=CARTESIAN_POINT('Ctrl Pts',(0.0826869460855996,0.0768633599284799,
-0.246323562821031));
#49395=CARTESIAN_POINT('Ctrl Pts',(-0.0186614262296518,0.111341179819334,
-0.239247933364389));
#49396=CARTESIAN_POINT('Ctrl Pts',(-0.0869327277281451,0.0583517239853639,
-0.233535834698566));
#49397=CARTESIAN_POINT('Ctrl Pts',(-0.0957375309395074,0.0133945553659869,
-0.230182279184957));
#49398=CARTESIAN_POINT('Ctrl Pts',(-0.0956894144726637,3.76115011439743E-5,
-0.229187266823562));
#49399=CARTESIAN_POINT('Ctrl Pts',(-0.0956936940907658,4.22760440678986E-5,
-0.265312733176437));
#49400=CARTESIAN_POINT('Ctrl Pts',(-0.0956180125879371,-0.0185956166067511,
-0.26392416577845));
#49401=CARTESIAN_POINT('Ctrl Pts',(-0.0814174178878608,-0.0689973587414746,
-0.260177055228248));
#49402=CARTESIAN_POINT('Ctrl Pts',(-0.000136639224089264,-0.112894143340924,
-0.254071401525832));
#49403=CARTESIAN_POINT('Ctrl Pts',(0.0941796886812631,-0.0622518474490773,
-0.24699577206919));
#49404=CARTESIAN_POINT('Ctrl Pts',(0.103811027648513,0.0443663927929224,
-0.239920142612548));
#49405=CARTESIAN_POINT('Ctrl Pts',(0.0200970195336817,0.111091026086466,
-0.232844513155906));
#49406=CARTESIAN_POINT('Ctrl Pts',(-0.0739223767674631,0.0804546630638847,
-0.226308710010535));
#49407=CARTESIAN_POINT('Ctrl Pts',(-0.0956116895268125,0.0242414495336793,
-0.22213145001738));
#49408=CARTESIAN_POINT('Ctrl Pts',(-0.0958285428573997,-8.30336993179982E-5,
-0.220312733176437));
#49409=CARTESIAN_POINT('Origin',(0.,0.,-0.656687266823562));
#49410=CARTESIAN_POINT('',(-0.0957672392885407,-7.82302815145639E-5,-0.319187266823562));
#49411=CARTESIAN_POINT('',(-0.0959646250468222,2.82723803149889E-5,-0.310312733176438));
#49412=CARTESIAN_POINT('',(-0.095825,-8.02710626669594E-15,-0.656687266823562));
#49413=CARTESIAN_POINT('Ctrl Pts',(-0.0957672392885407,-7.82302815145602E-5,
-0.319187266823562));
#49414=CARTESIAN_POINT('Ctrl Pts',(-0.0958419044756827,-0.00948879151886152,
-0.318484797011526));
#49415=CARTESIAN_POINT('Ctrl Pts',(-0.0902748424426151,-0.05040894390654,
-0.315423784047275));
#49416=CARTESIAN_POINT('Ctrl Pts',(-0.0321311120597763,-0.108225222523459,
-0.31000422793081));
#49417=CARTESIAN_POINT('Ctrl Pts',(0.0726716307772531,-0.0863941041545113,
-0.302928598474167));
#49418=CARTESIAN_POINT('Ctrl Pts',(0.112129113562205,0.0131213202160467,
-0.295852969017526));
#49419=CARTESIAN_POINT('Ctrl Pts',(0.050761748924207,0.100838246705403,
-0.288777339560883));
#49420=CARTESIAN_POINT('Ctrl Pts',(-0.0562498327028107,0.0978829069520032,
-0.281701710104242));
#49421=CARTESIAN_POINT('Ctrl Pts',(-0.0950381444241069,0.0353555158065548,
-0.276838352525134));
#49422=CARTESIAN_POINT('Ctrl Pts',(-0.0959690028874658,0.00198308028543397,
-0.274333538098241));
#49423=CARTESIAN_POINT('Ctrl Pts',(-0.0959600152474598,3.3751409993089E-5,
-0.274187266823562));
#49424=CARTESIAN_POINT('Ctrl Pts',(-0.0959646250468222,2.82723803149913E-5,
-0.310312733176438));
#49425=CARTESIAN_POINT('Ctrl Pts',(-0.0958469111848973,-0.0297840779926777,
-0.308075424691734));
#49426=CARTESIAN_POINT('Ctrl Pts',(-0.0650257803347639,-0.0912346316416612,
-0.303479573054817));
#49427=CARTESIAN_POINT('Ctrl Pts',(0.0391678436633201,-0.105881945078975,
-0.296525178265685));
#49428=CARTESIAN_POINT('Ctrl Pts',(0.109958707539584,-0.02557711686569,
-0.289449548809043));
#49429=CARTESIAN_POINT('Ctrl Pts',(0.0818763211215267,0.07772627812099,
-0.2823739193524));
#49430=CARTESIAN_POINT('Ctrl Pts',(-0.0198280473347807,0.111139348611692,
-0.275298289895759));
#49431=CARTESIAN_POINT('Ctrl Pts',(-0.0872430988643529,0.0576722220502956,
-0.269611227837104));
#49432=CARTESIAN_POINT('Ctrl Pts',(-0.0957465609684512,0.0130616685541945,
-0.266282708930664));
#49433=CARTESIAN_POINT('Ctrl Pts',(-0.0956936940907658,4.22760440678986E-5,
-0.265312733176437));
#49434=CARTESIAN_POINT('Origin',(0.,0.,-0.656687266823562));
#49435=CARTESIAN_POINT('',(-0.0957330477189453,6.77082873043808E-5,-0.364187266823562));
#49436=CARTESIAN_POINT('',(-0.0957585699307466,-7.62084821080075E-5,-0.355312733176438));
#49437=CARTESIAN_POINT('',(-0.095825,-8.02710626669594E-15,-0.656687266823562));
#49438=CARTESIAN_POINT('Ctrl Pts',(-0.0957330477189453,6.77082873043813E-5,
-0.364187266823562));
#49439=CARTESIAN_POINT('Ctrl Pts',(-0.0955939884635277,-0.0207317147833155,
-0.36263605592481));
#49440=CARTESIAN_POINT('Ctrl Pts',(-0.0787712860380626,-0.0733605892247887,
-0.358726301873844));
#49441=CARTESIAN_POINT('Ctrl Pts',(0.00754897625919715,-0.112641555869212,
-0.352458004670662));
#49442=CARTESIAN_POINT('Ctrl Pts',(0.0981990237225277,-0.0556961299676074,
-0.345382375214021));
#49443=CARTESIAN_POINT('Ctrl Pts',(0.100549955365708,0.0513304356908642,
-0.338306745757378));
#49444=CARTESIAN_POINT('Ctrl Pts',(0.0124878480988304,0.11220142959062,
-0.331231116300736));
#49445=CARTESIAN_POINT('Ctrl Pts',(-0.0769455196192706,0.0761556323356412,
-0.324857956656131));
#49446=CARTESIAN_POINT('Ctrl Pts',(-0.0955912160292541,0.0221071779940261,
-0.320843340163739));
#49447=CARTESIAN_POINT('Ctrl Pts',(-0.0957672392885407,-7.82302815145602E-5,
-0.319187266823562));
#49448=CARTESIAN_POINT('Ctrl Pts',(-0.0957585699307466,-7.62084821080058E-5,
-0.355312733176438));
#49449=CARTESIAN_POINT('Ctrl Pts',(-0.095833385029768,-0.00982440707728614,
-0.354585226757233));
#49450=CARTESIAN_POINT('Ctrl Pts',(-0.090012622095492,-0.0510886319044539,
-0.351499177185813));
#49451=CARTESIAN_POINT('Ctrl Pts',(-0.0309943734581772,-0.108556230059475,
-0.34605458446218));
#49452=CARTESIAN_POINT('Ctrl Pts',(0.0735736570237532,-0.0856272343546855,
-0.338978955005538));
#49453=CARTESIAN_POINT('Ctrl Pts',(0.111985338737018,0.0142965093240165,
-0.331903325548895));
#49454=CARTESIAN_POINT('Ctrl Pts',(0.0497014532331962,0.101365042383611,
-0.324827696092254));
#49455=CARTESIAN_POINT('Ctrl Pts',(-0.0572732469911756,0.0972876222859135,
-0.317752066635611));
#49456=CARTESIAN_POINT('Ctrl Pts',(-0.0952073964263819,0.0346808621441382,
-0.312913745663673));
#49457=CARTESIAN_POINT('Ctrl Pts',(-0.0959710036937587,0.00164373596519372,
-0.310433967843948));
#49458=CARTESIAN_POINT('Ctrl Pts',(-0.0959646250468222,2.82723803149913E-5,
-0.310312733176438));
#49459=CARTESIAN_POINT('Origin',(0.,0.,-0.656687266823562));
#49460=CARTESIAN_POINT('',(-0.0959740869885037,-9.86262265154315E-6,-0.409187266823562));
#49461=CARTESIAN_POINT('',(-0.0957406735922206,7.06966245190496E-5,-0.400312733176438));
#49462=CARTESIAN_POINT('',(-0.095825,-8.02710626669594E-15,-0.656687266823562));
#49463=CARTESIAN_POINT('Ctrl Pts',(-0.0959740869885037,-9.86262265153463E-6,
-0.409187266823562));
#49464=CARTESIAN_POINT('Ctrl Pts',(-0.0959749085624466,-0.000561493444819199,
-0.409145857990308));
#49465=CARTESIAN_POINT('Ctrl Pts',(-0.0957226212003185,-0.0325318593928511,
-0.40674590600484));
#49466=CARTESIAN_POINT('Ctrl Pts',(-0.0604936699172284,-0.0953185347786495,
-0.401987410867158));
#49467=CARTESIAN_POINT('Ctrl Pts',(0.0462849239846546,-0.102969961087666,
-0.394911781410515));
#49468=CARTESIAN_POINT('Ctrl Pts',(0.111444796996209,-0.0180323158387254,
-0.387836151953873));
#49469=CARTESIAN_POINT('Ctrl Pts',(0.0763951494091263,0.0831197226767399,
-0.380760522497231));
#49470=CARTESIAN_POINT('Ctrl Pts',(-0.0273478910507391,0.109531730550394,
-0.373684893040589));
#49471=CARTESIAN_POINT('Ctrl Pts',(-0.0891473386466404,0.0532561389240456,
-0.368160474482699));
#49472=CARTESIAN_POINT('Ctrl Pts',(-0.0958054215155266,0.0108928289152016,
-0.364994599077024));
#49473=CARTESIAN_POINT('Ctrl Pts',(-0.0957330477189453,6.77082873043813E-5,
-0.364187266823562));
#49474=CARTESIAN_POINT('Ctrl Pts',(-0.0957406735922206,7.06966245190514E-5,
-0.400312733176438));
#49475=CARTESIAN_POINT('Ctrl Pts',(-0.0955923160348808,-0.0210601752103308,
-0.398736485670517));
#49476=CARTESIAN_POINT('Ctrl Pts',(-0.0783440141407614,-0.0740293659639809,
-0.394801695012381));
#49477=CARTESIAN_POINT('Ctrl Pts',(0.00872984600194528,-0.112556190631666,
-0.388508361202033));
#49478=CARTESIAN_POINT('Ctrl Pts',(0.0987777120733966,-0.054663240617283,
-0.38143273174539));
#49479=CARTESIAN_POINT('Ctrl Pts',(0.100006114225775,0.0523820903322742,
-0.374357102288749));
#49480=CARTESIAN_POINT('Ctrl Pts',(0.0113104914411958,0.112326217122388,
-0.367281472832106));
#49481=CARTESIAN_POINT('Ctrl Pts',(-0.0773901089245864,0.0754897857684629,
-0.360933349794669));
#49482=CARTESIAN_POINT('Ctrl Pts',(-0.0955908378373022,0.0217788151570939,
-0.356943769909447));
#49483=CARTESIAN_POINT('Ctrl Pts',(-0.0957585699307466,-7.62084821080058E-5,
-0.355312733176438));
#49484=CARTESIAN_POINT('Origin',(0.,0.,-0.656687266823562));
#49485=CARTESIAN_POINT('',(-0.0957106322133127,-5.59492053251305E-5,-0.454187266823562));
#49486=CARTESIAN_POINT('',(-0.0959720410064835,-1.57534720231084E-5,-0.445312733176438));
#49487=CARTESIAN_POINT('',(-0.095825,-8.02710626669594E-15,-0.656687266823562));
#49488=CARTESIAN_POINT('Ctrl Pts',(-0.0957106322133127,-5.59492053251263E-5,
-0.454187266823563));
#49489=CARTESIAN_POINT('Ctrl Pts',(-0.0957755559596934,-0.0119985666202428,
-0.453297116903593));
#49490=CARTESIAN_POINT('Ctrl Pts',(-0.0882017718506858,-0.0555050230914065,
-0.450048423831408));
#49491=CARTESIAN_POINT('Ctrl Pts',(-0.0235324529605039,-0.110414375714813,
-0.44444118760701));
#49492=CARTESIAN_POINT('Ctrl Pts',(0.07923206509802,-0.0804200407641335,
-0.437365558150368));
#49493=CARTESIAN_POINT('Ctrl Pts',(0.110752326466076,0.0218867699872954,
-0.430289928693726));
#49494=CARTESIAN_POINT('Ctrl Pts',(0.0426857011445824,0.104513340790562,
-0.423214299237084));
#49495=CARTESIAN_POINT('Ctrl Pts',(-0.0631402910989122,0.0932294692290819,
-0.416180078613696));
#49496=CARTESIAN_POINT('Ctrl Pts',(-0.0959281137738762,0.0308580128761358,
-0.411504401142522));
#49497=CARTESIAN_POINT('Ctrl Pts',(-0.0959740869885037,-9.86262265153463E-6,
-0.409187266823562));
#49498=CARTESIAN_POINT('Ctrl Pts',(-0.0959720410064835,-1.57534720231178E-5,
-0.445312733176438));
#49499=CARTESIAN_POINT('Ctrl Pts',(-0.0959740933575537,-0.000900961988616875,
-0.445246287736015));
#49500=CARTESIAN_POINT('Ctrl Pts',(-0.0955650009318915,-0.0332055331898721,
-0.442821299143378));
#49501=CARTESIAN_POINT('Ctrl Pts',(-0.0594907218526991,-0.0959476973028402,
-0.438037767398527));
#49502=CARTESIAN_POINT('Ctrl Pts',(0.0473622336949324,-0.10247889791293,
-0.430962137941886));
#49503=CARTESIAN_POINT('Ctrl Pts',(0.111627772406076,-0.0168625899039329,
-0.423886508485243));
#49504=CARTESIAN_POINT('Ctrl Pts',(0.0755192590508171,0.0839163142856434,
-0.416810879028601));
#49505=CARTESIAN_POINT('Ctrl Pts',(-0.0284950580593602,0.109238902681774,
-0.409735249571959));
#49506=CARTESIAN_POINT('Ctrl Pts',(-0.0894235522255543,0.0525762734766696,
-0.404235867621238));
#49507=CARTESIAN_POINT('Ctrl Pts',(-0.0958143038252681,0.0105580020614414,
-0.401095028822731));
#49508=CARTESIAN_POINT('Ctrl Pts',(-0.0957406735922206,7.06966245190514E-5,
-0.400312733176438));
#49509=CARTESIAN_POINT('Origin',(0.,0.,-0.656687266823562));
#49510=CARTESIAN_POINT('',(-0.095796229339445,8.13944495619803E-5,-0.499187266823562));
#49511=CARTESIAN_POINT('',(-0.0957047411432482,-5.19454942728911E-5,-0.490312733176438));
#49512=CARTESIAN_POINT('',(-0.095825,-8.02710626669594E-15,-0.656687266823562));
#49513=CARTESIAN_POINT('Ctrl Pts',(-0.095796229339445,8.13944495619877E-5,
-0.499187266823562));
#49514=CARTESIAN_POINT('Ctrl Pts',(-0.0955964171293276,-0.0231944520604812,
-0.497448375816877));
#49515=CARTESIAN_POINT('Ctrl Pts',(-0.075437632712349,-0.0783490658574657,
-0.493350941657977));
#49516=CARTESIAN_POINT('Ctrl Pts',(0.0163731327305643,-0.111701819859221,
-0.486894964346863));
#49517=CARTESIAN_POINT('Ctrl Pts',(0.10226912842285,-0.0478115777644791,
-0.479819334890221));
#49518=CARTESIAN_POINT('Ctrl Pts',(0.0962085431136162,0.0590682350665474,
-0.472743705433579));
#49519=CARTESIAN_POINT('Ctrl Pts',(0.00363743500867127,0.112835759078637,
-0.465668075976936));
#49520=CARTESIAN_POINT('Ctrl Pts',(-0.0801464535262578,0.0711425571216517,
-0.459482596440265));
#49521=CARTESIAN_POINT('Ctrl Pts',(-0.0956035338609357,0.0196446182990092,
-0.455655660055807));
#49522=CARTESIAN_POINT('Ctrl Pts',(-0.0957106322133127,-5.59492053251263E-5,
-0.454187266823563));
#49523=CARTESIAN_POINT('Ctrl Pts',(-0.0957047411432482,-5.1945494272879E-5,
-0.490312733176438));
#49524=CARTESIAN_POINT('Ctrl Pts',(-0.0957664443284886,-0.0123322917923352,
-0.489397546649299));
#49525=CARTESIAN_POINT('Ctrl Pts',(-0.0879063054038062,-0.0561846157158543,
-0.486123816969947));
#49526=CARTESIAN_POINT('Ctrl Pts',(-0.0223731015898872,-0.110655243614886,
-0.48049154413838));
#49527=CARTESIAN_POINT('Ctrl Pts',(0.0800710122382963,-0.0795846175196028,
-0.473415914681738));
#49528=CARTESIAN_POINT('Ctrl Pts',(0.110516738602258,0.023046994991323,
-0.466340285225096));
#49529=CARTESIAN_POINT('Ctrl Pts',(0.041587290010598,0.104955262561484,
-0.459264655768454));
#49530=CARTESIAN_POINT('Ctrl Pts',(-0.0637382953975096,0.0926062780139632,
-0.452255471752234));
#49531=CARTESIAN_POINT('Ctrl Pts',(-0.0959012432337274,0.0305203435488716,
-0.447604830888229));
#49532=CARTESIAN_POINT('Ctrl Pts',(-0.0959720410064835,-1.57534720231178E-5,
-0.445312733176438));
#49533=CARTESIAN_POINT('Origin',(0.,0.,-0.656687266823562));
#49534=CARTESIAN_POINT('',(-0.095825,-8.02710626669594E-15,-0.5435));
#49535=CARTESIAN_POINT('',(-0.0957990153585407,7.37030635558182E-5,-0.535312733176437));
#49536=CARTESIAN_POINT('',(-0.095825,-8.02710626669594E-15,-0.656687266823562));
#49537=CARTESIAN_POINT('',(-0.0953841396803776,-0.00918131376406525,-0.5435));
#49538=CARTESIAN_POINT('Origin',(0.,0.,-0.5435));
#49539=CARTESIAN_POINT('Ctrl Pts',(-0.0953841396803776,-0.00918131376406524,
-0.5435));
#49540=CARTESIAN_POINT('Ctrl Pts',(-0.0923605976477055,-0.0405927177292199,
-0.541141456847786));
#49541=CARTESIAN_POINT('Ctrl Pts',(-0.0529443191752485,-0.0996768450839476,
-0.536424370543358));
#49542=CARTESIAN_POINT('Ctrl Pts',(0.0542885591219757,-0.0990657329549278,
-0.529348741086716));
#49543=CARTESIAN_POINT('Ctrl Pts',(0.112485789500799,-0.00919905073578263,
-0.522273111630074));
#49544=CARTESIAN_POINT('Ctrl Pts',(0.0696476756938639,0.0888493431316701,
-0.515197482173432));
#49545=CARTESIAN_POINT('Ctrl Pts',(-0.0358739599293379,0.107052680846593,
-0.508121852716789));
#49546=CARTESIAN_POINT('Ctrl Pts',(-0.0911102694613287,0.0481602885445596,
-0.502785114266833));
#49547=CARTESIAN_POINT('Ctrl Pts',(-0.0958674322292328,0.00837572007059505,
-0.499806918969091));
#49548=CARTESIAN_POINT('Ctrl Pts',(-0.095796229339445,8.13944495619877E-5,
-0.499187266823562));
#49549=CARTESIAN_POINT('Ctrl Pts',(-0.0957990153585407,7.3703063555813E-5,
-0.535312733176437));
#49550=CARTESIAN_POINT('Ctrl Pts',(-0.0955942319159112,-0.0235299141747378,
-0.533548805562583));
#49551=CARTESIAN_POINT('Ctrl Pts',(-0.0749791628368817,-0.0789981539215374,
-0.529426334796515));
#49552=CARTESIAN_POINT('Ctrl Pts',(0.0175496669572723,-0.111531282490646,
-0.522945320878233));
#49553=CARTESIAN_POINT('Ctrl Pts',(0.102761745137553,-0.0467325866898933,
-0.515869691421591));
#49554=CARTESIAN_POINT('Ctrl Pts',(0.0955854583748553,0.0600719067187621,
-0.508794061964948));
#49555=CARTESIAN_POINT('Ctrl Pts',(0.00245303643899368,0.11286876447647,
-0.501718432508308));
#49556=CARTESIAN_POINT('Ctrl Pts',(-0.0805504964401501,0.0704700920038005,
-0.495557989578802));
#49557=CARTESIAN_POINT('Ctrl Pts',(-0.095607427974223,0.0193156027179515,
-0.491756089801513));
#49558=CARTESIAN_POINT('Ctrl Pts',(-0.0957047411432482,-5.1945494272879E-5,
-0.490312733176438));
#49559=CARTESIAN_POINT('Origin',(1.13809670924099E-17,0.,-0.0135));
#49560=CARTESIAN_POINT('',(-0.0872731800879825,-0.0845318995251531,-0.0135));
#49561=CARTESIAN_POINT('Ctrl Pts',(-0.0256835729485001,0.0924624001170202,
-0.0134999999999999));
#49562=CARTESIAN_POINT('Ctrl Pts',(-0.0286929696929738,0.0920530644409703,
-0.0134999999999999));
#49563=CARTESIAN_POINT('Ctrl Pts',(-0.0316740080847999,0.0914938944008697,
-0.0135000000000002));
#49564=CARTESIAN_POINT('Ctrl Pts',(-0.0346156128527234,0.0907835000445219,
-0.0135000000000001));
#49565=CARTESIAN_POINT('Ctrl Pts',(-0.0386263660453573,0.0898149075048917,
-0.0135000000000001));
#49566=CARTESIAN_POINT('Ctrl Pts',(-0.0425638695384247,0.0885654375663179,
-0.0135));
#49567=CARTESIAN_POINT('Ctrl Pts',(-0.0464123421802407,0.0870586227379721,
-0.0135));
#49568=CARTESIAN_POINT('Ctrl Pts',(-0.0499619860475324,0.0856688100739905,
-0.0134999999999999));
#49569=CARTESIAN_POINT('Ctrl Pts',(-0.053437219658575,0.0840585579962781,
-0.0135000000000001));
#49570=CARTESIAN_POINT('Ctrl Pts',(-0.05680648974238,0.0822549280939232,
-0.0135000000000001));
#49571=CARTESIAN_POINT('Ctrl Pts',(-0.0607057413385475,0.0801675897088359,
-0.0135000000000001));
#49572=CARTESIAN_POINT('Ctrl Pts',(-0.0644691098509119,0.0778193898967427,
-0.0135));
#49573=CARTESIAN_POINT('Ctrl Pts',(-0.0680778405577365,0.0752361825612141,
-0.0135));
#49574=CARTESIAN_POINT('Ctrl Pts',(-0.0716069103383439,0.0727099982361779,
-0.0135000000000001));
#49575=CARTESIAN_POINT('Ctrl Pts',(-0.0749921954747181,0.0699544156545884,
-0.0135000000000001));
#49576=CARTESIAN_POINT('Ctrl Pts',(-0.0781906931260397,0.0670135871053226,
-0.0135000000000001));
#49577=CARTESIAN_POINT('Ctrl Pts',(-0.0841982556543313,0.0614899903043682,
-0.0135));
#49578=CARTESIAN_POINT('Ctrl Pts',(-0.0895641926404807,0.0553073555873199,
-0.0135000000000001));
#49579=CARTESIAN_POINT('Ctrl Pts',(-0.09417415447868,0.0486046086051259,
-0.0135000000000001));
#49580=CARTESIAN_POINT('Ctrl Pts',(-0.0960082526817258,0.0459378845351681,
-0.0135000000000001));
#49581=CARTESIAN_POINT('Ctrl Pts',(-0.097722436957705,0.0431883046963393,
-0.0135000000000001));
#49582=CARTESIAN_POINT('Ctrl Pts',(-0.0993080945262219,0.0403628223276675,
-0.0135));
#49583=CARTESIAN_POINT('Ctrl Pts',(-0.100621192866324,0.0380230131015422,
-0.0135));
#49584=CARTESIAN_POINT('Ctrl Pts',(-0.101841576040244,0.0356391671272654,
-0.0135));
#49585=CARTESIAN_POINT('Ctrl Pts',(-0.102965121363602,0.0332172590887685,
-0.0135));
#49586=CARTESIAN_POINT('Ctrl Pts',(-0.104411047879092,0.0301004279488587,
-0.0135));
#49587=CARTESIAN_POINT('Ctrl Pts',(-0.105696927631408,0.0269200665199215,
-0.0135000000000001));
#49588=CARTESIAN_POINT('Ctrl Pts',(-0.106814378879639,0.0236857924562531,
-0.0135000000000001));
#49589=CARTESIAN_POINT('Ctrl Pts',(-0.10872275852689,0.0181623096139294,
-0.0135000000000001));
#49590=CARTESIAN_POINT('Ctrl Pts',(-0.110140714954151,0.0124819005222567,
-0.0135));
#49591=CARTESIAN_POINT('Ctrl Pts',(-0.111089665498783,0.00669929876611018,
-0.0135));
#49592=CARTESIAN_POINT('Ctrl Pts',(-0.111763452113654,0.00259345817783101,
-0.0135));
#49593=CARTESIAN_POINT('Ctrl Pts',(-0.112200243379474,-0.00157061108088781,
-0.0135000000000001));
#49594=CARTESIAN_POINT('Ctrl Pts',(-0.112403879549441,-0.00573895849727011,
-0.0135000000000001));
#49595=CARTESIAN_POINT('Ctrl Pts',(-0.112746158071992,-0.0127452570118909,
-0.0135));
#49596=CARTESIAN_POINT('Ctrl Pts',(-0.112435256625197,-0.0197769752940045,
-0.0135000000000001));
#49597=CARTESIAN_POINT('Ctrl Pts',(-0.111507238982716,-0.0267440426387617,
-0.0135000000000001));
#49598=CARTESIAN_POINT('Ctrl Pts',(-0.110923739318404,-0.0311246505828438,
-0.0135));
#49599=CARTESIAN_POINT('Ctrl Pts',(-0.110095815737416,-0.0354799462789394,
-0.0134999999999999));
#49600=CARTESIAN_POINT('Ctrl Pts',(-0.109027864350346,-0.0397884631534964,
-0.0134999999999999));
#49601=CARTESIAN_POINT('Ctrl Pts',(-0.108289706193421,-0.0427664703116023,
-0.0134999999999999));
#49602=CARTESIAN_POINT('Ctrl Pts',(-0.107435885652299,-0.0457239504344895,
-0.0135000000000001));
#49603=CARTESIAN_POINT('Ctrl Pts',(-0.10647336946096,-0.0486369389278256,
-0.0135000000000001));
#49604=CARTESIAN_POINT('Ctrl Pts',(-0.10365954094822,-0.0571527957555754,
-0.0134999999999999));
#49605=CARTESIAN_POINT('Ctrl Pts',(-0.09991451527938,-0.0653187550302201,
-0.0135000000000001));
#49606=CARTESIAN_POINT('Ctrl Pts',(-0.0952853579514916,-0.0729633148625617,
-0.0135000000000002));
#49607=CARTESIAN_POINT('Ctrl Pts',(-0.0928581545785142,-0.0769715824792622,
-0.0135000000000003));
#49608=CARTESIAN_POINT('Ctrl Pts',(-0.0901870237235777,-0.0808365421038318,
-0.0135000000000001));
#49609=CARTESIAN_POINT('Ctrl Pts',(-0.0872731800879837,-0.0845318995251519,
-0.0135000000000001));
#49610=CARTESIAN_POINT('',(-0.1215,-1.48794586096403E-17,-0.0135));
#49611=CARTESIAN_POINT('Origin',(0.,0.,-0.0135));
#49612=CARTESIAN_POINT('',(0.0125914725202458,-0.12102200839196,-0.0134999999999998));
#49613=CARTESIAN_POINT('Origin',(0.,0.,-0.0135));
#49614=CARTESIAN_POINT('Ctrl Pts',(0.0125914725202424,-0.12102200839196,
-0.0134999999999999));
#49615=CARTESIAN_POINT('Ctrl Pts',(0.01630909845269,-0.120270541987533,
-0.0134999999999999));
#49616=CARTESIAN_POINT('Ctrl Pts',(0.0199811919896631,-0.119336381645409,
-0.0135));
#49617=CARTESIAN_POINT('Ctrl Pts',(0.0235953222232064,-0.118214550041642,
-0.0135));
#49618=CARTESIAN_POINT('Ctrl Pts',(0.0298728004468691,-0.116266011110226,
-0.0135000000000001));
#49619=CARTESIAN_POINT('Ctrl Pts',(0.0359760464873946,-0.113751796213398,
-0.0135000000000001));
#49620=CARTESIAN_POINT('Ctrl Pts',(0.0418497129701972,-0.110722148829279,
-0.0135000000000002));
#49621=CARTESIAN_POINT('Ctrl Pts',(0.0452658144899046,-0.108960117725986,
-0.0135000000000003));
#49622=CARTESIAN_POINT('Ctrl Pts',(0.0485961822757404,-0.107027418200187,
-0.0134999999999999));
#49623=CARTESIAN_POINT('Ctrl Pts',(0.0518253785851629,-0.104937954428778,
-0.0134999999999999));
#49624=CARTESIAN_POINT('Ctrl Pts',(0.0558573654441519,-0.102329041974594,
-0.0134999999999999));
#49625=CARTESIAN_POINT('Ctrl Pts',(0.0597343728416072,-0.0994744335231951,
-0.0135000000000001));
#49626=CARTESIAN_POINT('Ctrl Pts',(0.0634335156525812,-0.0963933155043625,
-0.0135000000000001));
#49627=CARTESIAN_POINT('Ctrl Pts',(0.0666996161571287,-0.0936728903599141,
-0.0135000000000001));
#49628=CARTESIAN_POINT('Ctrl Pts',(0.0698300587296424,-0.0907719367810035,
-0.0135));
#49629=CARTESIAN_POINT('Ctrl Pts',(0.0727869511219022,-0.0877247167350274,
-0.0135));
#49630=CARTESIAN_POINT('Ctrl Pts',(0.0787244614333784,-0.0816058263446699,
-0.0135));
#49631=CARTESIAN_POINT('Ctrl Pts',(0.0839828754633012,-0.0748863675200879,
-0.0135));
#49632=CARTESIAN_POINT('Ctrl Pts',(0.0884251702134852,-0.0676735386298863,
-0.0135000000000001));
#49633=CARTESIAN_POINT('Ctrl Pts',(0.0901937988706099,-0.0648018660841556,
-0.0135000000000001));
#49634=CARTESIAN_POINT('Ctrl Pts',(0.0918325225091036,-0.0618517952811021,
-0.0135));
#49635=CARTESIAN_POINT('Ctrl Pts',(0.0933302931359342,-0.0588296707391292,
-0.0134999999999999));
#49636=CARTESIAN_POINT('Ctrl Pts',(0.0944446233987782,-0.0565812324436539,
-0.0134999999999999));
#49637=CARTESIAN_POINT('Ctrl Pts',(0.0954796740979294,-0.054294932786333,
-0.0135));
#49638=CARTESIAN_POINT('Ctrl Pts',(0.0964281978132539,-0.0519815122319335,
-0.0135000000000001));
#49639=CARTESIAN_POINT('Ctrl Pts',(0.0979408892394924,-0.0482921037528562,
-0.0135000000000001));
#49640=CARTESIAN_POINT('Ctrl Pts',(0.0992365826214292,-0.0445280346329004,
-0.0135000000000001));
#49641=CARTESIAN_POINT('Ctrl Pts',(0.100299532825755,-0.040700640312293,
-0.0135000000000001));
#49642=CARTESIAN_POINT('Ctrl Pts',(0.101687029451378,-0.0357046426793301,
-0.0135000000000001));
#49643=CARTESIAN_POINT('Ctrl Pts',(0.102678183721985,-0.0306005696481754,
-0.0135000000000001));
#49644=CARTESIAN_POINT('Ctrl Pts',(0.103279392849383,-0.0254317444710534,
-0.0135000000000001));
#49645=CARTESIAN_POINT('Ctrl Pts',(0.103615422494957,-0.0225427688831181,
-0.0135000000000001));
#49646=CARTESIAN_POINT('Ctrl Pts',(0.103829532743543,-0.0196319843360579,
-0.0135000000000001));
#49647=CARTESIAN_POINT('Ctrl Pts',(0.103921664321782,-0.0167123916178717,
-0.0135000000000001));
#49648=CARTESIAN_POINT('Ctrl Pts',(0.104174258631648,-0.00870783420299761,
-0.0135000000000001));
#49649=CARTESIAN_POINT('Ctrl Pts',(0.103512737427135,-0.00070037618932715,
-0.0135000000000001));
#49650=CARTESIAN_POINT('Ctrl Pts',(0.101968203321781,0.00714835440083033,
-0.0135000000000002));
#49651=CARTESIAN_POINT('Ctrl Pts',(0.101237186149509,0.0108631036071164,
-0.0135000000000003));
#49652=CARTESIAN_POINT('Ctrl Pts',(0.100307649317537,0.0145420857439938,
-0.0135));
#49653=CARTESIAN_POINT('Ctrl Pts',(0.0991794056182389,0.0181660256448864,
-0.0135));
#49654=CARTESIAN_POINT('Ctrl Pts',(0.098236594455864,0.0211943527629211,
-0.0135));
#49655=CARTESIAN_POINT('Ctrl Pts',(0.0971539272984628,0.0241854881404279,
-0.0135));
#49656=CARTESIAN_POINT('Ctrl Pts',(0.0959395234098873,0.0271085791501241,
-0.0135));
#49657=CARTESIAN_POINT('Ctrl Pts',(0.0930741567527453,0.0340055658888603,
-0.0135000000000001));
#49658=CARTESIAN_POINT('Ctrl Pts',(0.0894707573383288,0.0405524725288617,
-0.0135000000000001));
#49659=CARTESIAN_POINT('Ctrl Pts',(0.0851332279891031,0.046597744453004,
-0.0135000000000002));
#49660=CARTESIAN_POINT('Ctrl Pts',(0.0832222855077887,0.0492610502201462,
-0.0135000000000002));
#49661=CARTESIAN_POINT('Ctrl Pts',(0.0811684147236789,0.0518265208596175,
-0.0135));
#49662=CARTESIAN_POINT('Ctrl Pts',(0.0789701248920227,0.0542784487576638,
-0.0135000000000001));
#49663=CARTESIAN_POINT('Ctrl Pts',(0.0955814485598029,-0.00682768747159289,
-0.558323468161444));
#49664=CARTESIAN_POINT('Ctrl Pts',(0.0978299067420195,0.024648693217557,
-0.55596492500923));
#49665=CARTESIAN_POINT('Ctrl Pts',(0.0688009783410032,0.0894707042253711,
-0.551247838704802));
#49666=CARTESIAN_POINT('Ctrl Pts',(-0.0370370537006431,0.106721729527787,
-0.54417220924816));
#49667=CARTESIAN_POINT('Ctrl Pts',(-0.109384159856722,0.0277988167736781,
-0.537096579791517));
#49668=CARTESIAN_POINT('Ctrl Pts',(-0.0834684332867814,-0.0760133271640939,
-0.530020950334875));
#49669=CARTESIAN_POINT('Ctrl Pts',(0.0175496669572723,-0.111531282490646,
-0.522945320878233));
#49670=CARTESIAN_POINT('Ctrl Pts',(0.102761745137553,-0.0467325866898933,
-0.515869691421591));
#49671=CARTESIAN_POINT('Ctrl Pts',(0.0955854583748553,0.0600719067187621,
-0.508794061964948));
#49672=CARTESIAN_POINT('Ctrl Pts',(0.00245303643899368,0.11286876447647,
-0.501718432508308));
#49673=CARTESIAN_POINT('Ctrl Pts',(-0.0928813817133624,0.0641714062989615,
-0.494642803051664));
#49674=CARTESIAN_POINT('Ctrl Pts',(-0.104700197801406,-0.0422256787109809,
-0.487567173595023));
#49675=CARTESIAN_POINT('Ctrl Pts',(-0.0223731015898872,-0.110655243614886,
-0.48049154413838));
#49676=CARTESIAN_POINT('Ctrl Pts',(0.0800710122382963,-0.0795846175196028,
-0.473415914681738));
#49677=CARTESIAN_POINT('Ctrl Pts',(0.110516738602258,0.023046994991323,
-0.466340285225096));
#49678=CARTESIAN_POINT('Ctrl Pts',(0.041587290010598,0.104955262561484,
-0.459264655768454));
#49679=CARTESIAN_POINT('Ctrl Pts',(-0.0647367575428925,0.0924892125017532,
-0.452189026311811));
#49680=CARTESIAN_POINT('Ctrl Pts',(-0.11285050815591,-0.00314172710120585,
-0.44511339685517));
#49681=CARTESIAN_POINT('Ctrl Pts',(-0.0594907218526991,-0.0959476973028402,
-0.438037767398527));
#49682=CARTESIAN_POINT('Ctrl Pts',(0.0473622336949324,-0.10247889791293,
-0.430962137941886));
#49683=CARTESIAN_POINT('Ctrl Pts',(0.111627772406076,-0.0168625899039329,
-0.423886508485243));
#49684=CARTESIAN_POINT('Ctrl Pts',(0.0755192590508171,0.0839163142856434,
-0.416810879028601));
#49685=CARTESIAN_POINT('Ctrl Pts',(-0.0284950580593602,0.109238902681774,
-0.409735249571959));
#49686=CARTESIAN_POINT('Ctrl Pts',(-0.106887039546414,0.0363354797358826,
-0.402659620115318));
#49687=CARTESIAN_POINT('Ctrl Pts',(-0.0891677688863871,-0.069240271962092,
-0.395583990658674));
#49688=CARTESIAN_POINT('Ctrl Pts',(0.00872984600194528,-0.112556190631666,
-0.388508361202033));
#49689=CARTESIAN_POINT('Ctrl Pts',(0.0987777120733966,-0.054663240617283,
-0.38143273174539));
#49690=CARTESIAN_POINT('Ctrl Pts',(0.100006114225775,0.0523820903322742,
-0.374357102288749));
#49691=CARTESIAN_POINT('Ctrl Pts',(0.0113104914411958,0.112326217122388,
-0.367281472832106));
#49692=CARTESIAN_POINT('Ctrl Pts',(-0.0875553586799717,0.0712682638930122,
-0.360205843375464));
#49693=CARTESIAN_POINT('Ctrl Pts',(-0.107692719823917,-0.0338730625668669,
-0.353130213918822));
#49694=CARTESIAN_POINT('Ctrl Pts',(-0.0309943734581772,-0.108556230059475,
-0.34605458446218));
#49695=CARTESIAN_POINT('Ctrl Pts',(0.0735736570237532,-0.0856272343546855,
-0.338978955005538));
#49696=CARTESIAN_POINT('Ctrl Pts',(0.111985338737018,0.0142965093240165,
-0.331903325548895));
#49697=CARTESIAN_POINT('Ctrl Pts',(0.0497014532331962,0.101365042383611,
-0.324827696092254));
#49698=CARTESIAN_POINT('Ctrl Pts',(-0.0572732469911756,0.0972876222859135,
-0.317752066635611));
#49699=CARTESIAN_POINT('Ctrl Pts',(-0.112748687069072,0.00573060512783594,
-0.310676437178969));
#49700=CARTESIAN_POINT('Ctrl Pts',(-0.0668421683520032,-0.0909792877579244,
-0.303600807722327));
#49701=CARTESIAN_POINT('Ctrl Pts',(0.0391678436633201,-0.105881945078975,
-0.296525178265685));
#49702=CARTESIAN_POINT('Ctrl Pts',(0.109958707539584,-0.02557711686569,
-0.289449548809043));
#49703=CARTESIAN_POINT('Ctrl Pts',(0.0818763211215267,0.07772627812099,
-0.2823739193524));
#49704=CARTESIAN_POINT('Ctrl Pts',(-0.0198280473347807,0.111139348611692,
-0.275298289895759));
#49705=CARTESIAN_POINT('Ctrl Pts',(-0.103703327664771,0.0446175537450222,
-0.268222660439116));
#49706=CARTESIAN_POINT('Ctrl Pts',(-0.0943301031515697,-0.0620236883000746,
-0.261147030982475));
#49707=CARTESIAN_POINT('Ctrl Pts',(-0.000136639224089264,-0.112894143340924,
-0.254071401525832));
#49708=CARTESIAN_POINT('Ctrl Pts',(0.0941796886812631,-0.0622518474490773,
-0.24699577206919));
#49709=CARTESIAN_POINT('Ctrl Pts',(0.103811027648513,0.0443663927929224,
-0.239920142612548));
#49710=CARTESIAN_POINT('Ctrl Pts',(0.0200970195336817,0.111091026086466,
-0.232844513155906));
#49711=CARTESIAN_POINT('Ctrl Pts',(-0.0816879325475845,0.0779242449234631,
-0.225768883699263));
#49712=CARTESIAN_POINT('Ctrl Pts',(-0.110020298820829,-0.0253108695644216,
-0.218693254242622));
#49713=CARTESIAN_POINT('Ctrl Pts',(-0.0394240328282805,-0.105786822938669,
-0.211617624785979));
#49714=CARTESIAN_POINT('Ctrl Pts',(0.0666217428299838,-0.0911408231911627,
-0.204541995329337));
#49715=CARTESIAN_POINT('Ctrl Pts',(0.112762228567538,0.00545766237499973,
-0.197466365872695));
#49716=CARTESIAN_POINT('Ctrl Pts',(0.0575085792042569,0.0971486983708248,
-0.190390736416053));
#49717=CARTESIAN_POINT('Ctrl Pts',(-0.0494559375846015,0.101485055541974,
-0.183315106959411));
#49718=CARTESIAN_POINT('Ctrl Pts',(-0.111950403671619,0.0145675456862952,
-0.176239477502769));
#49719=CARTESIAN_POINT('Ctrl Pts',(-0.0737807157070053,-0.0854488870635276,
-0.169163848046127));
#49720=CARTESIAN_POINT('Ctrl Pts',(0.0307315052759879,-0.108630938394162,
-0.162088218589485));
#49721=CARTESIAN_POINT('Ctrl Pts',(0.107610409091042,-0.0341336512276352,
-0.155012589132842));
#49722=CARTESIAN_POINT('Ctrl Pts',(0.087727618468951,0.0710561149260017,
-0.147936959676201));
#49723=CARTESIAN_POINT('Ctrl Pts',(-0.0110385554953438,0.112353264263208,
-0.140861330219558));
#49724=CARTESIAN_POINT('Ctrl Pts',(-0.0998790212114998,0.0526240223292122,
-0.133785700762916));
#49725=CARTESIAN_POINT('Ctrl Pts',(-0.0989097454024145,-0.054423982807721,
-0.126710071306274));
#49726=CARTESIAN_POINT('Ctrl Pts',(-0.00900227708678451,-0.112534711150002,
-0.119634441849632));
#49727=CARTESIAN_POINT('Ctrl Pts',(0.0889998943616218,-0.0694559474299769,
-0.11255881239299));
#49728=CARTESIAN_POINT('Ctrl Pts',(0.106974694106382,0.0360767003792724,
-0.105483182936348));
#49729=CARTESIAN_POINT('Ctrl Pts',(0.0287593818097131,0.109169484310085,
-0.0984075534797054));
#49730=CARTESIAN_POINT('Ctrl Pts',(-0.0753158619846615,0.0840991055108705,
-0.0913319240230634));
#49731=CARTESIAN_POINT('Ctrl Pts',(-0.111668345874976,-0.016592766249281,
-0.0842562945664211));
#49732=CARTESIAN_POINT('Ctrl Pts',(-0.0476100055917889,-0.102363117493165,
-0.0771806651097791));
#49733=CARTESIAN_POINT('Ctrl Pts',(0.0592579954685063,-0.0960930036749314,
-0.0701050356531369));
#49734=CARTESIAN_POINT('Ctrl Pts',(0.112843133809849,-0.00341188826479888,
-0.0630294061964947));
#49735=CARTESIAN_POINT('Ctrl Pts',(0.064959386513852,0.0923265347892355,
-0.0559537767398527));
#49736=CARTESIAN_POINT('Ctrl Pts',(-0.04133108222025,0.105066452432841,
-0.0488781472832105));
#49737=CARTESIAN_POINT('Ctrl Pts',(-0.110464478017885,0.023293869539893,
-0.0418025178265684));
#49738=CARTESIAN_POINT('Ctrl Pts',(-0.0802560572708783,-0.0793513321432661,
-0.0347268883699262));
#49739=CARTESIAN_POINT('Ctrl Pts',(0.022090743255976,-0.110784791206306,
-0.0276512589132841));
#49740=CARTESIAN_POINT('Ctrl Pts',(0.104628794236781,-0.0423248975405764,
-0.0205756294566421));
#49741=CARTESIAN_POINT('Ctrl Pts',(0.0968448185910171,0.0282724219436266,
-0.0158585431522139));
#49742=CARTESIAN_POINT('Ctrl Pts',(0.0789701248920212,0.0542784487576661,
-0.0134999999999998));
#49743=CARTESIAN_POINT('Ctrl Pts',(0.104118029799121,-0.00743748267407433,
-0.553382312107629));
#49744=CARTESIAN_POINT('Ctrl Pts',(0.10656730253505,0.0268501201185417,
-0.551023768955415));
#49745=CARTESIAN_POINT('Ctrl Pts',(0.0749457391685725,0.097461521969475,
-0.546306682650987));
#49746=CARTESIAN_POINT('Ctrl Pts',(-0.0403449112665664,0.116253272811989,
-0.539231053194345));
#49747=CARTESIAN_POINT('Ctrl Pts',(-0.119153490422236,0.030281587869128,
-0.532155423737704));
#49748=CARTESIAN_POINT('Ctrl Pts',(-0.0909231755239786,-0.0828022381126562,
-0.52507979428106));
#49749=CARTESIAN_POINT('Ctrl Pts',(0.0191170648149215,-0.121492377117822,
-0.518004164824419));
#49750=CARTESIAN_POINT('Ctrl Pts',(0.111939613844073,-0.0509063728043841,
-0.510928535367777));
#49751=CARTESIAN_POINT('Ctrl Pts',(0.104122397739233,0.0654370557056445,
-0.503852905911134));
#49752=CARTESIAN_POINT('Ctrl Pts',(0.00267212230931772,0.122949312447366,
-0.496777276454493));
#49753=CARTESIAN_POINT('Ctrl Pts',(-0.101176814274421,0.0699026902600922,
-0.489701646997849));
#49754=CARTESIAN_POINT('Ctrl Pts',(-0.114051193813411,-0.0459969433458333,
-0.482626017541209));
#49755=CARTESIAN_POINT('Ctrl Pts',(-0.024371290591785,-0.120538097358036,
-0.475550388084565));
#49756=CARTESIAN_POINT('Ctrl Pts',(0.0872223236191749,-0.0866924879598705,
-0.468474758627924));
#49757=CARTESIAN_POINT('Ctrl Pts',(0.120387222169918,0.0251053708375774,
-0.461399129171281));
#49758=CARTESIAN_POINT('Ctrl Pts',(0.0453015388010052,0.114329038946442,
-0.454323499714639));
#49759=CARTESIAN_POINT('Ctrl Pts',(-0.0705185342188244,0.100749619601441,
-0.447247870257997));
#49760=CARTESIAN_POINT('Ctrl Pts',(-0.122929425616221,-0.00342232139052918,
-0.440172240801355));
#49761=CARTESIAN_POINT('Ctrl Pts',(-0.0648039639905137,-0.104516988991684,
-0.433096611344713));
#49762=CARTESIAN_POINT('Ctrl Pts',(0.0515922549145764,-0.111631504935852,
-0.426020981888072));
#49763=CARTESIAN_POINT('Ctrl Pts',(0.121597484751588,-0.0183686234574026,
-0.418945352431428));
#49764=CARTESIAN_POINT('Ctrl Pts',(0.0822640437316759,0.0914110577217115,
-0.411869722974788));
#49765=CARTESIAN_POINT('Ctrl Pts',(-0.031040011935954,0.118995260021906,
-0.404794093518143));
#49766=CARTESIAN_POINT('Ctrl Pts',(-0.116433347017861,0.0395806782478192,
-0.397718464061503));
#49767=CARTESIAN_POINT('Ctrl Pts',(-0.0971315308349326,-0.0754242670316685,
-0.390642834604859));
#49768=CARTESIAN_POINT('Ctrl Pts',(0.0095095270041183,-0.122608821971672,
-0.383567205148219));
#49769=CARTESIAN_POINT('Ctrl Pts',(0.107599758364324,-0.0595453302001996,
-0.376491575691576));
#49770=CARTESIAN_POINT('Ctrl Pts',(0.108937871709893,0.0570604455606625,
-0.369415946234934));
#49771=CARTESIAN_POINT('Ctrl Pts',(0.0123206553432845,0.122358309042094,
-0.362340316778292));
#49772=CARTESIAN_POINT('Ctrl Pts',(-0.09537511286419,0.077633383209312,
-0.35526468732165));
#49773=CARTESIAN_POINT('Ctrl Pts',(-0.117310984304234,-0.0368983373956488,
-0.348189057865008));
#49774=CARTESIAN_POINT('Ctrl Pts',(-0.0337625464768359,-0.118251616464473,
-0.341113428408365));
#49775=CARTESIAN_POINT('Ctrl Pts',(0.0801446758743825,-0.0932747836791719,
-0.334037798951723));
#49776=CARTESIAN_POINT('Ctrl Pts',(0.121986986087476,0.0155733607959493,
-0.326962169495081));
#49777=CARTESIAN_POINT('Ctrl Pts',(0.0541403950951408,0.11041816861441,
-0.319886540038439));
#49778=CARTESIAN_POINT('Ctrl Pts',(-0.0623884417611494,0.105976585507727,
-0.312810910581797));
#49779=CARTESIAN_POINT('Ctrl Pts',(-0.122818510672858,0.00624241758685821,
-0.305735281125155));
#49780=CARTESIAN_POINT('Ctrl Pts',(-0.0728119837183407,-0.0991048402866123,
-0.298659651668513));
#49781=CARTESIAN_POINT('Ctrl Pts',(0.0426660065855064,-0.115338485438668,
-0.29158402221187));
#49782=CARTESIAN_POINT('Ctrl Pts',(0.119779352173304,-0.0278614632454685,
-0.284508392755229));
#49783=CARTESIAN_POINT('Ctrl Pts',(0.0891888684553656,0.0846681763408569,
-0.277432763298586));
#49784=CARTESIAN_POINT('Ctrl Pts',(-0.021598932160662,0.121065438795552,
-0.270357133841944));
#49785=CARTESIAN_POINT('Ctrl Pts',(-0.112965291097392,0.048602441795822,
-0.263281504385302));
#49786=CARTESIAN_POINT('Ctrl Pts',(-0.102754924087013,-0.0675631550262395,
-0.25620587492866));
#49787=CARTESIAN_POINT('Ctrl Pts',(-0.000148842762062005,-0.122976957951858,
-0.249130245472017));
#49788=CARTESIAN_POINT('Ctrl Pts',(0.102591075782372,-0.0678116915511916,
-0.242054616015376));
#49789=CARTESIAN_POINT('Ctrl Pts',(0.113082609994372,0.0483288491281101,
-0.234978986558733));
#49790=CARTESIAN_POINT('Ctrl Pts',(0.0218919268352818,0.12101280048344,
-0.227903357102091));
#49791=CARTESIAN_POINT('Ctrl Pts',(-0.0889836544996118,0.0848838239769811,
-0.220827727645449));
#49792=CARTESIAN_POINT('Ctrl Pts',(-0.119846444302087,-0.0275714368348496,
-0.213752098188807));
#49793=CARTESIAN_POINT('Ctrl Pts',(-0.0429450765463997,-0.115234867738913,
-0.206676468732164));
#49794=CARTESIAN_POINT('Ctrl Pts',(0.0725718715269475,-0.0992808027908956,
-0.199600839275523));
#49795=CARTESIAN_POINT('Ctrl Pts',(0.122833261591181,0.00594509773973707,
-0.19252520981888));
#49796=CARTESIAN_POINT('Ctrl Pts',(0.0626447919916975,0.105825254004083,
-0.185449580362239));
#49797=CARTESIAN_POINT('Ctrl Pts',(-0.0538729519249248,0.110548900401667,
-0.178373950905596));
#49798=CARTESIAN_POINT('Ctrl Pts',(-0.12194893089753,0.015868603988742,
-0.171298321448954));
#49799=CARTESIAN_POINT('Ctrl Pts',(-0.0803702274063793,-0.0930805078143962,
-0.164222691992312));
#49800=CARTESIAN_POINT('Ctrl Pts',(0.033476200981565,-0.118332997158473,
-0.15714706253567));
#49801=CARTESIAN_POINT('Ctrl Pts',(0.117221322225793,-0.0371821997806217,
-0.150071433079028));
#49802=CARTESIAN_POINT('Ctrl Pts',(0.095562757539098,0.077402286769553,
-0.142995803622386));
#49803=CARTESIAN_POINT('Ctrl Pts',(-0.012024432223208,0.12238777182024,
-0.135920174165744));
#49804=CARTESIAN_POINT('Ctrl Pts',(-0.108799427749825,0.0573239850157162,
-0.128844544709101));
#49805=CARTESIAN_POINT('Ctrl Pts',(-0.107743583869089,-0.05928470376985,
-0.121768915252459));
#49806=CARTESIAN_POINT('Ctrl Pts',(-0.00980628948509182,-0.12258542411209,
-0.114693285795817));
#49807=CARTESIAN_POINT('Ctrl Pts',(0.0969486630814565,-0.0756592049315504,
-0.107617656339175));
#49808=CARTESIAN_POINT('Ctrl Pts',(0.11652883019189,0.0392987867597841,
-0.100542026882533));
#49809=CARTESIAN_POINT('Ctrl Pts',(0.0313279429992586,0.118919641748685,
-0.093466397425891));
#49810=CARTESIAN_POINT('Ctrl Pts',(-0.0820424808435396,0.0916101744177033,
-0.0863907679692487));
#49811=CARTESIAN_POINT('Ctrl Pts',(-0.121641681922771,-0.0180747012817188,
-0.0793151385126067));
#49812=CARTESIAN_POINT('Ctrl Pts',(-0.0518621558433564,-0.111505383922027,
-0.0722395090559645));
#49813=CARTESIAN_POINT('Ctrl Pts',(0.0645504523209409,-0.104675272983059,
-0.0651638795993224));
#49814=CARTESIAN_POINT('Ctrl Pts',(0.122921392651723,-0.00371661121879128,
-0.0580882501426802));
#49815=CARTESIAN_POINT('Ctrl Pts',(0.0707610466538411,0.100572412798501,
-0.0510126206860381));
#49816=CARTESIAN_POINT('Ctrl Pts',(-0.0450224485512517,0.114450159420278,
-0.043936991229396));
#49817=CARTESIAN_POINT('Ctrl Pts',(-0.120330294082271,0.0253742942739985,
-0.0368613617727538));
#49818=CARTESIAN_POINT('Ctrl Pts',(-0.0874238954148212,-0.086438367373384,
-0.0297857323161117));
#49819=CARTESIAN_POINT('Ctrl Pts',(0.0240637142381377,-0.120679215118723,
-0.0227101028594695));
#49820=CARTESIAN_POINT('Ctrl Pts',(0.113973413045475,-0.0461050236188597,
-0.0156344734028275));
#49821=CARTESIAN_POINT('Ctrl Pts',(0.10549423407871,0.0307974917180502,
-0.0109173870983993));
#49822=CARTESIAN_POINT('Ctrl Pts',(0.0860231136966225,0.0591261717661117,
-0.0085588439461853));
#49823=CARTESIAN_POINT('Ctrl Pts',(0.112654611038439,-0.00804727787655577,
-0.548441156053815));
#49824=CARTESIAN_POINT('Ctrl Pts',(0.11530469832808,0.0290515470195264,
-0.546082612901601));
#49825=CARTESIAN_POINT('Ctrl Pts',(0.0810904999961417,0.105452339713579,
-0.541365526597172));
#49826=CARTESIAN_POINT('Ctrl Pts',(-0.0436527688324896,0.125784816096191,
-0.534289897140531));
#49827=CARTESIAN_POINT('Ctrl Pts',(-0.128922820987751,0.0327643589645776,
-0.527214267683888));
#49828=CARTESIAN_POINT('Ctrl Pts',(-0.0983779177611759,-0.0895911490612184,
-0.520138638227246));
#49829=CARTESIAN_POINT('Ctrl Pts',(0.0206844626725709,-0.131453471744998,
-0.513063008770604));
#49830=CARTESIAN_POINT('Ctrl Pts',(0.121117482550592,-0.0550801589188749,
-0.505987379313962));
#49831=CARTESIAN_POINT('Ctrl Pts',(0.112659337103611,0.0708022046925269,
-0.49891174985732));
#49832=CARTESIAN_POINT('Ctrl Pts',(0.00289120817964168,0.133029860418262,
-0.491836120400678));
#49833=CARTESIAN_POINT('Ctrl Pts',(-0.10947224683548,0.0756339742212229,
-0.484760490944035));
#49834=CARTESIAN_POINT('Ctrl Pts',(-0.123402189825416,-0.0497682079806857,
-0.477684861487394));
#49835=CARTESIAN_POINT('Ctrl Pts',(-0.0263694795936829,-0.130420951101186,
-0.470609232030751));
#49836=CARTESIAN_POINT('Ctrl Pts',(0.0943736350000536,-0.0938003584001382,
-0.463533602574109));
#49837=CARTESIAN_POINT('Ctrl Pts',(0.130257705737577,0.0271637466838317,
-0.456457973117467));
#49838=CARTESIAN_POINT('Ctrl Pts',(0.0490157875914125,0.123702815331401,
-0.449382343660825));
#49839=CARTESIAN_POINT('Ctrl Pts',(-0.0763003108947565,0.109010026701128,
-0.442306714204182));
#49840=CARTESIAN_POINT('Ctrl Pts',(-0.133008343076533,-0.00370291567985249,
-0.435231084747541));
#49841=CARTESIAN_POINT('Ctrl Pts',(-0.0701172061283284,-0.113086280680527,
-0.428155455290898));
#49842=CARTESIAN_POINT('Ctrl Pts',(0.0558222761342205,-0.120784111958774,
-0.421079825834257));
#49843=CARTESIAN_POINT('Ctrl Pts',(0.1315671970971,-0.0198746570108724,
-0.414004196377613));
#49844=CARTESIAN_POINT('Ctrl Pts',(0.0890088284125349,0.0989058011577798,
-0.406928566920972));
#49845=CARTESIAN_POINT('Ctrl Pts',(-0.0335849658125481,0.128751617362039,
-0.39985293746433));
#49846=CARTESIAN_POINT('Ctrl Pts',(-0.125979654489307,0.0428258767597559,
-0.392777308007688));
#49847=CARTESIAN_POINT('Ctrl Pts',(-0.105095292783478,-0.081608262101245,
-0.385701678551046));
#49848=CARTESIAN_POINT('Ctrl Pts',(0.0102892080062914,-0.132661453311677,
-0.378626049094403));
#49849=CARTESIAN_POINT('Ctrl Pts',(0.116421804655251,-0.0644274197831163,
-0.371550419637762));
#49850=CARTESIAN_POINT('Ctrl Pts',(0.117869629194011,0.0617388007890509,
-0.364474790181119));
#49851=CARTESIAN_POINT('Ctrl Pts',(0.0133308192453733,0.132390400961799,
-0.357399160724477));
#49852=CARTESIAN_POINT('Ctrl Pts',(-0.103194867048408,0.0839985025256118,
-0.350323531267834));
#49853=CARTESIAN_POINT('Ctrl Pts',(-0.126929248784551,-0.0399236122244308,
-0.343247901811194));
#49854=CARTESIAN_POINT('Ctrl Pts',(-0.0365307194954948,-0.127947002869472,
-0.33617227235455));
#49855=CARTESIAN_POINT('Ctrl Pts',(0.0867156947250119,-0.100922333003658,
-0.329096642897909));
#49856=CARTESIAN_POINT('Ctrl Pts',(0.131988633437934,0.0168502122678822,
-0.322021013441266));
#49857=CARTESIAN_POINT('Ctrl Pts',(0.0585793369570855,0.11947129484521,
-0.314945383984625));
#49858=CARTESIAN_POINT('Ctrl Pts',(-0.0675036365311233,0.114665548729541,
-0.307869754527982));
#49859=CARTESIAN_POINT('Ctrl Pts',(-0.132888334276644,0.00675423004588044,
-0.30079412507134));
#49860=CARTESIAN_POINT('Ctrl Pts',(-0.0787817990846783,-0.1072303928153,
-0.293718495614698));
#49861=CARTESIAN_POINT('Ctrl Pts',(0.0461641695076928,-0.124795025798362,
-0.286642866158056));
#49862=CARTESIAN_POINT('Ctrl Pts',(0.129599996807024,-0.0301458096252471,
-0.279567236701414));
#49863=CARTESIAN_POINT('Ctrl Pts',(0.0965014157892046,0.0916100745607239,
-0.272491607244771));
#49864=CARTESIAN_POINT('Ctrl Pts',(-0.0233698169865435,0.130991528979412,
-0.26541597778813));
#49865=CARTESIAN_POINT('Ctrl Pts',(-0.122227254530014,0.0525873298466217,
-0.258340348331487));
#49866=CARTESIAN_POINT('Ctrl Pts',(-0.111179745022457,-0.0731026217524041,
-0.251264718874846));
#49867=CARTESIAN_POINT('Ctrl Pts',(-0.000161046300034822,-0.133059772562792,
-0.244189089418203));
#49868=CARTESIAN_POINT('Ctrl Pts',(0.111002462883481,-0.0733715356533056,
-0.237113459961561));
#49869=CARTESIAN_POINT('Ctrl Pts',(0.122354192340231,0.0522913054632976,
-0.230037830504919));
#49870=CARTESIAN_POINT('Ctrl Pts',(0.023686834136882,0.130934574880413,
-0.222962201048277));
#49871=CARTESIAN_POINT('Ctrl Pts',(-0.0962793764516391,0.0918434030304992,
-0.215886571591634));
#49872=CARTESIAN_POINT('Ctrl Pts',(-0.129672589783346,-0.0298320041052777,
-0.208810942134993));
#49873=CARTESIAN_POINT('Ctrl Pts',(-0.0464661202645189,-0.124682912539157,
-0.20173531267835));
#49874=CARTESIAN_POINT('Ctrl Pts',(0.0785220002239111,-0.107420782390629,
-0.194659683221709));
#49875=CARTESIAN_POINT('Ctrl Pts',(0.132904294614823,0.00643253310447447,
-0.187584053765066));
#49876=CARTESIAN_POINT('Ctrl Pts',(0.0677810047791383,0.114501809637341,
-0.180508424308424));
#49877=CARTESIAN_POINT('Ctrl Pts',(-0.0582899662652481,0.119612745261361,
-0.173432794851782));
#49878=CARTESIAN_POINT('Ctrl Pts',(-0.13194745812344,0.0171696622911887,
-0.16635716539514));
#49879=CARTESIAN_POINT('Ctrl Pts',(-0.0869597391057534,-0.100712128565265,
-0.159281535938498));
#49880=CARTESIAN_POINT('Ctrl Pts',(0.036220896687142,-0.128035055922783,
-0.152205906481855));
#49881=CARTESIAN_POINT('Ctrl Pts',(0.126832235360543,-0.0402307483336081,
-0.145130277025213));
#49882=CARTESIAN_POINT('Ctrl Pts',(0.103397896609245,0.0837484586131044,
-0.138054647568571));
#49883=CARTESIAN_POINT('Ctrl Pts',(-0.0130103089510719,0.132422279377272,
-0.130979018111929));
#49884=CARTESIAN_POINT('Ctrl Pts',(-0.117719834288151,0.0620239477022202,
-0.123903388655287));
#49885=CARTESIAN_POINT('Ctrl Pts',(-0.116577422335763,-0.0641454247319789,
-0.116827759198645));
#49886=CARTESIAN_POINT('Ctrl Pts',(-0.0106103018833993,-0.132636137074179,
-0.109752129742003));
#49887=CARTESIAN_POINT('Ctrl Pts',(0.104897431801291,-0.0818624624331239,
-0.102676500285361));
#49888=CARTESIAN_POINT('Ctrl Pts',(0.126082966277398,0.0425208731402957,
-0.0956008708287183));
#49889=CARTESIAN_POINT('Ctrl Pts',(0.0338965041888041,0.128669799187284,
-0.0885252413720764));
#49890=CARTESIAN_POINT('Ctrl Pts',(-0.0887690997024177,0.099121243324536,
-0.0814496119154342));
#49891=CARTESIAN_POINT('Ctrl Pts',(-0.131615017970567,-0.0195566363141564,
-0.0743739824587921));
#49892=CARTESIAN_POINT('Ctrl Pts',(-0.0561143060949239,-0.120647650350888,
-0.0672983530021499));
#49893=CARTESIAN_POINT('Ctrl Pts',(0.0698429091733757,-0.113257542291187,
-0.0602227235455079));
#49894=CARTESIAN_POINT('Ctrl Pts',(0.132999651493598,-0.00402133417278372,
-0.0531470940888656));
#49895=CARTESIAN_POINT('Ctrl Pts',(0.0765627067938301,0.108818290807766,
-0.0460714646322236));
#49896=CARTESIAN_POINT('Ctrl Pts',(-0.0487138148822533,0.123833866407714,
-0.0389958351755814));
#49897=CARTESIAN_POINT('Ctrl Pts',(-0.130196110146656,0.027454719008104,
-0.0319202057189393));
#49898=CARTESIAN_POINT('Ctrl Pts',(-0.094591733558764,-0.0935254026035021,
-0.0248445762622972));
#49899=CARTESIAN_POINT('Ctrl Pts',(0.0260366852202995,-0.13057363903114,
-0.017768946805655));
#49900=CARTESIAN_POINT('Ctrl Pts',(0.123318031854169,-0.0498851496971432,
-0.010693317349013));
#49901=CARTESIAN_POINT('Ctrl Pts',(0.114143649566402,0.0333225614924737,
-0.00597623104458479));
#49902=CARTESIAN_POINT('Ctrl Pts',(0.0930761025012238,0.0639738947745574,
-0.00361768789237075));
#49903=CARTESIAN_POINT('Ctrl Pts',(0.121191192277757,-0.00865707307903722,
-0.5435));
#49904=CARTESIAN_POINT('Ctrl Pts',(0.124042094121111,0.0312529739205111,
-0.541141456847786));
#49905=CARTESIAN_POINT('Ctrl Pts',(0.0872352608237108,0.113443157457683,
-0.536424370543358));
#49906=CARTESIAN_POINT('Ctrl Pts',(-0.0469606263984128,0.135316359380393,
-0.529348741086716));
#49907=CARTESIAN_POINT('Ctrl Pts',(-0.138692151553265,0.0352471300600274,
-0.522273111630074));
#49908=CARTESIAN_POINT('Ctrl Pts',(-0.105832659998373,-0.0963800600097806,
-0.515197482173431));
#49909=CARTESIAN_POINT('Ctrl Pts',(0.02225186053022,-0.141414566372174,
-0.50812185271679));
#49910=CARTESIAN_POINT('Ctrl Pts',(0.130295351257111,-0.0592539450333656,
-0.501046223260147));
#49911=CARTESIAN_POINT('Ctrl Pts',(0.121196276467989,0.0761673536794093,
-0.493970593803505));
#49912=CARTESIAN_POINT('Ctrl Pts',(0.00311029404996583,0.143110408389158,
-0.486894964346863));
#49913=CARTESIAN_POINT('Ctrl Pts',(-0.117767679396539,0.0813652581823536,
-0.479819334890221));
#49914=CARTESIAN_POINT('Ctrl Pts',(-0.132753185837421,-0.0535394726155382,
-0.472743705433579));
#49915=CARTESIAN_POINT('Ctrl Pts',(-0.0283676685955808,-0.140303804844337,
-0.465668075976936));
#49916=CARTESIAN_POINT('Ctrl Pts',(0.101524946380932,-0.100908228840406,
-0.458592446520295));
#49917=CARTESIAN_POINT('Ctrl Pts',(0.140128189305237,0.0292221225300861,
-0.451516817063652));
#49918=CARTESIAN_POINT('Ctrl Pts',(0.0527300363818198,0.13307659171636,
-0.444441187607011));
#49919=CARTESIAN_POINT('Ctrl Pts',(-0.0820820875706887,0.117270433800816,
-0.437365558150368));
#49920=CARTESIAN_POINT('Ctrl Pts',(-0.143087260536844,-0.00398350996917575,
-0.430289928693726));
#49921=CARTESIAN_POINT('Ctrl Pts',(-0.0754304482661432,-0.121655572369371,
-0.423214299237084));
#49922=CARTESIAN_POINT('Ctrl Pts',(0.0600522973538647,-0.129936718981696,
-0.416138669780442));
#49923=CARTESIAN_POINT('Ctrl Pts',(0.141536909442611,-0.0213806905643422,
-0.409063040323799));
#49924=CARTESIAN_POINT('Ctrl Pts',(0.0957536130933939,0.106400544593848,
-0.401987410867158));
#49925=CARTESIAN_POINT('Ctrl Pts',(-0.036129919689142,0.138507974702171,
-0.394911781410515));
#49926=CARTESIAN_POINT('Ctrl Pts',(-0.135525961960754,0.0460710752716928,
-0.387836151953873));
#49927=CARTESIAN_POINT('Ctrl Pts',(-0.113059054732024,-0.0877922571708217,
-0.380760522497231));
#49928=CARTESIAN_POINT('Ctrl Pts',(0.0110688890084644,-0.142714084651682,
-0.373684893040588));
#49929=CARTESIAN_POINT('Ctrl Pts',(0.125243850946179,-0.0693095093660329,
-0.366609263583947));
#49930=CARTESIAN_POINT('Ctrl Pts',(0.126801386678129,0.0664171560174392,
-0.359533634127304));
#49931=CARTESIAN_POINT('Ctrl Pts',(0.014340983147462,0.142422492881504,
-0.352458004670663));
#49932=CARTESIAN_POINT('Ctrl Pts',(-0.111014621232627,0.0903636218419115,
-0.34538237521402));
#49933=CARTESIAN_POINT('Ctrl Pts',(-0.136547513264868,-0.0429488870532126,
-0.338306745757379));
#49934=CARTESIAN_POINT('Ctrl Pts',(-0.0392988925141536,-0.13764238927447,
-0.331231116300736));
#49935=CARTESIAN_POINT('Ctrl Pts',(0.0932867135756414,-0.108569882328145,
-0.324155486844094));
#49936=CARTESIAN_POINT('Ctrl Pts',(0.141990280788392,0.0181270637398149,
-0.317079857387452));
#49937=CARTESIAN_POINT('Ctrl Pts',(0.0630182788190301,0.12852442107601,
-0.31000422793081));
#49938=CARTESIAN_POINT('Ctrl Pts',(-0.0726188313010971,0.123354511951355,
-0.302928598474168));
#49939=CARTESIAN_POINT('Ctrl Pts',(-0.14295815788043,0.00726604250490275,
-0.295852969017526));
#49940=CARTESIAN_POINT('Ctrl Pts',(-0.0847516144510158,-0.115355945343988,
-0.288777339560883));
#49941=CARTESIAN_POINT('Ctrl Pts',(0.0496623324298792,-0.134251566158055,
-0.281701710104241));
#49942=CARTESIAN_POINT('Ctrl Pts',(0.139420641440745,-0.0324301560050256,
-0.274626080647599));
#49943=CARTESIAN_POINT('Ctrl Pts',(0.103813963123044,0.0985519727805908,
-0.267550451190957));
#49944=CARTESIAN_POINT('Ctrl Pts',(-0.0251407018124249,0.140917619163273,
-0.260474821734315));
#49945=CARTESIAN_POINT('Ctrl Pts',(-0.131489217962636,0.0565722178974215,
-0.253399192277673));
#49946=CARTESIAN_POINT('Ctrl Pts',(-0.119604565957901,-0.0786420884785688,
-0.246323562821031));
#49947=CARTESIAN_POINT('Ctrl Pts',(-0.000173249838007723,-0.143142587173726,
-0.239247933364388));
#49948=CARTESIAN_POINT('Ctrl Pts',(0.11941384998459,-0.0789313797554197,
-0.232172303907747));
#49949=CARTESIAN_POINT('Ctrl Pts',(0.131625774686089,0.0562537617984851,
-0.225096674451104));
#49950=CARTESIAN_POINT('Ctrl Pts',(0.0254817414384823,0.140856349277387,
-0.218021044994462));
#49951=CARTESIAN_POINT('Ctrl Pts',(-0.103575098403667,0.0988029820840171,
-0.21094541553782));
#49952=CARTESIAN_POINT('Ctrl Pts',(-0.139498735264605,-0.0320925713757056,
-0.203869786081178));
#49953=CARTESIAN_POINT('Ctrl Pts',(-0.0499871639826382,-0.134130957339402,
-0.196794156624536));
#49954=CARTESIAN_POINT('Ctrl Pts',(0.0844721289208749,-0.115560761990362,
-0.189718527167894));
#49955=CARTESIAN_POINT('Ctrl Pts',(0.142975327638465,0.0069199684692118,
-0.182642897711252));
#49956=CARTESIAN_POINT('Ctrl Pts',(0.0729172175665789,0.123178365270598,
-0.175567268254609));
#49957=CARTESIAN_POINT('Ctrl Pts',(-0.0627069806055713,0.128676590121054,
-0.168491638797968));
#49958=CARTESIAN_POINT('Ctrl Pts',(-0.141945985349352,0.0184707205936354,
-0.161416009341325));
#49959=CARTESIAN_POINT('Ctrl Pts',(-0.0935492508051274,-0.108343749316133,
-0.154340379884683));
#49960=CARTESIAN_POINT('Ctrl Pts',(0.0389655923927191,-0.137737114687094,
-0.147264750428041));
#49961=CARTESIAN_POINT('Ctrl Pts',(0.136443148495294,-0.0432792968865944,
-0.140189120971399));
#49962=CARTESIAN_POINT('Ctrl Pts',(0.111233035679392,0.0900946304566556,
-0.133113491514757));
#49963=CARTESIAN_POINT('Ctrl Pts',(-0.0139961856789359,0.142456786934305,
-0.126037862058115));
#49964=CARTESIAN_POINT('Ctrl Pts',(-0.126640240826477,0.0667239103887243,
-0.118962232601472));
#49965=CARTESIAN_POINT('Ctrl Pts',(-0.125411260802437,-0.0690061456941079,
-0.11188660314483));
#49966=CARTESIAN_POINT('Ctrl Pts',(-0.0114143142817069,-0.142686850036267,
-0.104810973688188));
#49967=CARTESIAN_POINT('Ctrl Pts',(0.112846200521126,-0.0880657199346974,
-0.097735344231546));
#49968=CARTESIAN_POINT('Ctrl Pts',(0.135637102362906,0.0457429595208074,
-0.0906597147749039));
#49969=CARTESIAN_POINT('Ctrl Pts',(0.0364650653783499,0.138419956625884,
-0.0835840853182618));
#49970=CARTESIAN_POINT('Ctrl Pts',(-0.0954957185612961,0.106632312231369,
-0.0765084558616196));
#49971=CARTESIAN_POINT('Ctrl Pts',(-0.141588354018362,-0.0210385713465942,
-0.0694328264049776));
#49972=CARTESIAN_POINT('Ctrl Pts',(-0.0603664563464917,-0.129789916779749,
-0.0623571969483353));
#49973=CARTESIAN_POINT('Ctrl Pts',(0.0751353660258105,-0.121839811599314,
-0.0552815674916933));
#49974=CARTESIAN_POINT('Ctrl Pts',(0.143077910335472,-0.00432605712677605,
-0.0482059380350511));
#49975=CARTESIAN_POINT('Ctrl Pts',(0.0823643669338191,0.117064168817031,
-0.041130308578409));
#49976=CARTESIAN_POINT('Ctrl Pts',(-0.0524051812132549,0.13321757339515,
-0.0340546791217669));
#49977=CARTESIAN_POINT('Ctrl Pts',(-0.140061926211041,0.0295351437422096,
-0.0269790496651247));
#49978=CARTESIAN_POINT('Ctrl Pts',(-0.101759571702707,-0.10061243783362,
-0.0199034202084826));
#49979=CARTESIAN_POINT('Ctrl Pts',(0.0280096562024612,-0.140468062943556,
-0.0128277907518404));
#49980=CARTESIAN_POINT('Ctrl Pts',(0.132662650662863,-0.0536652757754266,
-0.00575216129519843));
#49981=CARTESIAN_POINT('Ctrl Pts',(0.122793065054095,0.0358476312668972,
-0.00103507499077024));
#49982=CARTESIAN_POINT('Ctrl Pts',(0.100129091305825,0.068821617783003,
0.0013234681614438));
#49983=CARTESIAN_POINT('Ctrl Pts',(-0.121526217441981,0.000102663445846418,
-0.0254892650149941));
#49984=CARTESIAN_POINT('Ctrl Pts',(-0.121242244193571,-0.0314487625136614,
-0.0236273167461569));
#49985=CARTESIAN_POINT('Ctrl Pts',(-0.10862906823349,-0.0631956500232495,
-0.0217653684773198));
#49986=CARTESIAN_POINT('Ctrl Pts',(-0.0865150928032345,-0.0855637784226379,
-0.0199034202084826));
#49987=CARTESIAN_POINT('Ctrl Pts',(-0.0611643925841885,-0.111205830856965,
-0.017768946805655));
#49988=CARTESIAN_POINT('Ctrl Pts',(-0.0233281783799959,-0.124522749137967,
-0.0156344734028274));
#49989=CARTESIAN_POINT('Ctrl Pts',(0.0125914725202458,-0.12102200839196,
-0.0134999999999998));
#49990=CARTESIAN_POINT('',(-0.0397408188803946,0.087195744963362,-0.5435));
#49991=CARTESIAN_POINT('Ctrl Pts',(-0.0397589391997285,0.0873393895763303,
-0.5435));
#49992=CARTESIAN_POINT('Ctrl Pts',(-0.0371904915887145,0.0889602232112557,
-0.5435));
#49993=CARTESIAN_POINT('Ctrl Pts',(-0.034547455834076,0.0904480486342698,
-0.5435));
#49994=CARTESIAN_POINT('Ctrl Pts',(-0.0318374226014847,0.0917946820255231,
-0.5435));
#49995=CARTESIAN_POINT('Ctrl Pts',(-0.0281424054768352,0.0936307604106386,
-0.5435));
#49996=CARTESIAN_POINT('Ctrl Pts',(-0.0243229557383007,0.0952045898844149,
-0.5435));
#49997=CARTESIAN_POINT('Ctrl Pts',(-0.0204062890282129,0.0965240534970721,
-0.5435));
#49998=CARTESIAN_POINT('Ctrl Pts',(-0.0167937500951651,0.0977410612294859,
-0.5435));
#49999=CARTESIAN_POINT('Ctrl Pts',(-0.0130965167986539,0.0987413727747821,
-0.5435));
#50000=CARTESIAN_POINT('Ctrl Pts',(-0.00935615524967915,0.0995254364772876,
-0.5435));
#50001=CARTESIAN_POINT('Ctrl Pts',(-0.00502742217475035,0.100432836052822,
-0.5435));
#50002=CARTESIAN_POINT('Ctrl Pts',(-0.000635102360800403,0.101053058129917,
-0.5435));
#50003=CARTESIAN_POINT('Ctrl Pts',(0.00378981819427666,0.101393852742248,
-0.5435));
#50004=CARTESIAN_POINT('Ctrl Pts',(0.00811702703254377,0.101727121880114,
-0.5435));
#50005=CARTESIAN_POINT('Ctrl Pts',(0.0124815444740136,0.101792241042985,
-0.5435));
#50006=CARTESIAN_POINT('Ctrl Pts',(0.0168220483608817,0.101595391107322,
-0.5435));
#50007=CARTESIAN_POINT('Ctrl Pts',(0.0249746128899566,0.101225657121392,
-0.5435));
#50008=CARTESIAN_POINT('Ctrl Pts',(0.033059285085718,0.0999386418970613,
-0.5435));
#50009=CARTESIAN_POINT('Ctrl Pts',(0.0408991675195905,0.0977672662931198,
-0.5435));
#50010=CARTESIAN_POINT('Ctrl Pts',(0.0440182920238849,0.0969033769540376,
-0.5435));
#50011=CARTESIAN_POINT('Ctrl Pts',(0.0470988160191229,0.095898938611735,
-0.5435));
#50012=CARTESIAN_POINT('Ctrl Pts',(0.0501296723833096,0.0947537415835819,
-0.5435));
#50013=CARTESIAN_POINT('Ctrl Pts',(0.0526395802787472,0.0938053828633346,
-0.5435));
#50014=CARTESIAN_POINT('Ctrl Pts',(0.0551067701615479,0.0927636927312978,
-0.5435));
#50015=CARTESIAN_POINT('Ctrl Pts',(0.0575242429130301,0.0916305982235789,
-0.5435));
#50016=CARTESIAN_POINT('Ctrl Pts',(0.060635351146661,0.0901723895838809,
-0.5435));
#50017=CARTESIAN_POINT('Ctrl Pts',(0.0636646925010064,0.0885626376171208,
-0.5435));
#50018=CARTESIAN_POINT('Ctrl Pts',(0.0665996639859203,0.0868033222099646,
-0.5435));
#50019=CARTESIAN_POINT('Ctrl Pts',(0.0716119961421378,0.0837987706381539,
-0.5435));
#50020=CARTESIAN_POINT('Ctrl Pts',(0.0763495113381208,0.0803587684725567,
-0.5435));
#50021=CARTESIAN_POINT('Ctrl Pts',(0.0807934344329792,0.0765390108759656,
-0.5435));
#50022=CARTESIAN_POINT('Ctrl Pts',(0.083948765500447,0.0738268577721766,
-0.5435));
#50023=CARTESIAN_POINT('Ctrl Pts',(0.0869599760588301,0.0709177615381115,
-0.5435));
#50024=CARTESIAN_POINT('Ctrl Pts',(0.0897953293542451,0.0678555190520308,
-0.5435));
#50025=CARTESIAN_POINT('Ctrl Pts',(0.0945610893247136,0.0627083958756595,
-0.5435));
#50026=CARTESIAN_POINT('Ctrl Pts',(0.0988428232231053,0.0571219441198984,
-0.5435));
#50027=CARTESIAN_POINT('Ctrl Pts',(0.102610261682682,0.0511883432169625,
-0.5435));
#50028=CARTESIAN_POINT('Ctrl Pts',(0.104979073270572,0.0474575370664183,
-0.5435));
#50029=CARTESIAN_POINT('Ctrl Pts',(0.107144374825992,0.043589008576509,
-0.5435));
#50030=CARTESIAN_POINT('Ctrl Pts',(0.109095735641908,0.0396020278398452,
-0.5435));
#50031=CARTESIAN_POINT('Ctrl Pts',(0.110444498668307,0.0368462626524366,
-0.5435));
#50032=CARTESIAN_POINT('Ctrl Pts',(0.111691464616707,0.0340318757008926,
-0.5435));
#50033=CARTESIAN_POINT('Ctrl Pts',(0.112826566212854,0.031181703065903,
-0.5435));
#50034=CARTESIAN_POINT('Ctrl Pts',(0.11614493200818,0.0228494838048033,
-0.5435));
#50035=CARTESIAN_POINT('Ctrl Pts',(0.118525049958407,0.0141867394355863,
-0.5435));
#50036=CARTESIAN_POINT('Ctrl Pts',(0.119892735971079,0.00535510104883141,
-0.5435));
#50037=CARTESIAN_POINT('Ctrl Pts',(0.120609853674274,0.000724415221322913,
-0.5435));
#50038=CARTESIAN_POINT('Ctrl Pts',(0.12104799608301,-0.00395328391685804,
-0.5435));
#50039=CARTESIAN_POINT('Ctrl Pts',(0.121191192277757,-0.00865707307903657,
-0.5435));
#50040=CARTESIAN_POINT('Ctrl Pts',(-0.0397589391997287,0.0873393895763303,
-0.5435));
#50041=CARTESIAN_POINT('Ctrl Pts',(-0.0655870913757108,0.0753780187149155,
-0.541365526597173));
#50042=CARTESIAN_POINT('Ctrl Pts',(-0.091691234429318,0.0444812340450679,
-0.538636437655985));
#50043=CARTESIAN_POINT('Ctrl Pts',(-0.0958680473392353,0.00803042275043827,
-0.535907348714798));
#50044=CARTESIAN_POINT('Ctrl Pts',(-0.0957990153585407,7.37030635558182E-5,
-0.535312733176438));
#50045=CARTESIAN_POINT('Origin',(-1.13809670924099E-17,0.,-0.5435));
#50046=CARTESIAN_POINT('Ctrl Pts',(0.0681458046084942,-0.100801883029112,
-0.5435));
#50047=CARTESIAN_POINT('Ctrl Pts',(0.0648149048055578,-0.102615870197094,
-0.5435));
#50048=CARTESIAN_POINT('Ctrl Pts',(0.0614014517271168,-0.104260638022271,
-0.5435));
#50049=CARTESIAN_POINT('Ctrl Pts',(0.0579117686900797,-0.10572438322058,
-0.5435));
#50050=CARTESIAN_POINT('Ctrl Pts',(0.0518504450541602,-0.10826680133515,
-0.5435));
#50051=CARTESIAN_POINT('Ctrl Pts',(0.0455589824493805,-0.110263892026136,
-0.5435));
#50052=CARTESIAN_POINT('Ctrl Pts',(0.0391120749818753,-0.111718567430527,
-0.5435));
#50053=CARTESIAN_POINT('Ctrl Pts',(0.0353625795407656,-0.112564600792189,
-0.5435));
#50054=CARTESIAN_POINT('Ctrl Pts',(0.0315690566392495,-0.113224785984647,
-0.5435));
#50055=CARTESIAN_POINT('Ctrl Pts',(0.0277522696084378,-0.11369985104087,
-0.5435));
#50056=CARTESIAN_POINT('Ctrl Pts',(0.0229866093069774,-0.114293019761256,
-0.5435));
#50057=CARTESIAN_POINT('Ctrl Pts',(0.0181817399541562,-0.11459835491698,
-0.5435));
#50058=CARTESIAN_POINT('Ctrl Pts',(0.0133675253247798,-0.11461584389042,
-0.5435));
#50059=CARTESIAN_POINT('Ctrl Pts',(0.00911690029736573,-0.114631285467901,
-0.5435));
#50060=CARTESIAN_POINT('Ctrl Pts',(0.00485415397265722,-0.114421235647892,
-0.5435));
#50061=CARTESIAN_POINT('Ctrl Pts',(0.000630336365389325,-0.113987583954121,
-0.5435));
#50062=CARTESIAN_POINT('Ctrl Pts',(-0.00785120378156423,-0.113116799608654,
-0.5435));
#50063=CARTESIAN_POINT('Ctrl Pts',(-0.0161985641326431,-0.111349438130382,
-0.5435));
#50064=CARTESIAN_POINT('Ctrl Pts',(-0.0242378739522401,-0.108679541554347,
-0.5435));
#50065=CARTESIAN_POINT('Ctrl Pts',(-0.0274386034479911,-0.107616562652764,
-0.5435));
#50066=CARTESIAN_POINT('Ctrl Pts',(-0.0305902132968484,-0.10641002520364,
-0.5435));
#50067=CARTESIAN_POINT('Ctrl Pts',(-0.0336801620372295,-0.105057687860788,
-0.5435));
#50068=CARTESIAN_POINT('Ctrl Pts',(-0.0359790613319563,-0.104051558754799,
-0.5435));
#50069=CARTESIAN_POINT('Ctrl Pts',(-0.0382415656149683,-0.102965465891595,
-0.5435));
#50070=CARTESIAN_POINT('Ctrl Pts',(-0.0404552192737468,-0.101802978363352,
-0.5435));
#50071=CARTESIAN_POINT('Ctrl Pts',(-0.0439854985319678,-0.0999490724496493,
-0.5435));
#50072=CARTESIAN_POINT('Ctrl Pts',(-0.0473975398291214,-0.0978984910598355,
-0.5435));
#50073=CARTESIAN_POINT('Ctrl Pts',(-0.0506719957326547,-0.0956497968821656,
-0.5435));
#50074=CARTESIAN_POINT('Ctrl Pts',(-0.054946246470959,-0.0927145053307493,
-0.5435));
#50075=CARTESIAN_POINT('Ctrl Pts',(-0.0589863515765622,-0.0894416590788099,
-0.5435));
#50076=CARTESIAN_POINT('Ctrl Pts',(-0.0627693636876284,-0.0858685577421909,
-0.5435));
#50077=CARTESIAN_POINT('Ctrl Pts',(-0.0648837750791162,-0.0838714702501929,
-0.5435));
#50078=CARTESIAN_POINT('Ctrl Pts',(-0.0669188095625019,-0.0817793079138408,
-0.5435));
#50079=CARTESIAN_POINT('Ctrl Pts',(-0.0688660649399109,-0.0796019918163136,
-0.5435));
#50080=CARTESIAN_POINT('Ctrl Pts',(-0.0742047958657111,-0.0736325104016171,
-0.5435));
#50081=CARTESIAN_POINT('Ctrl Pts',(-0.0788451394315893,-0.0670732251057521,
-0.5435));
#50082=CARTESIAN_POINT('Ctrl Pts',(-0.0827070282539586,-0.0600679424715311,
-0.5435));
#50083=CARTESIAN_POINT('Ctrl Pts',(-0.0845348325968156,-0.0567523923325412,
-0.5435));
#50084=CARTESIAN_POINT('Ctrl Pts',(-0.0861875716311489,-0.0533366354792091,
-0.5435));
#50085=CARTESIAN_POINT('Ctrl Pts',(-0.0876527120283092,-0.0498353171887534,
-0.5435));
#50086=CARTESIAN_POINT('Ctrl Pts',(-0.0888770503705417,-0.0469094554490365,
-0.5435));
#50087=CARTESIAN_POINT('Ctrl Pts',(-0.0899703462593087,-0.0439221864599506,
-0.5435));
#50088=CARTESIAN_POINT('Ctrl Pts',(-0.0909189876323078,-0.040902363707549,
-0.5435));
#50089=CARTESIAN_POINT('Ctrl Pts',(-0.0931572896503075,-0.0337771469996449,
-0.5435));
#50090=CARTESIAN_POINT('Ctrl Pts',(-0.0946051988332896,-0.026445709106482,
-0.5435));
#50091=CARTESIAN_POINT('Ctrl Pts',(-0.0951682868431173,-0.0190266560863368,
-0.5435));
#50092=CARTESIAN_POINT('Ctrl Pts',(-0.0954163614839278,-0.0157581103510265,
-0.5435));
#50093=CARTESIAN_POINT('Ctrl Pts',(-0.0954920586844475,-0.0124726380609223,
-0.5435));
#50094=CARTESIAN_POINT('Ctrl Pts',(-0.0953841396803774,-0.00918131376406761,
-0.5435));
#50095=CARTESIAN_POINT('Origin',(0.,0.,-0.5435));
#50096=CARTESIAN_POINT('Origin',(0.,0.,-0.656687266823562));
#50097=CARTESIAN_POINT('Ctrl Pts',(-0.120941017178877,-0.0116413213914294,
-0.558323468161444));
#50098=CARTESIAN_POINT('Ctrl Pts',(-0.11710735835321,-0.0514689820412212,
-0.55596492500923));
#50099=CARTESIAN_POINT('Ctrl Pts',(-0.0671300264001348,-0.126383894366809,
-0.551247838704802));
#50100=CARTESIAN_POINT('Ctrl Pts',(0.0688344370813445,-0.125609043089213,
-0.544172209248159));
#50101=CARTESIAN_POINT('Ctrl Pts',(0.142624820499317,-0.0116638107424766,
-0.537096579791518));
#50102=CARTESIAN_POINT('Ctrl Pts',(0.0883088191683241,0.112655311145294,
-0.530020950334875));
#50103=CARTESIAN_POINT('Ctrl Pts',(-0.0454858975362832,0.135735984585036,
-0.522945320878234));
#50104=CARTESIAN_POINT('Ctrl Pts',(-0.138342174559802,0.0367335649717563,
-0.51586969142159));
#50105=CARTESIAN_POINT('Ctrl Pts',(-0.10682330188696,-0.0952826647968933,
-0.50879406196495));
#50106=CARTESIAN_POINT('Ctrl Pts',(0.0207600900262283,-0.141630796899509,
-0.501718432508306));
#50107=CARTESIAN_POINT('Ctrl Pts',(0.129670744621718,-0.0606220370298399,
-0.494642803051665));
#50108=CARTESIAN_POINT('Ctrl Pts',(0.121986308252591,0.0748947619158391,
-0.487567173595023));
#50109=CARTESIAN_POINT('Ctrl Pts',(0.00461203604021712,0.143068559645755,
-0.48049154413838));
#50110=CARTESIAN_POINT('Ctrl Pts',(-0.116908498038604,0.0825965493599512,
-0.473415914681739));
#50111=CARTESIAN_POINT('Ctrl Pts',(-0.133307060630641,-0.052144710735923,
-0.466340285225096));
#50112=CARTESIAN_POINT('Ctrl Pts',(-0.0298376523318702,-0.139998399680144,
-0.459264655768454));
#50113=CARTESIAN_POINT('Ctrl Pts',(0.100461214812515,-0.101967492333341,
-0.452189026311812));
#50114=CARTESIAN_POINT('Ctrl Pts',(0.140426899719575,0.0277510310822455,
-0.445113396855169));
#50115=CARTESIAN_POINT('Ctrl Pts',(0.0541227517773754,0.132516263042559,
-0.438037767398528));
#50116=CARTESIAN_POINT('Ctrl Pts',(-0.0808477600960478,0.118124808842324,
-0.430962137941885));
#50117=CARTESIAN_POINT('Ctrl Pts',(-0.143121165975879,-0.00248272619463574,
-0.423886508485243));
#50118=CARTESIAN_POINT('Ctrl Pts',(-0.0767021225665899,-0.120857834339742,
-0.416810879028602));
#50119=CARTESIAN_POINT('Ctrl Pts',(0.0586863372203009,-0.130559355827306,
-0.409735249571959));
#50120=CARTESIAN_POINT('Ctrl Pts',(0.141304908270695,-0.0228638285875853,
-0.402659620115317));
#50121=CARTESIAN_POINT('Ctrl Pts',(0.0968641863105561,0.105390517142955,
-0.395583990658675));
#50122=CARTESIAN_POINT('Ctrl Pts',(-0.0346753849482346,0.138879261798831,
-0.388508361202033));
#50123=CARTESIAN_POINT('Ctrl Pts',(-0.135035360971776,0.047489819885674,
-0.38143273174539));
#50124=CARTESIAN_POINT('Ctrl Pts',(-0.113973529173592,-0.0866017686993902,
-0.374357102288749));
#50125=CARTESIAN_POINT('Ctrl Pts',(0.00957162134612276,-0.142822322338734,
-0.367281472832107));
#50126=CARTESIAN_POINT('Ctrl Pts',(0.124510110955252,-0.0706191473108742,
-0.360205843375464));
#50127=CARTESIAN_POINT('Ctrl Pts',(0.127490942623884,0.0650837248780568,
-0.353130213918822));
#50128=CARTESIAN_POINT('Ctrl Pts',(0.0158337964415146,0.142264270234911,
-0.34605458446218));
#50129=CARTESIAN_POINT('Ctrl Pts',(-0.110060866297358,0.0915228791372047,
-0.338978955005538));
#50130=CARTESIAN_POINT('Ctrl Pts',(-0.13699041908937,-0.0415145368890392,
-0.331903325548895));
#50131=CARTESIAN_POINT('Ctrl Pts',(-0.0407402046988056,-0.137222692789984,
-0.324827696092254));
#50132=CARTESIAN_POINT('Ctrl Pts',(0.0921430017160038,-0.109542224417149,
-0.317752066635611));
#50133=CARTESIAN_POINT('Ctrl Pts',(0.142172578114354,0.0166369987607558,
-0.31067643717897));
#50134=CARTESIAN_POINT('Ctrl Pts',(0.0643626662592367,0.127856477690649,
-0.303600807722327));
#50135=CARTESIAN_POINT('Ctrl Pts',(-0.0713212071316596,0.124109295013498,
-0.296525178265685));
#50136=CARTESIAN_POINT('Ctrl Pts',(-0.142874101523106,0.0087648622021492,
-0.289449548809043));
#50137=CARTESIAN_POINT('Ctrl Pts',(-0.08595670814417,-0.114460805608188,
-0.282373919352401));
#50138=CARTESIAN_POINT('Ctrl Pts',(0.0482516911858636,-0.134765002850031,
-0.275298289895759));
#50139=CARTESIAN_POINT('Ctrl Pts',(0.13907288047591,-0.0338904944134862,
-0.268222660439116));
#50140=CARTESIAN_POINT('Ctrl Pts',(0.10484178397496,0.0974578474438835,
-0.261147030982475));
#50141=CARTESIAN_POINT('Ctrl Pts',(-0.0236615005155487,0.14117352828645,
-0.254071401525832));
#50142=CARTESIAN_POINT('Ctrl Pts',(-0.130888712240556,0.0579480517657311,
-0.24699577206919));
#50143=CARTESIAN_POINT('Ctrl Pts',(-0.120422721711377,-0.0773834594148965,
-0.239920142612548));
#50144=CARTESIAN_POINT('Ctrl Pts',(-0.00167439346369711,-0.143132903632313,
-0.232844513155906));
#50145=CARTESIAN_POINT('Ctrl Pts',(0.118579524725311,-0.0801793490316698,
-0.225768883699263));
#50146=CARTESIAN_POINT('Ctrl Pts',(0.132208480778061,0.0548702952924991,
-0.218693254242622));
#50147=CARTESIAN_POINT('Ctrl Pts',(0.0269575181460965,0.140581378256179,
-0.211617624785979));
#50148=CARTESIAN_POINT('Ctrl Pts',(-0.102533247759778,0.0998837564234286,
-0.204541995329338));
#50149=CARTESIAN_POINT('Ctrl Pts',(-0.139827627438852,-0.0306278680121232,
-0.197466365872695));
#50150=CARTESIAN_POINT('Ctrl Pts',(-0.051391063975439,-0.133599364702921,
-0.190390736416053));
#50151=CARTESIAN_POINT('Ctrl Pts',(0.0832555873046201,-0.116440280236949,
-0.183315106959411));
#50152=CARTESIAN_POINT('Ctrl Pts',(0.143040040704376,0.00542018897790831,
-0.176239477502769));
#50153=CARTESIAN_POINT('Ctrl Pts',(0.0742049962749289,0.122406904572045,
-0.169163848046126));
#50154=CARTESIAN_POINT('Ctrl Pts',(-0.0613540878947369,0.129327133537324,
-0.162088218589485));
#50155=CARTESIAN_POINT('Ctrl Pts',(-0.141744479849913,0.0199583105394808,
-0.155012589132842));
#50156=CARTESIAN_POINT('Ctrl Pts',(-0.0946803232670462,-0.107356734608036,
-0.1479369596762));
#50157=CARTESIAN_POINT('Ctrl Pts',(0.0375189856164575,-0.138138178990805,
-0.140861330219558));
#50158=CARTESIAN_POINT('Ctrl Pts',(0.135981775009837,-0.0447078191806976,
-0.133785700762916));
#50159=CARTESIAN_POINT('Ctrl Pts',(0.112171755540986,0.0889231755496423,
-0.126710071306274));
#50160=CARTESIAN_POINT('Ctrl Pts',(-0.0125014551897662,0.14259571800196,
-0.119634441849632));
#50161=CARTESIAN_POINT('Ctrl Pts',(-0.125933540022816,0.068048371817411,
-0.11255881239299));
#50162=CARTESIAN_POINT('Ctrl Pts',(-0.126128043361885,-0.0676872214632633,
-0.105483182936348));
#50163=CARTESIAN_POINT('Ctrl Pts',(-0.0129100623071776,-0.142559170771431,
-0.0984075534797053));
#50164=CARTESIAN_POINT('Ctrl Pts',(0.111916446224502,-0.0892445667815422,
-0.0913319240230634));
#50165=CARTESIAN_POINT('Ctrl Pts',(0.136109354430927,0.0443184882404931,
-0.0842562945664211));
#50166=CARTESIAN_POINT('Ctrl Pts',(0.037914698287885,0.138029015203821,
-0.077180665109779));
#50167=CARTESIAN_POINT('Ctrl Pts',(-0.0943722248490409,0.107629675951055,
-0.070105035653137));
#50168=CARTESIAN_POINT('Ctrl Pts',(-0.141801168750683,-0.0195558834566498,
-0.0630294061964947));
#50169=CARTESIAN_POINT('Ctrl Pts',(-0.0617243330219531,-0.129143403898395,
-0.0559537767398526));
#50170=CARTESIAN_POINT('Ctrl Pts',(0.0738536247947097,-0.122633056272086,
-0.0488781472832105));
#50171=CARTESIAN_POINT('Ctrl Pts',(0.143024424514937,-0.00580350448589463,
-0.0418025178265684));
#50172=CARTESIAN_POINT('Ctrl Pts',(0.0835879551182714,0.116150495748595,
-0.0347268883699262));
#50173=CARTESIAN_POINT('Ctrl Pts',(-0.0510057890185001,0.133844017127003,
-0.0276512589132841));
#50174=CARTESIAN_POINT('Ctrl Pts',(-0.139745887278106,0.0308288207471279,
-0.020575629456642));
#50175=CARTESIAN_POINT('Ctrl Pts',(-0.115110781316278,-0.0557915541778742,
-0.0158585431522139));
#50176=CARTESIAN_POINT('Ctrl Pts',(-0.0872731800879813,-0.0845318995251544,
-0.0134999999999998));
#50177=CARTESIAN_POINT('Ctrl Pts',(-0.112422058012711,-0.0108213188489747,
-0.553382312107629));
#50178=CARTESIAN_POINT('Ctrl Pts',(-0.108858438118042,-0.0478435606038874,
-0.551023768955415));
#50179=CARTESIAN_POINT('Ctrl Pts',(-0.0624014573251726,-0.117481544605856,
-0.546306682650987));
#50180=CARTESIAN_POINT('Ctrl Pts',(0.0639858110948882,-0.116761273044451,
-0.539231053194346));
#50181=CARTESIAN_POINT('Ctrl Pts',(0.132578476833144,-0.0108422240735788,
-0.532155423737702));
#50182=CARTESIAN_POINT('Ctrl Pts',(0.0820884380101708,0.104719988474086,
-0.525079794281062));
#50183=CARTESIAN_POINT('Ctrl Pts',(-0.0422819183339681,0.126174883338888,
-0.518004164824418));
#50184=CARTESIAN_POINT('Ctrl Pts',(-0.128597496008848,0.0341460909507685,
-0.510928535367777));
#50185=CARTESIAN_POINT('Ctrl Pts',(-0.0992987798678985,-0.0885710532230661,
-0.503852905911134));
#50186=CARTESIAN_POINT('Ctrl Pts',(0.0192977709276737,-0.131654471219413,
-0.496777276454492));
#50187=CARTESIAN_POINT('Ctrl Pts',(0.120536872555428,-0.0563518839413863,
-0.48970164699785));
#50188=CARTESIAN_POINT('Ctrl Pts',(0.113393719872933,0.0696192529660752,
-0.482626017541208));
#50189=CARTESIAN_POINT('Ctrl Pts',(0.0042871690297017,0.132990959456715,
-0.475550388084567));
#50190=CARTESIAN_POINT('Ctrl Pts',(-0.108673585316681,0.0767785345319212,
-0.468474758627923));
#50191=CARTESIAN_POINT('Ctrl Pts',(-0.123917050255629,-0.0484716916737979,
-0.461399129171282));
#50192=CARTESIAN_POINT('Ctrl Pts',(-0.0277359192080814,-0.130137058358367,
-0.454323499714639));
#50193=CARTESIAN_POINT('Ctrl Pts',(0.09338483157435,-0.0947850084769385,
-0.447247870257998));
#50194=CARTESIAN_POINT('Ctrl Pts',(0.130535375301742,0.0257962773839288,
-0.440172240801355));
#50195=CARTESIAN_POINT('Ctrl Pts',(0.0503104015664444,0.123181955625226,
-0.433096611344713));
#50196=CARTESIAN_POINT('Ctrl Pts',(-0.0751529281606134,0.109804220455419,
-0.426020981888071));
#50197=CARTESIAN_POINT('Ctrl Pts',(-0.133039860251789,-0.00230784554978795,
-0.418945352431429));
#50198=CARTESIAN_POINT('Ctrl Pts',(-0.0712993050168028,-0.112344734486044,
-0.411869722974787));
#50199=CARTESIAN_POINT('Ctrl Pts',(0.0545525328084189,-0.121362890914093,
-0.404794093518144));
#50200=CARTESIAN_POINT('Ctrl Pts',(0.131351537845866,-0.0212533243379652,
-0.397718464061502));
#50201=CARTESIAN_POINT('Ctrl Pts',(0.0900411740100795,0.09796691898755,
-0.39064283460486));
#50202=CARTESIAN_POINT('Ctrl Pts',(-0.0322328869824028,0.129096751382686,
-0.383567205148218));
#50203=CARTESIAN_POINT('Ctrl Pts',(-0.12552361092253,0.0441446864822037,
-0.376491575691576));
#50204=CARTESIAN_POINT('Ctrl Pts',(-0.105945352598744,-0.0805016303966285,
-0.369415946234934));
#50205=CARTESIAN_POINT('Ctrl Pts',(0.00889740631714755,-0.132762066848893,
-0.362340316778292));
#50206=CARTESIAN_POINT('Ctrl Pts',(0.115739748544344,-0.065644808196452,
-0.355264687321649));
#50207=CARTESIAN_POINT('Ctrl Pts',(0.118510613537825,0.0604992951489926,
-0.348189057865007));
#50208=CARTESIAN_POINT('Ctrl Pts',(0.0147184803272866,0.13224332335348,
-0.341113428408366));
#50209=CARTESIAN_POINT('Ctrl Pts',(-0.102308293616468,0.0850761029455781,
-0.334037798951723));
#50210=CARTESIAN_POINT('Ctrl Pts',(-0.127340956784515,-0.0385902961904772,
-0.326962169495081));
#50211=CARTESIAN_POINT('Ctrl Pts',(-0.0378705071524625,-0.127556869367809,
-0.319886540038439));
#50212=CARTESIAN_POINT('Ctrl Pts',(0.0856525447364202,-0.101826184329603,
-0.312810910581796));
#50213=CARTESIAN_POINT('Ctrl Pts',(0.132158089930304,0.0154651059125196,
-0.305735281125155));
#50214=CARTESIAN_POINT('Ctrl Pts',(0.0598290271475602,0.118850400695567,
-0.298659651668512));
#50215=CARTESIAN_POINT('Ctrl Pts',(-0.0662974156553768,0.115367165659667,
-0.291584022211871));
#50216=CARTESIAN_POINT('Ctrl Pts',(-0.132810198761499,0.0081474744462084,
-0.284508392755229));
#50217=CARTESIAN_POINT('Ctrl Pts',(-0.0799020072344259,-0.106398305789285,
-0.277432763298586));
#50218=CARTESIAN_POINT('Ctrl Pts',(0.0448528923622785,-0.125272296545025,
-0.270357133841945));
#50219=CARTESIAN_POINT('Ctrl Pts',(0.129276731762003,-0.0315032833186536,
-0.263281504385301));
#50220=CARTESIAN_POINT('Ctrl Pts',(0.0974568380118396,0.0905930182720822,
-0.256205874928661));
#50221=CARTESIAN_POINT('Ctrl Pts',(-0.0219948090869163,0.131229412130745,
-0.249130245472017));
#50222=CARTESIAN_POINT('Ctrl Pts',(-0.121669047804956,0.0538662514115874,
-0.242054616015376));
#50223=CARTESIAN_POINT('Ctrl Pts',(-0.111940270737605,-0.0719326492078258,
-0.234978986558733));
#50224=CARTESIAN_POINT('Ctrl Pts',(-0.00155645093370914,-0.133050771119941,
-0.227903357102092));
#50225=CARTESIAN_POINT('Ctrl Pts',(0.110226906625662,-0.0745315992747744,
-0.220827727645449));
#50226=CARTESIAN_POINT('Ctrl Pts',(0.122895853222569,0.051005288895696,
-0.213752098188807));
#50227=CARTESIAN_POINT('Ctrl Pts',(0.0250586586717446,0.130678972531276,
-0.206676468732165));
#50228=CARTESIAN_POINT('Ctrl Pts',(-0.0953109126809523,0.0928480487521756,
-0.199600839275523));
#50229=CARTESIAN_POINT('Ctrl Pts',(-0.129978315135717,-0.0284704729196375,
-0.192525209818881));
#50230=CARTESIAN_POINT('Ctrl Pts',(-0.0477711310054264,-0.124188764733792,
-0.185449580362238));
#50231=CARTESIAN_POINT('Ctrl Pts',(0.0773911505308316,-0.108238348288846,
-0.178373950905597));
#50232=CARTESIAN_POINT('Ctrl Pts',(0.132964449359835,0.0050383965169822,
-0.171298321448954));
#50233=CARTESIAN_POINT('Ctrl Pts',(0.0689780736978123,0.113784689826127,
-0.164222691992312));
#50234=CARTESIAN_POINT('Ctrl Pts',(-0.0570323699065417,0.120217465077596,
-0.15714706253567));
#50235=CARTESIAN_POINT('Ctrl Pts',(-0.131760146461308,0.018552467952097,
-0.150071433079028));
#50236=CARTESIAN_POINT('Ctrl Pts',(-0.0880111400026247,-0.0997946381442195,
-0.142995803622385));
#50237=CARTESIAN_POINT('Ctrl Pts',(0.0348761873840781,-0.12840786967506,
-0.135920174165744));
#50238=CARTESIAN_POINT('Ctrl Pts',(0.126403360542409,-0.0415586470065835,
-0.128844544709101));
#50239=CARTESIAN_POINT('Ctrl Pts',(0.104270494022426,0.0826595197684713,
-0.121768915252459));
#50240=CARTESIAN_POINT('Ctrl Pts',(-0.0116208657192668,0.132551424285361,
-0.114693285795817));
#50241=CARTESIAN_POINT('Ctrl Pts',(-0.117062912752348,0.0632551154486533,
-0.107617656339175));
#50242=CARTESIAN_POINT('Ctrl Pts',(-0.117243715478986,-0.062919404148945,
-0.100542026882533));
#50243=CARTESIAN_POINT('Ctrl Pts',(-0.0120006909773092,-0.132517451403649,
-0.0934663974258908));
#50244=CARTESIAN_POINT('Ctrl Pts',(0.104033168428031,-0.0829582725370532,
-0.0863907679692488));
#50245=CARTESIAN_POINT('Ctrl Pts',(0.126521953402081,0.0411967401319214,
-0.0793151385126065));
#50246=CARTESIAN_POINT('Ctrl Pts',(0.0352440264674689,0.128306395271426,
-0.0722395090559646));
#50247=CARTESIAN_POINT('Ctrl Pts',(-0.087724743715985,0.100048353783583,
-0.0651638795993223));
#50248=CARTESIAN_POINT('Ctrl Pts',(-0.131812842255007,-0.018178387413442,
-0.0580882501426802));
#50249=CARTESIAN_POINT('Ctrl Pts',(-0.0573765353529852,-0.120046677162891,
-0.0510126206860381));
#50250=CARTESIAN_POINT('Ctrl Pts',(0.0686514524583478,-0.113994911636185,
-0.0439369912293959));
#50251=CARTESIAN_POINT('Ctrl Pts',(0.132949933158501,-0.0053947116802003,
-0.0368613617727538));
#50252=CARTESIAN_POINT('Ctrl Pts',(0.0777001067021897,0.107968975917745,
-0.0297857323161117));
#50253=CARTESIAN_POINT('Ctrl Pts',(-0.0474129944147971,0.124416184096178,
-0.0227101028594696));
#50254=CARTESIAN_POINT('Ctrl Pts',(-0.129902332666679,0.0286572707534853,
-0.0156344734028275));
#50255=CARTESIAN_POINT('Ctrl Pts',(-0.107002497886112,-0.0518616552656198,
-0.0109173870983993));
#50256=CARTESIAN_POINT('Ctrl Pts',(-0.0811257482669688,-0.0785775606491374,
-0.0085588439461853));
#50257=CARTESIAN_POINT('Ctrl Pts',(-0.103903098846544,-0.01000131630652,
-0.548441156053815));
#50258=CARTESIAN_POINT('Ctrl Pts',(-0.100609517882874,-0.0442181391665536,
-0.546082612901601));
#50259=CARTESIAN_POINT('Ctrl Pts',(-0.0576728882502106,-0.108579194844902,
-0.541365526597172));
#50260=CARTESIAN_POINT('Ctrl Pts',(0.059137185108432,-0.107913502999689,
-0.534289897140531));
#50261=CARTESIAN_POINT('Ctrl Pts',(0.122532133166971,-0.0100206374046807,
-0.527214267683888));
#50262=CARTESIAN_POINT('Ctrl Pts',(0.0758680568520174,0.096784665802878,
-0.520138638227247));
#50263=CARTESIAN_POINT('Ctrl Pts',(-0.0390779391316531,0.11661378209274,
-0.513063008770604));
#50264=CARTESIAN_POINT('Ctrl Pts',(-0.118852817457893,0.0315586169297806,
-0.505987379313962));
#50265=CARTESIAN_POINT('Ctrl Pts',(-0.0917742578488372,-0.0818594416492388,
-0.49891174985732));
#50266=CARTESIAN_POINT('Ctrl Pts',(0.017835451829119,-0.121678145539317,
-0.491836120400678));
#50267=CARTESIAN_POINT('Ctrl Pts',(0.111403000489139,-0.0520817308529327,
-0.484760490944035));
#50268=CARTESIAN_POINT('Ctrl Pts',(0.104801131493274,0.0643437440163113,
-0.477684861487394));
#50269=CARTESIAN_POINT('Ctrl Pts',(0.00396230201918651,0.122913359267676,
-0.470609232030751));
#50270=CARTESIAN_POINT('Ctrl Pts',(-0.100438672594758,0.0709605197038912,
-0.46353360257411));
#50271=CARTESIAN_POINT('Ctrl Pts',(-0.114527039880617,-0.0447986726116728,
-0.456457973117467));
#50272=CARTESIAN_POINT('Ctrl Pts',(-0.0256341860842926,-0.12027571703659,
-0.449382343660825));
#50273=CARTESIAN_POINT('Ctrl Pts',(0.086308448336185,-0.0876025246205361,
-0.442306714204183));
#50274=CARTESIAN_POINT('Ctrl Pts',(0.120643850883909,0.0238415236856122,
-0.435231084747541));
#50275=CARTESIAN_POINT('Ctrl Pts',(0.0464980513555134,0.113847648207894,
-0.428155455290898));
#50276=CARTESIAN_POINT('Ctrl Pts',(-0.0694580962251789,0.101483632068514,
-0.421079825834256));
#50277=CARTESIAN_POINT('Ctrl Pts',(-0.1229585545277,-0.00213296490494009,
-0.414004196377614));
#50278=CARTESIAN_POINT('Ctrl Pts',(-0.0658964874670156,-0.103831634632347,
-0.406928566920973));
#50279=CARTESIAN_POINT('Ctrl Pts',(0.0504187283965367,-0.112166426000879,
-0.39985293746433));
#50280=CARTESIAN_POINT('Ctrl Pts',(0.121398167421037,-0.0196428200883453,
-0.392777308007688));
#50281=CARTESIAN_POINT('Ctrl Pts',(0.0832181617096029,0.090543320832145,
-0.385701678551046));
#50282=CARTESIAN_POINT('Ctrl Pts',(-0.0297903890165711,0.11931424096654,
-0.378626049094403));
#50283=CARTESIAN_POINT('Ctrl Pts',(-0.116011860873284,0.0407995530787335,
-0.371550419637762));
#50284=CARTESIAN_POINT('Ctrl Pts',(-0.097917176023896,-0.0744014920938668,
-0.364474790181119));
#50285=CARTESIAN_POINT('Ctrl Pts',(0.00822319128817242,-0.122701811359053,
-0.357399160724477));
#50286=CARTESIAN_POINT('Ctrl Pts',(0.106969386133436,-0.0606704690820297,
-0.350323531267835));
#50287=CARTESIAN_POINT('Ctrl Pts',(0.109530284451767,0.0559148654199285,
-0.343247901811193));
#50288=CARTESIAN_POINT('Ctrl Pts',(0.0136031642130584,0.12222237647205,
-0.336172272354551));
#50289=CARTESIAN_POINT('Ctrl Pts',(-0.0945557209355774,0.0786293267539514,
-0.329096642897909));
#50290=CARTESIAN_POINT('Ctrl Pts',(-0.11769149447966,-0.0356660554919151,
-0.322021013441267));
#50291=CARTESIAN_POINT('Ctrl Pts',(-0.0350008096061194,-0.117891045945634,
-0.314945383984624));
#50292=CARTESIAN_POINT('Ctrl Pts',(0.0791620877568367,-0.0941101442420569,
-0.307869754527982));
#50293=CARTESIAN_POINT('Ctrl Pts',(0.122143601746255,0.0142932130642829,
-0.30079412507134));
#50294=CARTESIAN_POINT('Ctrl Pts',(0.0552953880358837,0.109844323700485,
-0.293718495614698));
#50295=CARTESIAN_POINT('Ctrl Pts',(-0.0612736241790938,0.106625036305835,
-0.286642866158056));
#50296=CARTESIAN_POINT('Ctrl Pts',(-0.122746295999892,0.00753008669026765,
-0.279567236701414));
#50297=CARTESIAN_POINT('Ctrl Pts',(-0.0738473063246818,-0.0983358059703825,
-0.272491607244772));
#50298=CARTESIAN_POINT('Ctrl Pts',(0.0414540935386933,-0.115779590240019,
-0.26541597778813));
#50299=CARTESIAN_POINT('Ctrl Pts',(0.119480583048096,-0.0291160722238209,
-0.258340348331487));
#50300=CARTESIAN_POINT('Ctrl Pts',(0.0900718920487197,0.083728189100281,
-0.251264718874845));
#50301=CARTESIAN_POINT('Ctrl Pts',(-0.0203281176582841,0.121285295975039,
-0.244189089418203));
#50302=CARTESIAN_POINT('Ctrl Pts',(-0.112449383369356,0.0497844510574437,
-0.237113459961561));
#50303=CARTESIAN_POINT('Ctrl Pts',(-0.103457819763834,-0.0664818390007551,
-0.230037830504919));
#50304=CARTESIAN_POINT('Ctrl Pts',(-0.001438508403721,-0.122968638607569,
-0.222962201048277));
#50305=CARTESIAN_POINT('Ctrl Pts',(0.101874288526012,-0.0688838495178792,
-0.215886571591635));
#50306=CARTESIAN_POINT('Ctrl Pts',(0.113583225667077,0.0471402824988931,
-0.208810942134992));
#50307=CARTESIAN_POINT('Ctrl Pts',(0.0231597991973928,0.120776566806372,
-0.20173531267835));
#50308=CARTESIAN_POINT('Ctrl Pts',(-0.0880885776021261,0.0858123410809228,
-0.194659683221708));
#50309=CARTESIAN_POINT('Ctrl Pts',(-0.120129002832582,-0.0263130778271519,
-0.187584053765066));
#50310=CARTESIAN_POINT('Ctrl Pts',(-0.0441511980354138,-0.114778164764663,
-0.180508424308424));
#50311=CARTESIAN_POINT('Ctrl Pts',(0.0715267137570432,-0.100036416340742,
-0.173432794851782));
#50312=CARTESIAN_POINT('Ctrl Pts',(0.122888858015295,0.00465660405605617,
-0.16635716539514));
#50313=CARTESIAN_POINT('Ctrl Pts',(0.0637511511206958,0.105162475080209,
-0.159281535938498));
#50314=CARTESIAN_POINT('Ctrl Pts',(-0.0527106519183466,0.111107796617868,
-0.152205906481856));
#50315=CARTESIAN_POINT('Ctrl Pts',(-0.121775813072703,0.0171466253647131,
-0.145130277025213));
#50316=CARTESIAN_POINT('Ctrl Pts',(-0.0813419567382034,-0.0922325416804027,
-0.138054647568571));
#50317=CARTESIAN_POINT('Ctrl Pts',(0.0322333891516986,-0.118677560359315,
-0.130979018111929));
#50318=CARTESIAN_POINT('Ctrl Pts',(0.116824946074981,-0.0384094748324691,
-0.123903388655287));
#50319=CARTESIAN_POINT('Ctrl Pts',(0.0963692325038669,0.0763958639873,-0.116827759198645));
#50320=CARTESIAN_POINT('Ctrl Pts',(-0.0107402762487675,0.122507130568762,
-0.109752129742003));
#50321=CARTESIAN_POINT('Ctrl Pts',(-0.10819228548188,0.0584618590798953,
-0.10267650028536));
#50322=CARTESIAN_POINT('Ctrl Pts',(-0.108359387596088,-0.0581515868346264,
-0.0956008708287185));
#50323=CARTESIAN_POINT('Ctrl Pts',(-0.0110913196474408,-0.122475732035867,
-0.0885252413720763));
#50324=CARTESIAN_POINT('Ctrl Pts',(0.0961498906315588,-0.0766719782925641,
-0.0814496119154342));
#50325=CARTESIAN_POINT('Ctrl Pts',(0.116934552373236,0.0380749920233496,
-0.0743739824587921));
#50326=CARTESIAN_POINT('Ctrl Pts',(0.0325733546470527,0.118583775339031,
-0.06729835300215));
#50327=CARTESIAN_POINT('Ctrl Pts',(-0.0810772625829288,0.092467031616111,
-0.0602227235455078));
#50328=CARTESIAN_POINT('Ctrl Pts',(-0.121824515759332,-0.0168008913702342,
-0.0531470940888656));
#50329=CARTESIAN_POINT('Ctrl Pts',(-0.053028737684017,-0.110949950427387,
-0.0460714646322235));
#50330=CARTESIAN_POINT('Ctrl Pts',(0.0634492801219856,-0.105356767000284,
-0.0389958351755814));
#50331=CARTESIAN_POINT('Ctrl Pts',(0.122875441802065,-0.00498591887450599,
-0.0319202057189393));
#50332=CARTESIAN_POINT('Ctrl Pts',(0.0718122582861078,0.099787456086894,
-0.0248445762622972));
#50333=CARTESIAN_POINT('Ctrl Pts',(-0.043820199811094,0.114988351065352,
-0.017768946805655));
#50334=CARTESIAN_POINT('Ctrl Pts',(-0.120058778055251,0.0264857207598426,
-0.010693317349013));
#50335=CARTESIAN_POINT('Ctrl Pts',(-0.0988942144559457,-0.0479317563533654,
-0.00597623104458479));
#50336=CARTESIAN_POINT('Ctrl Pts',(-0.0749783164459562,-0.0726232217731204,
-0.00361768789237075));
#50337=CARTESIAN_POINT('Ctrl Pts',(-0.0953841396803776,-0.00918131376406524,
-0.5435));
#50338=CARTESIAN_POINT('Ctrl Pts',(-0.0923605976477055,-0.0405927177292199,
-0.541141456847786));
#50339=CARTESIAN_POINT('Ctrl Pts',(-0.0529443191752485,-0.0996768450839476,
-0.536424370543358));
#50340=CARTESIAN_POINT('Ctrl Pts',(0.0542885591219757,-0.0990657329549278,
-0.529348741086716));
#50341=CARTESIAN_POINT('Ctrl Pts',(0.112485789500799,-0.00919905073578263,
-0.522273111630074));
#50342=CARTESIAN_POINT('Ctrl Pts',(0.0696476756938639,0.0888493431316701,
-0.515197482173432));
#50343=CARTESIAN_POINT('Ctrl Pts',(-0.0358739599293379,0.107052680846593,
-0.508121852716789));
#50344=CARTESIAN_POINT('Ctrl Pts',(-0.109108138906939,0.0289711429087928,
-0.501046223260148));
#50345=CARTESIAN_POINT('Ctrl Pts',(-0.0842497358297758,-0.0751478300754116,
-0.493970593803505));
#50346=CARTESIAN_POINT('Ctrl Pts',(0.0163731327305643,-0.111701819859221,
-0.486894964346863));
#50347=CARTESIAN_POINT('Ctrl Pts',(0.10226912842285,-0.0478115777644791,
-0.479819334890221));
#50348=CARTESIAN_POINT('Ctrl Pts',(0.0962085431136162,0.0590682350665474,
-0.472743705433579));
#50349=CARTESIAN_POINT('Ctrl Pts',(0.00363743500867127,0.112835759078637,
-0.465668075976936));
#50350=CARTESIAN_POINT('Ctrl Pts',(-0.0922037598728345,0.0651425048758612,
-0.458592446520295));
#50351=CARTESIAN_POINT('Ctrl Pts',(-0.105137029505605,-0.0411256535495477,
-0.451516817063652));
#50352=CARTESIAN_POINT('Ctrl Pts',(-0.0235324529605039,-0.110414375714813,
-0.44444118760701));
#50353=CARTESIAN_POINT('Ctrl Pts',(0.07923206509802,-0.0804200407641335,
-0.437365558150368));
#50354=CARTESIAN_POINT('Ctrl Pts',(0.110752326466076,0.0218867699872954,
-0.430289928693726));
#50355=CARTESIAN_POINT('Ctrl Pts',(0.0426857011445824,0.104513340790562,
-0.423214299237084));
#50356=CARTESIAN_POINT('Ctrl Pts',(-0.0637632642897446,0.0931630436816094,
-0.416138669780442));
#50357=CARTESIAN_POINT('Ctrl Pts',(-0.11287724880361,-0.00195808426009219,
-0.409063040323799));
#50358=CARTESIAN_POINT('Ctrl Pts',(-0.0604936699172284,-0.0953185347786495,
-0.401987410867158));
#50359=CARTESIAN_POINT('Ctrl Pts',(0.0462849239846546,-0.102969961087666,
-0.394911781410515));
#50360=CARTESIAN_POINT('Ctrl Pts',(0.111444796996209,-0.0180323158387254,
-0.387836151953873));
#50361=CARTESIAN_POINT('Ctrl Pts',(0.0763951494091263,0.0831197226767399,
-0.380760522497231));
#50362=CARTESIAN_POINT('Ctrl Pts',(-0.0273478910507391,0.109531730550394,
-0.373684893040589));
#50363=CARTESIAN_POINT('Ctrl Pts',(-0.106500110824037,0.0374544196752633,
-0.366609263583947));
#50364=CARTESIAN_POINT('Ctrl Pts',(-0.0898889994490478,-0.0683013537911051,
-0.359533634127305));
#50365=CARTESIAN_POINT('Ctrl Pts',(0.00754897625919715,-0.112641555869212,
-0.352458004670662));
#50366=CARTESIAN_POINT('Ctrl Pts',(0.0981990237225277,-0.0556961299676074,
-0.345382375214021));
#50367=CARTESIAN_POINT('Ctrl Pts',(0.100549955365708,0.0513304356908642,
-0.338306745757378));
#50368=CARTESIAN_POINT('Ctrl Pts',(0.0124878480988304,0.11220142959062,
-0.331231116300736));
#50369=CARTESIAN_POINT('Ctrl Pts',(-0.0868031482546871,0.0721825505623247,
-0.324155486844094));
#50370=CARTESIAN_POINT('Ctrl Pts',(-0.108042032174805,-0.0327418147933531,
-0.317079857387452));
#50371=CARTESIAN_POINT('Ctrl Pts',(-0.0321311120597763,-0.108225222523459,
-0.31000422793081));
#50372=CARTESIAN_POINT('Ctrl Pts',(0.0726716307772531,-0.0863941041545113,
-0.302928598474167));
#50373=CARTESIAN_POINT('Ctrl Pts',(0.112129113562205,0.0131213202160467,
-0.295852969017526));
#50374=CARTESIAN_POINT('Ctrl Pts',(0.050761748924207,0.100838246705403,
-0.288777339560883));
#50375=CARTESIAN_POINT('Ctrl Pts',(-0.0562498327028107,0.0978829069520032,
-0.281701710104242));
#50376=CARTESIAN_POINT('Ctrl Pts',(-0.112682393238285,0.0069126989343267,
-0.274626080647599));
#50377=CARTESIAN_POINT('Ctrl Pts',(-0.0677926054149375,-0.0902733061514795,
-0.267550451190957));
#50378=CARTESIAN_POINT('Ctrl Pts',(0.038055294715108,-0.106286883935013,
-0.260474821734315));
#50379=CARTESIAN_POINT('Ctrl Pts',(0.10968443433419,-0.0267288611289883,
-0.253399192277673));
#50380=CARTESIAN_POINT('Ctrl Pts',(0.0826869460855996,0.0768633599284799,
-0.246323562821031));
#50381=CARTESIAN_POINT('Ctrl Pts',(-0.0186614262296518,0.111341179819334,
-0.239247933364389));
#50382=CARTESIAN_POINT('Ctrl Pts',(-0.103229718933756,0.0457026507033001,
-0.232172303907746));
#50383=CARTESIAN_POINT('Ctrl Pts',(-0.094975368790062,-0.0610310287936844,
-0.225096674451104));
#50384=CARTESIAN_POINT('Ctrl Pts',(-0.00132056587373289,-0.112886506095197,
-0.218021044994462));
#50385=CARTESIAN_POINT('Ctrl Pts',(0.0935216704263627,-0.0632360997609839,
-0.21094541553782));
#50386=CARTESIAN_POINT('Ctrl Pts',(0.104270598111585,0.04327527610209,-0.203869786081178));
#50387=CARTESIAN_POINT('Ctrl Pts',(0.0212609397230408,0.110874161081468,
-0.196794156624536));
#50388=CARTESIAN_POINT('Ctrl Pts',(-0.0808662425232999,0.0787766334096698,
-0.189718527167894));
#50389=CARTESIAN_POINT('Ctrl Pts',(-0.110279690529448,-0.0241556827346662,
-0.182642897711252));
#50390=CARTESIAN_POINT('Ctrl Pts',(-0.040531265065401,-0.105367564795535,
-0.17556726825461));
#50391=CARTESIAN_POINT('Ctrl Pts',(0.0656622769832545,-0.0918344843926382,
-0.168491638797967));
#50392=CARTESIAN_POINT('Ctrl Pts',(0.112813266670755,0.00427481159513008,
-0.161416009341325));
#50393=CARTESIAN_POINT('Ctrl Pts',(0.0585242285435791,0.0965402603342907,
-0.154340379884683));
#50394=CARTESIAN_POINT('Ctrl Pts',(-0.0483889339301513,0.10199812815814,
-0.147264750428041));
#50395=CARTESIAN_POINT('Ctrl Pts',(-0.111791479684098,0.0157407827773292,
-0.140189120971399));
#50396=CARTESIAN_POINT('Ctrl Pts',(-0.0746727734737821,-0.0846704452165861,
-0.133113491514757));
#50397=CARTESIAN_POINT('Ctrl Pts',(0.0295905909193192,-0.108947251043571,
-0.126037862058114));
#50398=CARTESIAN_POINT('Ctrl Pts',(0.107246531607553,-0.0352603026583548,
-0.118962232601472));
#50399=CARTESIAN_POINT('Ctrl Pts',(0.0884679709853073,0.0701322082061288,
-0.11188660314483));
#50400=CARTESIAN_POINT('Ctrl Pts',(-0.00985968677826821,0.112462836852163,
-0.104810973688188));
#50401=CARTESIAN_POINT('Ctrl Pts',(-0.0993216582114113,0.0536686027111373,
-0.097735344231546));
#50402=CARTESIAN_POINT('Ctrl Pts',(-0.0994750597131893,-0.053383769520308,
-0.0906597147749039));
#50403=CARTESIAN_POINT('Ctrl Pts',(-0.0101819483175724,-0.112434012668085,
-0.0835840853182618));
#50404=CARTESIAN_POINT('Ctrl Pts',(0.0882666128350871,-0.0703856840480749,
-0.0765084558616196));
#50405=CARTESIAN_POINT('Ctrl Pts',(0.107347151344391,0.0349532439147777,
-0.0694328264049776));
#50406=CARTESIAN_POINT('Ctrl Pts',(0.0299026828266366,0.108861155406636,
-0.0623571969483354));
#50407=CARTESIAN_POINT('Ctrl Pts',(-0.0744297814498727,0.0848857094486392,
-0.0552815674916933));
#50408=CARTESIAN_POINT('Ctrl Pts',(-0.111836189263656,-0.0154233953270265,
-0.048205938035051));
#50409=CARTESIAN_POINT('Ctrl Pts',(-0.0486809400150489,-0.101853223691883,
-0.041130308578409));
#50410=CARTESIAN_POINT('Ctrl Pts',(0.0582471077856237,-0.0967186223643828,
-0.0340546791217668));
#50411=CARTESIAN_POINT('Ctrl Pts',(0.112800950445628,-0.0045771260688116,
-0.0269790496651248));
#50412=CARTESIAN_POINT('Ctrl Pts',(0.0659244098700261,0.0916059362560433,
-0.0199034202084826));
#50413=CARTESIAN_POINT('Ctrl Pts',(-0.040227405207391,0.105560518034527,
-0.0128277907518405));
#50414=CARTESIAN_POINT('Ctrl Pts',(-0.110215223443824,0.0243141707662,-0.00575216129519839));
#50415=CARTESIAN_POINT('Ctrl Pts',(-0.0907859310257796,-0.044001857441111,
-0.00103507499077024));
#50416=CARTESIAN_POINT('Ctrl Pts',(-0.0688308846249437,-0.0666688828971034,
0.0013234681614438));
#50417=CARTESIAN_POINT('Ctrl Pts',(-0.0872731800879813,-0.0845318995251544,
-0.0134999999999998));
#50418=CARTESIAN_POINT('Ctrl Pts',(-0.108954027555681,-0.0621479649852055,
-0.0153369116616685));
#50419=CARTESIAN_POINT('Ctrl Pts',(-0.121220706757624,-0.0309262392804433,
-0.0171738233233372));
#50420=CARTESIAN_POINT('Ctrl Pts',(-0.121508540285962,0.000130861710946541,
-0.0190107349850059));
#50421=CARTESIAN_POINT('Origin',(0.,0.,-0.29));
#50422=CARTESIAN_POINT('Origin',(0.,0.,-0.0135));
#50423=CARTESIAN_POINT('Origin',(0.228475398698832,-0.0402863772187279,
0.04));
#50424=CARTESIAN_POINT('',(0.221856282657939,-0.0374805262129628,0.04));
#50425=CARTESIAN_POINT('',(0.221295806635937,-0.0406591436868745,0.04));
#50426=CARTESIAN_POINT('Origin',(0.,0.,0.04));
#50427=CARTESIAN_POINT('',(0.215672897909674,-0.0380289509090578,0.04));
#50428=CARTESIAN_POINT('',(0.24249343673166,-0.0356501492573125,0.04));
#50429=CARTESIAN_POINT('',(0.215672897909674,-0.0380289509090578,0.04));
#50430=CARTESIAN_POINT('Origin',(0.215672897909674,-0.0380289509090578,
0.04));
#50431=CARTESIAN_POINT('',(0.221295806635937,-0.0406591436868745,0.235));
#50432=CARTESIAN_POINT('',(0.221295806635937,-0.0406591436868745,0.1175));
#50433=CARTESIAN_POINT('',(0.215672897909674,-0.0380289509090578,0.241));
#50434=CARTESIAN_POINT('',(0.215672897909674,-0.0380289509090578,0.04));
#50435=CARTESIAN_POINT('Ctrl Pts',(0.221295806635937,-0.0406591436868745,
0.235));
#50436=CARTESIAN_POINT('Ctrl Pts',(0.218446359646244,-0.0393262757251279,
0.23804339528899));
#50437=CARTESIAN_POINT('Ctrl Pts',(0.215672897909674,-0.0380289509090578,
0.241));
#50438=CARTESIAN_POINT('Origin',(0.24249343673166,-0.0356501492573125,0.04));
#50439=CARTESIAN_POINT('',(0.221856282657939,-0.0374805262129628,0.235));
#50440=CARTESIAN_POINT('',(0.221856282657939,-0.0374805262129628,0.1175));
#50441=CARTESIAN_POINT('Ctrl Pts',(0.215672897909674,-0.0380289509090578,
0.241));
#50442=CARTESIAN_POINT('Ctrl Pts',(0.218722810657151,-0.0377584441332792,
0.238043395288934));
#50443=CARTESIAN_POINT('Ctrl Pts',(0.221856282657939,-0.0374805262129628,
0.235));
#50444=CARTESIAN_POINT('Origin',(0.218008688022331,-0.0793486732515553,
0.04));
#50445=CARTESIAN_POINT('',(0.211977362141128,-0.0754360519890137,0.04));
#50446=CARTESIAN_POINT('',(0.210873439877438,-0.0784690534813354,0.04));
#50447=CARTESIAN_POINT('Origin',(0.,0.,0.04));
#50448=CARTESIAN_POINT('',(0.205792683952114,-0.0749024113883216,0.04));
#50449=CARTESIAN_POINT('',(0.232618833095827,-0.0772170867692877,0.04));
#50450=CARTESIAN_POINT('',(0.205792683952114,-0.0749024113883216,0.04));
#50451=CARTESIAN_POINT('Origin',(0.205792683952114,-0.0749024113883216,
0.04));
#50452=CARTESIAN_POINT('',(0.210873439877438,-0.0784690534813354,0.235));
#50453=CARTESIAN_POINT('',(0.210873439877438,-0.0784690534813354,0.1175));
#50454=CARTESIAN_POINT('',(0.205792683952114,-0.0749024113883216,0.241));
#50455=CARTESIAN_POINT('',(0.205792683952114,-0.0749024113883216,0.04));
#50456=CARTESIAN_POINT('Ctrl Pts',(0.210873439877438,-0.0784690534813354,
0.235));
#50457=CARTESIAN_POINT('Ctrl Pts',(0.208298732482818,-0.0766616335017468,
0.23804339528899));
#50458=CARTESIAN_POINT('Ctrl Pts',(0.205792683952114,-0.0749024113883216,
0.241));
#50459=CARTESIAN_POINT('Origin',(0.232618833095827,-0.0772170867692877,
0.04));
#50460=CARTESIAN_POINT('',(0.211977362141128,-0.0754360519890138,0.235));
#50461=CARTESIAN_POINT('',(0.211977362141128,-0.0754360519890138,0.1175));
#50462=CARTESIAN_POINT('Ctrl Pts',(0.205792683952114,-0.0749024113883216,
0.241));
#50463=CARTESIAN_POINT('Ctrl Pts',(0.20884323468045,-0.0751656260089308,
0.238043395288983));
#50464=CARTESIAN_POINT('Ctrl Pts',(0.211977362141128,-0.0754360519890137,
0.235));
#50465=CARTESIAN_POINT('Origin',(0.20091789367799,-0.116,0.04));
#50466=CARTESIAN_POINT('',(0.195657616741379,-0.111099491497862,0.04));
#50467=CARTESIAN_POINT('',(0.194043790355372,-0.113894720793023,0.04));
#50468=CARTESIAN_POINT('Origin',(0.,0.,0.04));
#50469=CARTESIAN_POINT('',(0.189659563428792,-0.1095,0.04));
#50470=CARTESIAN_POINT('',(0.215676223927187,-0.116437822173509,0.04));
#50471=CARTESIAN_POINT('',(0.189659563428792,-0.1095,0.04));
#50472=CARTESIAN_POINT('Origin',(0.189659563428792,-0.1095,0.04));
#50473=CARTESIAN_POINT('',(0.194043790355372,-0.113894720793023,0.235));
#50474=CARTESIAN_POINT('',(0.194043790355372,-0.113894720793023,0.1175));
#50475=CARTESIAN_POINT('',(0.189659563428792,-0.1095,0.241));
#50476=CARTESIAN_POINT('',(0.189659563428792,-0.1095,0.04));
#50477=CARTESIAN_POINT('Ctrl Pts',(0.194043790355372,-0.113894720793023,
0.235));
#50478=CARTESIAN_POINT('Ctrl Pts',(0.191822053737127,-0.111667666337054,
0.238043395289017));
#50479=CARTESIAN_POINT('Ctrl Pts',(0.189659563428792,-0.1095,0.241));
#50480=CARTESIAN_POINT('Origin',(0.215676223927187,-0.116437822173509,0.04));
#50481=CARTESIAN_POINT('',(0.195657616741379,-0.111099491497862,0.235));
#50482=CARTESIAN_POINT('',(0.195657616741379,-0.111099491497862,0.1175));
#50483=CARTESIAN_POINT('Ctrl Pts',(0.189659563428792,-0.1095,0.241));
#50484=CARTESIAN_POINT('Ctrl Pts',(0.192618062697872,-0.110288938373955,
0.238043395288922));
#50485=CARTESIAN_POINT('Ctrl Pts',(0.195657616741379,-0.111099491497863,
0.235));
#50486=CARTESIAN_POINT('Origin',(0.177722310803603,-0.149126725447277,0.04));
#50487=CARTESIAN_POINT('',(0.173392913664475,-0.143387229176604,0.04));
#50488=CARTESIAN_POINT('',(0.171318218454253,-0.145859754646924,0.04));
#50489=CARTESIAN_POINT('Origin',(0.,0.,0.04));
#50490=CARTESIAN_POINT('',(0.167763733043056,-0.140770486521352,0.04));
#50491=CARTESIAN_POINT('',(0.192180401831955,-0.152120653271369,0.04));
#50492=CARTESIAN_POINT('',(0.167763733043056,-0.140770486521352,0.04));
#50493=CARTESIAN_POINT('Origin',(0.167763733043056,-0.140770486521352,0.04));
#50494=CARTESIAN_POINT('',(0.171318218454253,-0.145859754646924,0.235));
#50495=CARTESIAN_POINT('',(0.171318218454253,-0.145859754646924,0.1175));
#50496=CARTESIAN_POINT('',(0.167763733043056,-0.140770486521352,0.241));
#50497=CARTESIAN_POINT('',(0.167763733043056,-0.140770486521352,0.04));
#50498=CARTESIAN_POINT('Ctrl Pts',(0.171318218454253,-0.145859754646924,
0.235));
#50499=CARTESIAN_POINT('Ctrl Pts',(0.169516958955325,-0.143280733637328,
0.238043395288973));
#50500=CARTESIAN_POINT('Ctrl Pts',(0.167763733043056,-0.140770486521352,
0.241));
#50501=CARTESIAN_POINT('Origin',(0.192180401831955,-0.152120653271369,0.04));
#50502=CARTESIAN_POINT('',(0.173392913664475,-0.143387229176604,0.235));
#50503=CARTESIAN_POINT('',(0.173392913664475,-0.143387229176604,0.1175));
#50504=CARTESIAN_POINT('Ctrl Pts',(0.167763733043056,-0.140770486521352,
0.241));
#50505=CARTESIAN_POINT('Ctrl Pts',(0.170540288349532,-0.142061177155346,
0.238043395288992));
#50506=CARTESIAN_POINT('Ctrl Pts',(0.173392913664475,-0.143387229176604,
0.235));
#50507=CARTESIAN_POINT('Origin',(0.149126725447277,-0.177722310803603,0.04));
#50508=CARTESIAN_POINT('',(0.145859754646924,-0.171318218454253,0.04));
#50509=CARTESIAN_POINT('',(0.143387229176604,-0.173392913664475,0.04));
#50510=CARTESIAN_POINT('Origin',(0.,0.,0.04));
#50511=CARTESIAN_POINT('',(0.140770486521352,-0.167763733043056,0.04));
#50512=CARTESIAN_POINT('',(0.162845275475035,-0.183181375296344,0.04));
#50513=CARTESIAN_POINT('',(0.140770486521352,-0.167763733043056,0.04));
#50514=CARTESIAN_POINT('Origin',(0.140770486521352,-0.167763733043056,0.04));
#50515=CARTESIAN_POINT('',(0.143387229176604,-0.173392913664475,0.235));
#50516=CARTESIAN_POINT('',(0.143387229176604,-0.173392913664475,0.1175));
#50517=CARTESIAN_POINT('',(0.140770486521352,-0.167763733043056,0.241));
#50518=CARTESIAN_POINT('',(0.140770486521352,-0.167763733043056,0.04));
#50519=CARTESIAN_POINT('Ctrl Pts',(0.143387229176604,-0.173392913664475,
0.235));
#50520=CARTESIAN_POINT('Ctrl Pts',(0.142061177155362,-0.170540288349568,
0.238043395288954));
#50521=CARTESIAN_POINT('Ctrl Pts',(0.140770486521352,-0.167763733043056,
0.241));
#50522=CARTESIAN_POINT('Origin',(0.162845275475035,-0.183181375296344,0.04));
#50523=CARTESIAN_POINT('',(0.145859754646924,-0.171318218454253,0.235));
#50524=CARTESIAN_POINT('',(0.145859754646924,-0.171318218454253,0.1175));
#50525=CARTESIAN_POINT('Ctrl Pts',(0.140770486521352,-0.167763733043056,
0.241));
#50526=CARTESIAN_POINT('Ctrl Pts',(0.143280733637332,-0.169516958955328,
0.238043395288968));
#50527=CARTESIAN_POINT('Ctrl Pts',(0.145859754646923,-0.171318218454253,
0.235));
#50528=CARTESIAN_POINT('Origin',(0.116,-0.20091789367799,0.04));
#50529=CARTESIAN_POINT('',(0.113894720793023,-0.194043790355372,0.04));
#50530=CARTESIAN_POINT('',(0.111099491497862,-0.195657616741379,0.04));
#50531=CARTESIAN_POINT('Origin',(0.,0.,0.04));
#50532=CARTESIAN_POINT('',(0.1095,-0.189659563428792,0.04));
#50533=CARTESIAN_POINT('',(0.128562177826491,-0.208676223927188,0.04));
#50534=CARTESIAN_POINT('',(0.1095,-0.189659563428792,0.04));
#50535=CARTESIAN_POINT('Origin',(0.1095,-0.189659563428792,0.04));
#50536=CARTESIAN_POINT('',(0.111099491497862,-0.195657616741379,0.235));
#50537=CARTESIAN_POINT('',(0.111099491497862,-0.195657616741379,0.1175));
#50538=CARTESIAN_POINT('',(0.1095,-0.189659563428792,0.241));
#50539=CARTESIAN_POINT('',(0.1095,-0.189659563428792,0.04));
#50540=CARTESIAN_POINT('Ctrl Pts',(0.111099491497862,-0.195657616741379,
0.235));
#50541=CARTESIAN_POINT('Ctrl Pts',(0.110288938373936,-0.192618062697803,
0.238043395288991));
#50542=CARTESIAN_POINT('Ctrl Pts',(0.1095,-0.189659563428792,0.241));
#50543=CARTESIAN_POINT('Origin',(0.128562177826491,-0.208676223927188,0.04));
#50544=CARTESIAN_POINT('',(0.113894720793023,-0.194043790355372,0.235));
#50545=CARTESIAN_POINT('',(0.113894720793023,-0.194043790355372,0.1175));
#50546=CARTESIAN_POINT('Ctrl Pts',(0.1095,-0.189659563428792,0.241));
#50547=CARTESIAN_POINT('Ctrl Pts',(0.111667666337076,-0.191822053737149,
0.238043395288987));
#50548=CARTESIAN_POINT('Ctrl Pts',(0.113894720793023,-0.194043790355372,
0.235));
#50549=CARTESIAN_POINT('Origin',(0.079348673251555,-0.218008688022331,0.04));
#50550=CARTESIAN_POINT('',(0.0784690534813351,-0.210873439877438,0.04));
#50551=CARTESIAN_POINT('',(0.0754360519890135,-0.211977362141128,0.04));
#50552=CARTESIAN_POINT('Origin',(0.,0.,0.04));
#50553=CARTESIAN_POINT('',(0.0749024113883213,-0.205792683952114,0.04));
#50554=CARTESIAN_POINT('',(0.0903727834602901,-0.227830551089268,0.04));
#50555=CARTESIAN_POINT('',(0.0749024113883213,-0.205792683952114,0.04));
#50556=CARTESIAN_POINT('Origin',(0.0749024113883213,-0.205792683952114,
0.04));
#50557=CARTESIAN_POINT('',(0.0754360519890135,-0.211977362141128,0.235));
#50558=CARTESIAN_POINT('',(0.0754360519890135,-0.211977362141128,0.1175));
#50559=CARTESIAN_POINT('',(0.0749024113883213,-0.205792683952114,0.241));
#50560=CARTESIAN_POINT('',(0.0749024113883213,-0.205792683952114,0.04));
#50561=CARTESIAN_POINT('Ctrl Pts',(0.0754360519890135,-0.211977362141128,
0.235));
#50562=CARTESIAN_POINT('Ctrl Pts',(0.075165626008936,-0.208843234680514,
0.238043395288922));
#50563=CARTESIAN_POINT('Ctrl Pts',(0.0749024113883213,-0.205792683952114,
0.241));
#50564=CARTESIAN_POINT('Origin',(0.0903727834602901,-0.227830551089268,
0.04));
#50565=CARTESIAN_POINT('',(0.0784690534813351,-0.210873439877438,0.235));
#50566=CARTESIAN_POINT('',(0.0784690534813351,-0.210873439877438,0.1175));
#50567=CARTESIAN_POINT('Ctrl Pts',(0.0749024113883213,-0.205792683952114,
0.241));
#50568=CARTESIAN_POINT('Ctrl Pts',(0.0766616335017888,-0.208298732482879,
0.238043395288919));
#50569=CARTESIAN_POINT('Ctrl Pts',(0.0784690534813351,-0.210873439877438,
0.235));
#50570=CARTESIAN_POINT('Origin',(0.0402863772187278,-0.228475398698832,
0.04));
#50571=CARTESIAN_POINT('',(0.0406591436868744,-0.221295806635937,0.04));
#50572=CARTESIAN_POINT('',(0.0374805262129627,-0.221856282657939,0.04));
#50573=CARTESIAN_POINT('Origin',(0.,0.,0.04));
#50574=CARTESIAN_POINT('',(0.0380289509090577,-0.215672897909674,0.04));
#50575=CARTESIAN_POINT('',(0.0494374577994833,-0.240062362244323,0.04));
#50576=CARTESIAN_POINT('',(0.0380289509090577,-0.215672897909674,0.04));
#50577=CARTESIAN_POINT('Origin',(0.0380289509090577,-0.215672897909674,
0.04));
#50578=CARTESIAN_POINT('',(0.0374805262129627,-0.221856282657939,0.235));
#50579=CARTESIAN_POINT('',(0.0374805262129627,-0.221856282657939,0.1175));
#50580=CARTESIAN_POINT('',(0.0380289509090577,-0.215672897909674,0.241));
#50581=CARTESIAN_POINT('',(0.0380289509090577,-0.215672897909674,0.04));
#50582=CARTESIAN_POINT('Ctrl Pts',(0.0374805262129627,-0.221856282657939,
0.235));
#50583=CARTESIAN_POINT('Ctrl Pts',(0.0377584441332851,-0.218722810657084,
0.238043395288999));
#50584=CARTESIAN_POINT('Ctrl Pts',(0.0380289509090577,-0.215672897909674,
0.241));
#50585=CARTESIAN_POINT('Origin',(0.0494374577994833,-0.240062362244323,
0.04));
#50586=CARTESIAN_POINT('',(0.0406591436868744,-0.221295806635937,0.235));
#50587=CARTESIAN_POINT('',(0.0406591436868744,-0.221295806635937,0.1175));
#50588=CARTESIAN_POINT('Ctrl Pts',(0.0380289509090577,-0.215672897909674,
0.241));
#50589=CARTESIAN_POINT('Ctrl Pts',(0.0393262757251536,-0.218446359646299,
0.238043395288931));
#50590=CARTESIAN_POINT('Ctrl Pts',(0.0406591436868744,-0.221295806635937,
0.235));
#50591=CARTESIAN_POINT('Origin',(-4.16333634234434E-17,-0.232,0.04));
#50592=CARTESIAN_POINT('',(0.00161382638600745,-0.224994212290885,0.04));
#50593=CARTESIAN_POINT('',(-0.00161382638600754,-0.224994212290885,0.04));
#50594=CARTESIAN_POINT('Origin',(0.,0.,0.04));
#50595=CARTESIAN_POINT('',(-4.16333634234434E-17,-0.219,0.04));
#50596=CARTESIAN_POINT('',(0.00699999999999996,-0.245,0.04));
#50597=CARTESIAN_POINT('',(-4.16333634234434E-17,-0.219,0.04));
#50598=CARTESIAN_POINT('Origin',(-4.16333634234434E-17,-0.219,0.04));
#50599=CARTESIAN_POINT('',(-0.00161382638600754,-0.224994212290885,0.235));
#50600=CARTESIAN_POINT('',(-0.00161382638600754,-0.224994212290885,0.1175));
#50601=CARTESIAN_POINT('',(-4.16333634234434E-17,-0.219,0.241));
#50602=CARTESIAN_POINT('',(-4.16333634234434E-17,-0.219,0.04));
#50603=CARTESIAN_POINT('Ctrl Pts',(-0.00161382638600753,-0.224994212290885,
0.235));
#50604=CARTESIAN_POINT('Ctrl Pts',(-0.000796008960679004,-0.221956604711093,
0.238043395288907));
#50605=CARTESIAN_POINT('Ctrl Pts',(-4.16333634234434E-17,-0.219,0.241));
#50606=CARTESIAN_POINT('Origin',(0.00699999999999996,-0.245,0.04));
#50607=CARTESIAN_POINT('',(0.00161382638600745,-0.224994212290885,0.235));
#50608=CARTESIAN_POINT('',(0.00161382638600745,-0.224994212290885,0.1175));
#50609=CARTESIAN_POINT('Ctrl Pts',(-4.16333634234434E-17,-0.219,0.241));
#50610=CARTESIAN_POINT('Ctrl Pts',(0.000796008960667156,-0.22195660471105,
0.23804339528895));
#50611=CARTESIAN_POINT('Ctrl Pts',(0.00161382638600743,-0.224994212290885,
0.235));
#50612=CARTESIAN_POINT('Origin',(-0.0402863772187278,-0.228475398698832,
0.04));
#50613=CARTESIAN_POINT('',(-0.0374805262129628,-0.221856282657939,0.04));
#50614=CARTESIAN_POINT('',(-0.0406591436868745,-0.221295806635937,0.04));
#50615=CARTESIAN_POINT('Origin',(0.,0.,0.04));
#50616=CARTESIAN_POINT('',(-0.0380289509090577,-0.215672897909674,0.04));
#50617=CARTESIAN_POINT('',(-0.0356501492573125,-0.24249343673166,0.04));
#50618=CARTESIAN_POINT('',(-0.0380289509090577,-0.215672897909674,0.04));
#50619=CARTESIAN_POINT('Origin',(-0.0380289509090577,-0.215672897909674,
0.04));
#50620=CARTESIAN_POINT('',(-0.0406591436868745,-0.221295806635937,0.235));
#50621=CARTESIAN_POINT('',(-0.0406591436868745,-0.221295806635937,0.1175));
#50622=CARTESIAN_POINT('',(-0.0380289509090577,-0.215672897909674,0.241));
#50623=CARTESIAN_POINT('',(-0.0380289509090577,-0.215672897909674,0.04));
#50624=CARTESIAN_POINT('Ctrl Pts',(-0.0406591436868745,-0.221295806635937,
0.235));
#50625=CARTESIAN_POINT('Ctrl Pts',(-0.0393262757251577,-0.218446359646308,
0.238043395288922));
#50626=CARTESIAN_POINT('Ctrl Pts',(-0.0380289509090577,-0.215672897909674,
0.241));
#50627=CARTESIAN_POINT('Origin',(-0.0356501492573125,-0.24249343673166,
0.04));
#50628=CARTESIAN_POINT('',(-0.0374805262129628,-0.221856282657939,0.235));
#50629=CARTESIAN_POINT('',(-0.0374805262129628,-0.221856282657939,0.1175));
#50630=CARTESIAN_POINT('Ctrl Pts',(-0.0380289509090577,-0.215672897909674,
0.241));
#50631=CARTESIAN_POINT('Ctrl Pts',(-0.0377584441332853,-0.218722810657082,
0.238043395289));
#50632=CARTESIAN_POINT('Ctrl Pts',(-0.0374805262129628,-0.221856282657939,
0.235));
#50633=CARTESIAN_POINT('Origin',(-0.0793486732515553,-0.218008688022331,
0.04));
#50634=CARTESIAN_POINT('',(-0.0754360519890138,-0.211977362141128,0.04));
#50635=CARTESIAN_POINT('',(-0.0784690534813354,-0.210873439877438,0.04));
#50636=CARTESIAN_POINT('Origin',(0.,0.,0.04));
#50637=CARTESIAN_POINT('',(-0.0749024113883216,-0.205792683952114,0.04));
#50638=CARTESIAN_POINT('',(-0.0772170867692877,-0.232618833095827,0.04));
#50639=CARTESIAN_POINT('',(-0.0749024113883216,-0.205792683952114,0.04));
#50640=CARTESIAN_POINT('Origin',(-0.0749024113883216,-0.205792683952114,
0.04));
#50641=CARTESIAN_POINT('',(-0.0784690534813354,-0.210873439877438,0.235));
#50642=CARTESIAN_POINT('',(-0.0784690534813354,-0.210873439877438,0.1175));
#50643=CARTESIAN_POINT('',(-0.0749024113883216,-0.205792683952114,0.241));
#50644=CARTESIAN_POINT('',(-0.0749024113883216,-0.205792683952114,0.04));
#50645=CARTESIAN_POINT('Ctrl Pts',(-0.0784690534813354,-0.210873439877438,
0.235));
#50646=CARTESIAN_POINT('Ctrl Pts',(-0.0766616335017839,-0.208298732482871,
0.238043395288928));
#50647=CARTESIAN_POINT('Ctrl Pts',(-0.0749024113883216,-0.205792683952114,
0.241));
#50648=CARTESIAN_POINT('Origin',(-0.0772170867692877,-0.232618833095827,
0.04));
#50649=CARTESIAN_POINT('',(-0.0754360519890137,-0.211977362141128,0.235));
#50650=CARTESIAN_POINT('',(-0.0754360519890137,-0.211977362141128,0.1175));
#50651=CARTESIAN_POINT('Ctrl Pts',(-0.0749024113883216,-0.205792683952114,
0.241));
#50652=CARTESIAN_POINT('Ctrl Pts',(-0.0751656260089316,-0.208843234680459,
0.238043395288975));
#50653=CARTESIAN_POINT('Ctrl Pts',(-0.0754360519890138,-0.211977362141128,
0.235));
#50654=CARTESIAN_POINT('Origin',(-0.116,-0.20091789367799,0.04));
#50655=CARTESIAN_POINT('',(-0.111099491497862,-0.195657616741379,0.04));
#50656=CARTESIAN_POINT('',(-0.113894720793023,-0.194043790355372,0.04));
#50657=CARTESIAN_POINT('Origin',(0.,0.,0.04));
#50658=CARTESIAN_POINT('',(-0.1095,-0.189659563428792,0.04));
#50659=CARTESIAN_POINT('',(-0.116437822173509,-0.215676223927187,0.04));
#50660=CARTESIAN_POINT('',(-0.1095,-0.189659563428792,0.04));
#50661=CARTESIAN_POINT('Origin',(-0.1095,-0.189659563428792,0.04));
#50662=CARTESIAN_POINT('',(-0.113894720793023,-0.194043790355372,0.235));
#50663=CARTESIAN_POINT('',(-0.113894720793023,-0.194043790355372,0.1175));
#50664=CARTESIAN_POINT('',(-0.1095,-0.189659563428792,0.241));
#50665=CARTESIAN_POINT('',(-0.1095,-0.189659563428792,0.04));
#50666=CARTESIAN_POINT('Ctrl Pts',(-0.113894720793023,-0.194043790355372,
0.235));
#50667=CARTESIAN_POINT('Ctrl Pts',(-0.111667666337054,-0.191822053737127,
0.238043395289017));
#50668=CARTESIAN_POINT('Ctrl Pts',(-0.1095,-0.189659563428792,0.241));
#50669=CARTESIAN_POINT('Origin',(-0.116437822173509,-0.215676223927187,
0.04));
#50670=CARTESIAN_POINT('',(-0.111099491497862,-0.195657616741379,0.235));
#50671=CARTESIAN_POINT('',(-0.111099491497862,-0.195657616741379,0.1175));
#50672=CARTESIAN_POINT('Ctrl Pts',(-0.1095,-0.189659563428792,0.241));
#50673=CARTESIAN_POINT('Ctrl Pts',(-0.110288938373955,-0.192618062697872,
0.238043395288922));
#50674=CARTESIAN_POINT('Ctrl Pts',(-0.111099491497863,-0.195657616741379,
0.235));
#50675=CARTESIAN_POINT('Origin',(-0.149126725447277,-0.177722310803603,
0.04));
#50676=CARTESIAN_POINT('',(-0.143387229176604,-0.173392913664475,0.04));
#50677=CARTESIAN_POINT('',(-0.145859754646924,-0.171318218454253,0.04));
#50678=CARTESIAN_POINT('Origin',(0.,0.,0.04));
#50679=CARTESIAN_POINT('',(-0.140770486521352,-0.167763733043056,0.04));
#50680=CARTESIAN_POINT('',(-0.152120653271369,-0.192180401831955,0.04));
#50681=CARTESIAN_POINT('',(-0.140770486521352,-0.167763733043056,0.04));
#50682=CARTESIAN_POINT('Origin',(-0.140770486521352,-0.167763733043056,
0.04));
#50683=CARTESIAN_POINT('',(-0.145859754646924,-0.171318218454253,0.235));
#50684=CARTESIAN_POINT('',(-0.145859754646924,-0.171318218454253,0.1175));
#50685=CARTESIAN_POINT('',(-0.140770486521352,-0.167763733043056,0.241));
#50686=CARTESIAN_POINT('',(-0.140770486521352,-0.167763733043056,0.04));
#50687=CARTESIAN_POINT('Ctrl Pts',(-0.145859754646924,-0.171318218454253,
0.235));
#50688=CARTESIAN_POINT('Ctrl Pts',(-0.143280733637303,-0.169516958955308,
0.238043395289003));
#50689=CARTESIAN_POINT('Ctrl Pts',(-0.140770486521352,-0.167763733043056,
0.241));
#50690=CARTESIAN_POINT('Origin',(-0.152120653271369,-0.192180401831955,
0.04));
#50691=CARTESIAN_POINT('',(-0.143387229176604,-0.173392913664475,0.235));
#50692=CARTESIAN_POINT('',(-0.143387229176604,-0.173392913664475,0.1175));
#50693=CARTESIAN_POINT('Ctrl Pts',(-0.140770486521352,-0.167763733043056,
0.241));
#50694=CARTESIAN_POINT('Ctrl Pts',(-0.142061177155329,-0.170540288349497,
0.238043395289029));
#50695=CARTESIAN_POINT('Ctrl Pts',(-0.143387229176604,-0.173392913664475,
0.235));
#50696=CARTESIAN_POINT('Origin',(-0.177722310803603,-0.149126725447277,
0.04));
#50697=CARTESIAN_POINT('',(-0.171318218454253,-0.145859754646924,0.04));
#50698=CARTESIAN_POINT('',(-0.173392913664475,-0.143387229176604,0.04));
#50699=CARTESIAN_POINT('Origin',(0.,0.,0.04));
#50700=CARTESIAN_POINT('',(-0.167763733043056,-0.140770486521352,0.04));
#50701=CARTESIAN_POINT('',(-0.183181375296344,-0.162845275475035,0.04));
#50702=CARTESIAN_POINT('',(-0.167763733043056,-0.140770486521352,0.04));
#50703=CARTESIAN_POINT('Origin',(-0.167763733043056,-0.140770486521352,
0.04));
#50704=CARTESIAN_POINT('',(-0.173392913664475,-0.143387229176604,0.235));
#50705=CARTESIAN_POINT('',(-0.173392913664475,-0.143387229176604,0.1175));
#50706=CARTESIAN_POINT('',(-0.167763733043056,-0.140770486521352,0.241));
#50707=CARTESIAN_POINT('',(-0.167763733043056,-0.140770486521352,0.04));
#50708=CARTESIAN_POINT('Ctrl Pts',(-0.173392913664475,-0.143387229176604,
0.235));
#50709=CARTESIAN_POINT('Ctrl Pts',(-0.170540288349525,-0.142061177155342,
0.238043395288999));
#50710=CARTESIAN_POINT('Ctrl Pts',(-0.167763733043056,-0.140770486521352,
0.241));
#50711=CARTESIAN_POINT('Origin',(-0.183181375296344,-0.162845275475035,
0.04));
#50712=CARTESIAN_POINT('',(-0.171318218454253,-0.145859754646924,0.235));
#50713=CARTESIAN_POINT('',(-0.171318218454253,-0.145859754646924,0.1175));
#50714=CARTESIAN_POINT('Ctrl Pts',(-0.167763733043056,-0.140770486521352,
0.241));
#50715=CARTESIAN_POINT('Ctrl Pts',(-0.169516958955354,-0.14328073363737,
0.238043395288925));
#50716=CARTESIAN_POINT('Ctrl Pts',(-0.171318218454253,-0.145859754646924,
0.235));
#50717=CARTESIAN_POINT('Origin',(-0.20091789367799,-0.116,0.04));
#50718=CARTESIAN_POINT('',(-0.194043790355372,-0.113894720793023,0.04));
#50719=CARTESIAN_POINT('',(-0.195657616741379,-0.111099491497862,0.04));
#50720=CARTESIAN_POINT('Origin',(0.,0.,0.04));
#50721=CARTESIAN_POINT('',(-0.189659563428792,-0.1095,0.04));
#50722=CARTESIAN_POINT('',(-0.208676223927188,-0.128562177826491,0.04));
#50723=CARTESIAN_POINT('',(-0.189659563428792,-0.1095,0.04));
#50724=CARTESIAN_POINT('Origin',(-0.189659563428792,-0.1095,0.04));
#50725=CARTESIAN_POINT('',(-0.195657616741379,-0.111099491497862,0.235));
#50726=CARTESIAN_POINT('',(-0.195657616741379,-0.111099491497862,0.1175));
#50727=CARTESIAN_POINT('',(-0.189659563428792,-0.1095,0.241));
#50728=CARTESIAN_POINT('',(-0.189659563428792,-0.1095,0.04));
#50729=CARTESIAN_POINT('Ctrl Pts',(-0.195657616741379,-0.111099491497862,
0.235));
#50730=CARTESIAN_POINT('Ctrl Pts',(-0.192618062697799,-0.110288938373935,
0.238043395288995));
#50731=CARTESIAN_POINT('Ctrl Pts',(-0.189659563428792,-0.1095,0.241));
#50732=CARTESIAN_POINT('Origin',(-0.208676223927188,-0.128562177826491,
0.04));
#50733=CARTESIAN_POINT('',(-0.194043790355372,-0.113894720793023,0.235));
#50734=CARTESIAN_POINT('',(-0.194043790355372,-0.113894720793023,0.1175));
#50735=CARTESIAN_POINT('Ctrl Pts',(-0.189659563428792,-0.1095,0.241));
#50736=CARTESIAN_POINT('Ctrl Pts',(-0.191822053737133,-0.111667666337059,
0.238043395289009));
#50737=CARTESIAN_POINT('Ctrl Pts',(-0.194043790355372,-0.113894720793023,
0.235));
#50738=CARTESIAN_POINT('Origin',(-0.218008688022331,-0.0793486732515551,
0.04));
#50739=CARTESIAN_POINT('',(-0.210873439877438,-0.0784690534813352,0.04));
#50740=CARTESIAN_POINT('',(-0.211977362141128,-0.0754360519890136,0.04));
#50741=CARTESIAN_POINT('Origin',(0.,0.,0.04));
#50742=CARTESIAN_POINT('',(-0.205792683952114,-0.0749024113883215,0.04));
#50743=CARTESIAN_POINT('',(-0.227830551089268,-0.0903727834602902,0.04));
#50744=CARTESIAN_POINT('',(-0.205792683952114,-0.0749024113883215,0.04));
#50745=CARTESIAN_POINT('Origin',(-0.205792683952114,-0.0749024113883215,
0.04));
#50746=CARTESIAN_POINT('',(-0.211977362141128,-0.0754360519890136,0.235));
#50747=CARTESIAN_POINT('',(-0.211977362141128,-0.0754360519890136,0.1175));
#50748=CARTESIAN_POINT('',(-0.205792683952114,-0.0749024113883215,0.241));
#50749=CARTESIAN_POINT('',(-0.205792683952114,-0.0749024113883215,0.04));
#50750=CARTESIAN_POINT('Ctrl Pts',(-0.211977362141128,-0.0754360519890136,
0.235));
#50751=CARTESIAN_POINT('Ctrl Pts',(-0.208843234680406,-0.0751656260089268,
0.238043395289026));
#50752=CARTESIAN_POINT('Ctrl Pts',(-0.205792683952114,-0.0749024113883215,
0.241));
#50753=CARTESIAN_POINT('Origin',(-0.227830551089268,-0.0903727834602902,
0.04));
#50754=CARTESIAN_POINT('',(-0.210873439877438,-0.0784690534813352,0.235));
#50755=CARTESIAN_POINT('',(-0.210873439877438,-0.0784690534813352,0.1175));
#50756=CARTESIAN_POINT('Ctrl Pts',(-0.205792683952114,-0.0749024113883215,
0.241));
#50757=CARTESIAN_POINT('Ctrl Pts',(-0.208298732482853,-0.0766616335017707,
0.23804339528895));
#50758=CARTESIAN_POINT('Ctrl Pts',(-0.210873439877438,-0.0784690534813352,
0.235));
#50759=CARTESIAN_POINT('Origin',(-0.228475398698832,-0.0402863772187278,
0.04));
#50760=CARTESIAN_POINT('',(-0.221295806635937,-0.0406591436868744,0.04));
#50761=CARTESIAN_POINT('',(-0.221856282657939,-0.0374805262129627,0.04));
#50762=CARTESIAN_POINT('Origin',(0.,0.,0.04));
#50763=CARTESIAN_POINT('',(-0.215672897909674,-0.0380289509090577,0.04));
#50764=CARTESIAN_POINT('',(-0.240062362244323,-0.0494374577994833,0.04));
#50765=CARTESIAN_POINT('',(-0.215672897909674,-0.0380289509090577,0.04));
#50766=CARTESIAN_POINT('Origin',(-0.215672897909674,-0.0380289509090577,
0.04));
#50767=CARTESIAN_POINT('',(-0.221856282657939,-0.0374805262129627,0.235));
#50768=CARTESIAN_POINT('',(-0.221856282657939,-0.0374805262129627,0.1175));
#50769=CARTESIAN_POINT('',(-0.215672897909674,-0.0380289509090577,0.241));
#50770=CARTESIAN_POINT('',(-0.215672897909674,-0.0380289509090577,0.04));
#50771=CARTESIAN_POINT('Ctrl Pts',(-0.221856282657939,-0.0374805262129627,
0.235));
#50772=CARTESIAN_POINT('Ctrl Pts',(-0.218722810657085,-0.037758444133285,
0.238043395288998));
#50773=CARTESIAN_POINT('Ctrl Pts',(-0.215672897909674,-0.0380289509090577,
0.241));
#50774=CARTESIAN_POINT('Origin',(-0.240062362244323,-0.0494374577994833,
0.04));
#50775=CARTESIAN_POINT('',(-0.221295806635937,-0.0406591436868744,0.235));
#50776=CARTESIAN_POINT('',(-0.221295806635937,-0.0406591436868744,0.1175));
#50777=CARTESIAN_POINT('Ctrl Pts',(-0.215672897909674,-0.0380289509090577,
0.241));
#50778=CARTESIAN_POINT('Ctrl Pts',(-0.218446359646305,-0.0393262757251562,
0.238043395288925));
#50779=CARTESIAN_POINT('Ctrl Pts',(-0.221295806635937,-0.0406591436868744,
0.235));
#50780=CARTESIAN_POINT('Origin',(-0.232,2.77555756156289E-17,0.04));
#50781=CARTESIAN_POINT('',(-0.224994212290885,-0.00161382638600747,0.04));
#50782=CARTESIAN_POINT('',(-0.225,-2.75545529808154E-17,0.04));
#50783=CARTESIAN_POINT('Origin',(0.,0.,0.04));
#50784=CARTESIAN_POINT('',(-0.219,2.77555756156289E-17,0.04));
#50785=CARTESIAN_POINT('',(-0.245,-0.00699999999999998,0.04));
#50786=CARTESIAN_POINT('',(-0.224994212290885,0.00161382638600753,0.04));
#50787=CARTESIAN_POINT('',(-0.219,2.77555756156289E-17,0.04));
#50788=CARTESIAN_POINT('Origin',(0.,0.,0.04));
#50789=CARTESIAN_POINT('Origin',(-0.219,2.77555756156289E-17,0.04));
#50790=CARTESIAN_POINT('',(-0.224994212290885,0.00161382638600753,0.235));
#50791=CARTESIAN_POINT('',(-0.224994212290885,0.00161382638600753,0.1175));
#50792=CARTESIAN_POINT('',(-0.219,2.77555756156289E-17,0.241));
#50793=CARTESIAN_POINT('',(-0.219,2.77555756156289E-17,0.04));
#50794=CARTESIAN_POINT('Ctrl Pts',(-0.224994212290885,0.00161382638600752,
0.235));
#50795=CARTESIAN_POINT('Ctrl Pts',(-0.221956604711078,0.000796008960674882,
0.238043395288922));
#50796=CARTESIAN_POINT('Ctrl Pts',(-0.219,2.77555756156289E-17,0.241));
#50797=CARTESIAN_POINT('Origin',(-0.245,-0.00699999999999998,0.04));
#50798=CARTESIAN_POINT('',(-0.224994212290885,-0.00161382638600747,0.235));
#50799=CARTESIAN_POINT('',(-0.224994212290885,-0.00161382638600747,0.1175));
#50800=CARTESIAN_POINT('Ctrl Pts',(-0.219,2.77555756156289E-17,0.241));
#50801=CARTESIAN_POINT('Ctrl Pts',(-0.221956604711001,-0.000796008960654102,
0.238043395288999));
#50802=CARTESIAN_POINT('Ctrl Pts',(-0.224994212290885,-0.00161382638600745,
0.235));
#50803=CARTESIAN_POINT('Origin',(-0.228475398698832,0.0402863772187279,
0.04));
#50804=CARTESIAN_POINT('',(-0.221856282657939,0.0374805262129629,0.04));
#50805=CARTESIAN_POINT('',(-0.221295806635937,0.0406591436868746,0.04));
#50806=CARTESIAN_POINT('Origin',(0.,0.,0.04));
#50807=CARTESIAN_POINT('',(-0.215672897909674,0.0380289509090578,0.04));
#50808=CARTESIAN_POINT('',(-0.24249343673166,0.0356501492573126,0.04));
#50809=CARTESIAN_POINT('',(-0.215672897909674,0.0380289509090578,0.04));
#50810=CARTESIAN_POINT('Origin',(-0.215672897909674,0.0380289509090578,
0.04));
#50811=CARTESIAN_POINT('',(-0.221295806635937,0.0406591436868746,0.235));
#50812=CARTESIAN_POINT('',(-0.221295806635937,0.0406591436868746,0.1175));
#50813=CARTESIAN_POINT('',(-0.215672897909674,0.0380289509090578,0.241));
#50814=CARTESIAN_POINT('',(-0.215672897909674,0.0380289509090578,0.04));
#50815=CARTESIAN_POINT('Ctrl Pts',(-0.221295806635937,0.0406591436868746,
0.235));
#50816=CARTESIAN_POINT('Ctrl Pts',(-0.218446359646237,0.0393262757251244,
0.238043395288998));
#50817=CARTESIAN_POINT('Ctrl Pts',(-0.215672897909674,0.0380289509090578,
0.241));
#50818=CARTESIAN_POINT('Origin',(-0.24249343673166,0.0356501492573126,0.04));
#50819=CARTESIAN_POINT('',(-0.221856282657939,0.0374805262129629,0.235));
#50820=CARTESIAN_POINT('',(-0.221856282657939,0.0374805262129629,0.1175));
#50821=CARTESIAN_POINT('Ctrl Pts',(-0.215672897909674,0.0380289509090578,
0.241));
#50822=CARTESIAN_POINT('Ctrl Pts',(-0.218722810657132,0.037758444133281,
0.238043395288953));
#50823=CARTESIAN_POINT('Ctrl Pts',(-0.221856282657939,0.0374805262129629,
0.235));
#50824=CARTESIAN_POINT('Origin',(-0.218008688022331,0.0793486732515552,
0.04));
#50825=CARTESIAN_POINT('',(-0.211977362141128,0.0754360519890136,0.04));
#50826=CARTESIAN_POINT('',(-0.210873439877438,0.0784690534813353,0.04));
#50827=CARTESIAN_POINT('Origin',(0.,0.,0.04));
#50828=CARTESIAN_POINT('',(-0.205792683952114,0.0749024113883215,0.04));
#50829=CARTESIAN_POINT('',(-0.232618833095827,0.0772170867692875,0.04));
#50830=CARTESIAN_POINT('',(-0.205792683952114,0.0749024113883215,0.04));
#50831=CARTESIAN_POINT('Origin',(-0.205792683952114,0.0749024113883215,
0.04));
#50832=CARTESIAN_POINT('',(-0.210873439877438,0.0784690534813353,0.235));
#50833=CARTESIAN_POINT('',(-0.210873439877438,0.0784690534813353,0.1175));
#50834=CARTESIAN_POINT('',(-0.205792683952114,0.0749024113883215,0.241));
#50835=CARTESIAN_POINT('',(-0.205792683952114,0.0749024113883215,0.04));
#50836=CARTESIAN_POINT('Ctrl Pts',(-0.210873439877438,0.0784690534813352,
0.235));
#50837=CARTESIAN_POINT('Ctrl Pts',(-0.208298732482843,0.0766616335017642,
0.238043395288961));
#50838=CARTESIAN_POINT('Ctrl Pts',(-0.205792683952114,0.0749024113883215,
0.241));
#50839=CARTESIAN_POINT('Origin',(-0.232618833095827,0.0772170867692875,
0.04));
#50840=CARTESIAN_POINT('',(-0.211977362141128,0.0754360519890136,0.235));
#50841=CARTESIAN_POINT('',(-0.211977362141128,0.0754360519890136,0.1175));
#50842=CARTESIAN_POINT('Ctrl Pts',(-0.205792683952114,0.0749024113883215,
0.241));
#50843=CARTESIAN_POINT('Ctrl Pts',(-0.208843234680461,0.0751656260089316,
0.238043395288973));
#50844=CARTESIAN_POINT('Ctrl Pts',(-0.211977362141128,0.0754360519890136,
0.235));
#50845=CARTESIAN_POINT('Origin',(-0.20091789367799,0.116,0.04));
#50846=CARTESIAN_POINT('',(-0.195657616741379,0.111099491497862,0.04));
#50847=CARTESIAN_POINT('',(-0.194043790355372,0.113894720793023,0.04));
#50848=CARTESIAN_POINT('Origin',(0.,0.,0.04));
#50849=CARTESIAN_POINT('',(-0.189659563428792,0.1095,0.04));
#50850=CARTESIAN_POINT('',(-0.215676223927188,0.116437822173509,0.04));
#50851=CARTESIAN_POINT('',(-0.189659563428792,0.1095,0.04));
#50852=CARTESIAN_POINT('Origin',(-0.189659563428792,0.1095,0.04));
#50853=CARTESIAN_POINT('',(-0.194043790355372,0.113894720793023,0.235));
#50854=CARTESIAN_POINT('',(-0.194043790355372,0.113894720793023,0.1175));
#50855=CARTESIAN_POINT('',(-0.189659563428792,0.1095,0.241));
#50856=CARTESIAN_POINT('',(-0.189659563428792,0.1095,0.04));
#50857=CARTESIAN_POINT('Ctrl Pts',(-0.194043790355372,0.113894720793023,
0.235));
#50858=CARTESIAN_POINT('Ctrl Pts',(-0.19182205373716,0.111667666337086,
0.238043395288973));
#50859=CARTESIAN_POINT('Ctrl Pts',(-0.189659563428792,0.1095,0.241));
#50860=CARTESIAN_POINT('Origin',(-0.215676223927188,0.116437822173509,0.04));
#50861=CARTESIAN_POINT('',(-0.195657616741379,0.111099491497862,0.235));
#50862=CARTESIAN_POINT('',(-0.195657616741379,0.111099491497862,0.1175));
#50863=CARTESIAN_POINT('Ctrl Pts',(-0.189659563428792,0.1095,0.241));
#50864=CARTESIAN_POINT('Ctrl Pts',(-0.192618062697796,0.110288938373934,
0.238043395288998));
#50865=CARTESIAN_POINT('Ctrl Pts',(-0.195657616741379,0.111099491497862,
0.235));
#50866=CARTESIAN_POINT('Origin',(-0.177722310803603,0.149126725447277,0.04));
#50867=CARTESIAN_POINT('',(-0.173392913664475,0.143387229176604,0.04));
#50868=CARTESIAN_POINT('',(-0.171318218454253,0.145859754646924,0.04));
#50869=CARTESIAN_POINT('Origin',(0.,0.,0.04));
#50870=CARTESIAN_POINT('',(-0.167763733043056,0.140770486521352,0.04));
#50871=CARTESIAN_POINT('',(-0.192180401831955,0.152120653271369,0.04));
#50872=CARTESIAN_POINT('',(-0.167763733043056,0.140770486521352,0.04));
#50873=CARTESIAN_POINT('Origin',(-0.167763733043056,0.140770486521352,0.04));
#50874=CARTESIAN_POINT('',(-0.171318218454253,0.145859754646924,0.235));
#50875=CARTESIAN_POINT('',(-0.171318218454253,0.145859754646924,0.1175));
#50876=CARTESIAN_POINT('',(-0.167763733043056,0.140770486521352,0.241));
#50877=CARTESIAN_POINT('',(-0.167763733043056,0.140770486521352,0.04));
#50878=CARTESIAN_POINT('Ctrl Pts',(-0.171318218454253,0.145859754646924,
0.235));
#50879=CARTESIAN_POINT('Ctrl Pts',(-0.169516958955308,0.143280733637303,
0.238043395289003));
#50880=CARTESIAN_POINT('Ctrl Pts',(-0.167763733043056,0.140770486521352,
0.241));
#50881=CARTESIAN_POINT('Origin',(-0.192180401831955,0.152120653271369,0.04));
#50882=CARTESIAN_POINT('',(-0.173392913664475,0.143387229176604,0.235));
#50883=CARTESIAN_POINT('',(-0.173392913664475,0.143387229176604,0.1175));
#50884=CARTESIAN_POINT('Ctrl Pts',(-0.167763733043056,0.140770486521352,
0.241));
#50885=CARTESIAN_POINT('Ctrl Pts',(-0.170540288349497,0.142061177155329,
0.238043395289029));
#50886=CARTESIAN_POINT('Ctrl Pts',(-0.173392913664475,0.143387229176604,
0.235));
#50887=CARTESIAN_POINT('Origin',(-0.149126725447277,0.177722310803603,0.04));
#50888=CARTESIAN_POINT('',(-0.145859754646924,0.171318218454253,0.04));
#50889=CARTESIAN_POINT('',(-0.143387229176604,0.173392913664475,0.04));
#50890=CARTESIAN_POINT('Origin',(0.,0.,0.04));
#50891=CARTESIAN_POINT('',(-0.140770486521352,0.167763733043056,0.04));
#50892=CARTESIAN_POINT('',(-0.162845275475035,0.183181375296344,0.04));
#50893=CARTESIAN_POINT('',(-0.140770486521352,0.167763733043056,0.04));
#50894=CARTESIAN_POINT('Origin',(-0.140770486521352,0.167763733043056,0.04));
#50895=CARTESIAN_POINT('',(-0.143387229176604,0.173392913664475,0.235));
#50896=CARTESIAN_POINT('',(-0.143387229176604,0.173392913664475,0.1175));
#50897=CARTESIAN_POINT('',(-0.140770486521352,0.167763733043056,0.241));
#50898=CARTESIAN_POINT('',(-0.140770486521352,0.167763733043056,0.04));
#50899=CARTESIAN_POINT('Ctrl Pts',(-0.143387229176604,0.173392913664475,
0.235));
#50900=CARTESIAN_POINT('Ctrl Pts',(-0.14206117715533,0.170540288349499,
0.238043395289028));
#50901=CARTESIAN_POINT('Ctrl Pts',(-0.140770486521352,0.167763733043056,
0.241));
#50902=CARTESIAN_POINT('Origin',(-0.162845275475035,0.183181375296344,0.04));
#50903=CARTESIAN_POINT('',(-0.145859754646924,0.171318218454253,0.235));
#50904=CARTESIAN_POINT('',(-0.145859754646924,0.171318218454253,0.1175));
#50905=CARTESIAN_POINT('Ctrl Pts',(-0.140770486521352,0.167763733043056,
0.241));
#50906=CARTESIAN_POINT('Ctrl Pts',(-0.143280733637291,0.169516958955299,
0.238043395289017));
#50907=CARTESIAN_POINT('Ctrl Pts',(-0.145859754646924,0.171318218454253,
0.235));
#50908=CARTESIAN_POINT('Origin',(-0.116,0.20091789367799,0.04));
#50909=CARTESIAN_POINT('',(-0.113894720793023,0.194043790355372,0.04));
#50910=CARTESIAN_POINT('',(-0.111099491497862,0.195657616741379,0.04));
#50911=CARTESIAN_POINT('Origin',(0.,0.,0.04));
#50912=CARTESIAN_POINT('',(-0.1095,0.189659563428792,0.04));
#50913=CARTESIAN_POINT('',(-0.128562177826491,0.208676223927188,0.04));
#50914=CARTESIAN_POINT('',(-0.1095,0.189659563428792,0.04));
#50915=CARTESIAN_POINT('Origin',(-0.1095,0.189659563428792,0.04));
#50916=CARTESIAN_POINT('',(-0.111099491497862,0.195657616741379,0.235));
#50917=CARTESIAN_POINT('',(-0.111099491497862,0.195657616741379,0.1175));
#50918=CARTESIAN_POINT('',(-0.1095,0.189659563428792,0.241));
#50919=CARTESIAN_POINT('',(-0.1095,0.189659563428792,0.04));
#50920=CARTESIAN_POINT('Ctrl Pts',(-0.111099491497862,0.195657616741379,
0.235));
#50921=CARTESIAN_POINT('Ctrl Pts',(-0.110288938373934,0.192618062697795,
0.238043395288999));
#50922=CARTESIAN_POINT('Ctrl Pts',(-0.1095,0.189659563428792,0.241));
#50923=CARTESIAN_POINT('Origin',(-0.128562177826491,0.208676223927188,0.04));
#50924=CARTESIAN_POINT('',(-0.113894720793023,0.194043790355372,0.235));
#50925=CARTESIAN_POINT('',(-0.113894720793023,0.194043790355372,0.1175));
#50926=CARTESIAN_POINT('Ctrl Pts',(-0.1095,0.189659563428792,0.241));
#50927=CARTESIAN_POINT('Ctrl Pts',(-0.111667666337081,0.191822053737154,
0.23804339528898));
#50928=CARTESIAN_POINT('Ctrl Pts',(-0.113894720793023,0.194043790355372,
0.235));
#50929=CARTESIAN_POINT('Origin',(-0.0793486732515551,0.218008688022331,
0.04));
#50930=CARTESIAN_POINT('',(-0.0784690534813352,0.210873439877438,0.04));
#50931=CARTESIAN_POINT('',(-0.0754360519890136,0.211977362141128,0.04));
#50932=CARTESIAN_POINT('Origin',(0.,0.,0.04));
#50933=CARTESIAN_POINT('',(-0.0749024113883215,0.205792683952114,0.04));
#50934=CARTESIAN_POINT('',(-0.0903727834602902,0.227830551089268,0.04));
#50935=CARTESIAN_POINT('',(-0.0749024113883215,0.205792683952114,0.04));
#50936=CARTESIAN_POINT('Origin',(-0.0749024113883215,0.205792683952114,
0.04));
#50937=CARTESIAN_POINT('',(-0.0754360519890136,0.211977362141128,0.235));
#50938=CARTESIAN_POINT('',(-0.0754360519890136,0.211977362141128,0.1175));
#50939=CARTESIAN_POINT('',(-0.0749024113883215,0.205792683952114,0.241));
#50940=CARTESIAN_POINT('',(-0.0749024113883215,0.205792683952114,0.04));
#50941=CARTESIAN_POINT('Ctrl Pts',(-0.0754360519890136,0.211977362141128,
0.235));
#50942=CARTESIAN_POINT('Ctrl Pts',(-0.0751656260089268,0.208843234680406,
0.238043395289026));
#50943=CARTESIAN_POINT('Ctrl Pts',(-0.0749024113883215,0.205792683952114,
0.241));
#50944=CARTESIAN_POINT('Origin',(-0.0903727834602902,0.227830551089268,
0.04));
#50945=CARTESIAN_POINT('',(-0.0784690534813352,0.210873439877438,0.235));
#50946=CARTESIAN_POINT('',(-0.0784690534813352,0.210873439877438,0.1175));
#50947=CARTESIAN_POINT('Ctrl Pts',(-0.0749024113883215,0.205792683952114,
0.241));
#50948=CARTESIAN_POINT('Ctrl Pts',(-0.0766616335017707,0.208298732482853,
0.23804339528895));
#50949=CARTESIAN_POINT('Ctrl Pts',(-0.0784690534813352,0.210873439877438,
0.235));
#50950=CARTESIAN_POINT('Origin',(-0.0402863772187278,0.228475398698832,
0.04));
#50951=CARTESIAN_POINT('',(-0.0406591436868745,0.221295806635937,0.04));
#50952=CARTESIAN_POINT('',(-0.0374805262129628,0.221856282657939,0.04));
#50953=CARTESIAN_POINT('Origin',(0.,0.,0.04));
#50954=CARTESIAN_POINT('',(-0.0380289509090578,0.215672897909674,0.04));
#50955=CARTESIAN_POINT('',(-0.0494374577994834,0.240062362244323,0.04));
#50956=CARTESIAN_POINT('',(-0.0380289509090578,0.215672897909674,0.04));
#50957=CARTESIAN_POINT('Origin',(-0.0380289509090578,0.215672897909674,
0.04));
#50958=CARTESIAN_POINT('',(-0.0374805262129628,0.221856282657939,0.235));
#50959=CARTESIAN_POINT('',(-0.0374805262129628,0.221856282657939,0.1175));
#50960=CARTESIAN_POINT('',(-0.0380289509090578,0.215672897909674,0.241));
#50961=CARTESIAN_POINT('',(-0.0380289509090578,0.215672897909674,0.04));
#50962=CARTESIAN_POINT('Ctrl Pts',(-0.0374805262129628,0.221856282657939,
0.235));
#50963=CARTESIAN_POINT('Ctrl Pts',(-0.037758444133279,0.218722810657154,
0.238043395288931));
#50964=CARTESIAN_POINT('Ctrl Pts',(-0.0380289509090578,0.215672897909674,
0.241));
#50965=CARTESIAN_POINT('Origin',(-0.0494374577994834,0.240062362244323,
0.04));
#50966=CARTESIAN_POINT('',(-0.0406591436868745,0.221295806635937,0.235));
#50967=CARTESIAN_POINT('',(-0.0406591436868745,0.221295806635937,0.1175));
#50968=CARTESIAN_POINT('Ctrl Pts',(-0.0380289509090578,0.215672897909674,
0.241));
#50969=CARTESIAN_POINT('Ctrl Pts',(-0.0393262757251606,0.218446359646314,
0.238043395288915));
#50970=CARTESIAN_POINT('Ctrl Pts',(-0.0406591436868745,0.221295806635937,
0.235));
#50971=CARTESIAN_POINT('Origin',(1.38777878078145E-17,0.232,0.04));
#50972=CARTESIAN_POINT('',(-0.00161382638600747,0.224994212290885,0.04));
#50973=CARTESIAN_POINT('',(0.0016138263860075,0.224994212290885,0.04));
#50974=CARTESIAN_POINT('Origin',(0.,0.,0.04));
#50975=CARTESIAN_POINT('',(1.38777878078145E-17,0.219,0.04));
#50976=CARTESIAN_POINT('',(-0.00699999999999999,0.245,0.04));
#50977=CARTESIAN_POINT('',(1.38777878078145E-17,0.219,0.04));
#50978=CARTESIAN_POINT('Origin',(1.38777878078145E-17,0.219,0.04));
#50979=CARTESIAN_POINT('',(0.00161382638600752,0.224994212290885,0.235));
#50980=CARTESIAN_POINT('',(0.00161382638600752,0.224994212290885,0.1175));
#50981=CARTESIAN_POINT('',(1.38777878078145E-17,0.219,0.241));
#50982=CARTESIAN_POINT('',(1.38777878078145E-17,0.219,0.04));
#50983=CARTESIAN_POINT('Ctrl Pts',(0.00161382638600749,0.224994212290885,
0.235));
#50984=CARTESIAN_POINT('Ctrl Pts',(0.000796008960674862,0.221956604711078,
0.238043395288922));
#50985=CARTESIAN_POINT('Ctrl Pts',(1.38777878078145E-17,0.219,0.241));
#50986=CARTESIAN_POINT('Origin',(-0.00699999999999999,0.245,0.04));
#50987=CARTESIAN_POINT('',(-0.00161382638600748,0.224994212290885,0.235));
#50988=CARTESIAN_POINT('',(-0.00161382638600748,0.224994212290885,0.1175));
#50989=CARTESIAN_POINT('Ctrl Pts',(1.38777878078145E-17,0.219,0.241));
#50990=CARTESIAN_POINT('Ctrl Pts',(-0.000796008960647555,0.221956604710977,
0.238043395289023));
#50991=CARTESIAN_POINT('Ctrl Pts',(-0.00161382638600747,0.224994212290885,
0.235));
#50992=CARTESIAN_POINT('Origin',(0.0402863772187279,0.228475398698832,0.04));
#50993=CARTESIAN_POINT('',(0.0374805262129628,0.221856282657939,0.04));
#50994=CARTESIAN_POINT('',(0.0406591436868745,0.221295806635937,0.04));
#50995=CARTESIAN_POINT('Origin',(0.,0.,0.04));
#50996=CARTESIAN_POINT('',(0.0380289509090578,0.215672897909674,0.04));
#50997=CARTESIAN_POINT('',(0.0356501492573125,0.24249343673166,0.04));
#50998=CARTESIAN_POINT('',(0.0380289509090578,0.215672897909674,0.04));
#50999=CARTESIAN_POINT('Origin',(0.0380289509090578,0.215672897909674,0.04));
#51000=CARTESIAN_POINT('',(0.0406591436868745,0.221295806635937,0.235));
#51001=CARTESIAN_POINT('',(0.0406591436868745,0.221295806635937,0.1175));
#51002=CARTESIAN_POINT('',(0.0380289509090578,0.215672897909674,0.241));
#51003=CARTESIAN_POINT('',(0.0380289509090578,0.215672897909674,0.04));
#51004=CARTESIAN_POINT('Ctrl Pts',(0.0406591436868745,0.221295806635937,
0.235));
#51005=CARTESIAN_POINT('Ctrl Pts',(0.0393262757251286,0.218446359646246,
0.238043395288988));
#51006=CARTESIAN_POINT('Ctrl Pts',(0.0380289509090578,0.215672897909674,
0.241));
#51007=CARTESIAN_POINT('Origin',(0.0356501492573125,0.24249343673166,0.04));
#51008=CARTESIAN_POINT('',(0.0374805262129628,0.221856282657939,0.235));
#51009=CARTESIAN_POINT('',(0.0374805262129628,0.221856282657939,0.1175));
#51010=CARTESIAN_POINT('Ctrl Pts',(0.0380289509090578,0.215672897909674,
0.241));
#51011=CARTESIAN_POINT('Ctrl Pts',(0.0377584441332792,0.218722810657151,
0.238043395288934));
#51012=CARTESIAN_POINT('Ctrl Pts',(0.0374805262129628,0.221856282657939,
0.235));
#51013=CARTESIAN_POINT('Origin',(0.0793486732515552,0.218008688022331,0.04));
#51014=CARTESIAN_POINT('',(0.0754360519890136,0.211977362141128,0.04));
#51015=CARTESIAN_POINT('',(0.0784690534813353,0.210873439877438,0.04));
#51016=CARTESIAN_POINT('Origin',(0.,0.,0.04));
#51017=CARTESIAN_POINT('',(0.0749024113883215,0.205792683952114,0.04));
#51018=CARTESIAN_POINT('',(0.0772170867692875,0.232618833095827,0.04));
#51019=CARTESIAN_POINT('',(0.0749024113883215,0.205792683952114,0.04));
#51020=CARTESIAN_POINT('Origin',(0.0749024113883215,0.205792683952114,0.04));
#51021=CARTESIAN_POINT('',(0.0784690534813353,0.210873439877438,0.235));
#51022=CARTESIAN_POINT('',(0.0784690534813353,0.210873439877438,0.1175));
#51023=CARTESIAN_POINT('',(0.0749024113883215,0.205792683952114,0.241));
#51024=CARTESIAN_POINT('',(0.0749024113883215,0.205792683952114,0.04));
#51025=CARTESIAN_POINT('Ctrl Pts',(0.0784690534813352,0.210873439877438,
0.235));
#51026=CARTESIAN_POINT('Ctrl Pts',(0.0766616335017642,0.208298732482843,
0.238043395288961));
#51027=CARTESIAN_POINT('Ctrl Pts',(0.0749024113883215,0.205792683952114,
0.241));
#51028=CARTESIAN_POINT('Origin',(0.0772170867692875,0.232618833095827,0.04));
#51029=CARTESIAN_POINT('',(0.0754360519890136,0.211977362141128,0.235));
#51030=CARTESIAN_POINT('',(0.0754360519890136,0.211977362141128,0.1175));
#51031=CARTESIAN_POINT('Ctrl Pts',(0.0749024113883215,0.205792683952114,
0.241));
#51032=CARTESIAN_POINT('Ctrl Pts',(0.0751656260089316,0.208843234680461,
0.238043395288973));
#51033=CARTESIAN_POINT('Ctrl Pts',(0.0754360519890136,0.211977362141128,
0.235));
#51034=CARTESIAN_POINT('Origin',(0.116,0.20091789367799,0.04));
#51035=CARTESIAN_POINT('',(0.111099491497862,0.195657616741379,0.04));
#51036=CARTESIAN_POINT('',(0.113894720793023,0.194043790355372,0.04));
#51037=CARTESIAN_POINT('Origin',(0.,0.,0.04));
#51038=CARTESIAN_POINT('',(0.1095,0.189659563428792,0.04));
#51039=CARTESIAN_POINT('',(0.116437822173509,0.215676223927188,0.04));
#51040=CARTESIAN_POINT('',(0.1095,0.189659563428792,0.04));
#51041=CARTESIAN_POINT('Origin',(0.1095,0.189659563428792,0.04));
#51042=CARTESIAN_POINT('',(0.113894720793023,0.194043790355372,0.235));
#51043=CARTESIAN_POINT('',(0.113894720793023,0.194043790355372,0.1175));
#51044=CARTESIAN_POINT('',(0.1095,0.189659563428792,0.241));
#51045=CARTESIAN_POINT('',(0.1095,0.189659563428792,0.04));
#51046=CARTESIAN_POINT('Ctrl Pts',(0.113894720793023,0.194043790355372,
0.235));
#51047=CARTESIAN_POINT('Ctrl Pts',(0.111667666337037,0.19182205373711,0.23804339528904));
#51048=CARTESIAN_POINT('Ctrl Pts',(0.1095,0.189659563428792,0.241));
#51049=CARTESIAN_POINT('Origin',(0.116437822173509,0.215676223927188,0.04));
#51050=CARTESIAN_POINT('',(0.111099491497862,0.195657616741379,0.235));
#51051=CARTESIAN_POINT('',(0.111099491497862,0.195657616741379,0.1175));
#51052=CARTESIAN_POINT('Ctrl Pts',(0.1095,0.189659563428792,0.241));
#51053=CARTESIAN_POINT('Ctrl Pts',(0.110288938373932,0.192618062697786,
0.238043395289008));
#51054=CARTESIAN_POINT('Ctrl Pts',(0.111099491497862,0.195657616741379,
0.235));
#51055=CARTESIAN_POINT('Origin',(0.149126725447277,0.177722310803603,0.04));
#51056=CARTESIAN_POINT('',(0.143387229176604,0.173392913664475,0.04));
#51057=CARTESIAN_POINT('',(0.145859754646924,0.171318218454253,0.04));
#51058=CARTESIAN_POINT('Origin',(0.,0.,0.04));
#51059=CARTESIAN_POINT('',(0.140770486521352,0.167763733043056,0.04));
#51060=CARTESIAN_POINT('',(0.152120653271369,0.192180401831955,0.04));
#51061=CARTESIAN_POINT('',(0.140770486521352,0.167763733043056,0.04));
#51062=CARTESIAN_POINT('Origin',(0.140770486521352,0.167763733043056,0.04));
#51063=CARTESIAN_POINT('',(0.145859754646924,0.171318218454253,0.235));
#51064=CARTESIAN_POINT('',(0.145859754646924,0.171318218454253,0.1175));
#51065=CARTESIAN_POINT('',(0.140770486521352,0.167763733043056,0.241));
#51066=CARTESIAN_POINT('',(0.140770486521352,0.167763733043056,0.04));
#51067=CARTESIAN_POINT('Ctrl Pts',(0.145859754646924,0.171318218454253,
0.235));
#51068=CARTESIAN_POINT('Ctrl Pts',(0.143280733637348,0.169516958955339,
0.23804339528895));
#51069=CARTESIAN_POINT('Ctrl Pts',(0.140770486521352,0.167763733043056,
0.241));
#51070=CARTESIAN_POINT('Origin',(0.152120653271369,0.192180401831955,0.04));
#51071=CARTESIAN_POINT('',(0.143387229176604,0.173392913664475,0.235));
#51072=CARTESIAN_POINT('',(0.143387229176604,0.173392913664475,0.1175));
#51073=CARTESIAN_POINT('Ctrl Pts',(0.140770486521352,0.167763733043056,
0.241));
#51074=CARTESIAN_POINT('Ctrl Pts',(0.142061177155356,0.170540288349555,
0.238043395288967));
#51075=CARTESIAN_POINT('Ctrl Pts',(0.143387229176604,0.173392913664475,
0.235));
#51076=CARTESIAN_POINT('Origin',(0.177722310803603,0.149126725447277,0.04));
#51077=CARTESIAN_POINT('',(0.171318218454253,0.145859754646924,0.04));
#51078=CARTESIAN_POINT('',(0.173392913664475,0.143387229176604,0.04));
#51079=CARTESIAN_POINT('Origin',(0.,0.,0.04));
#51080=CARTESIAN_POINT('',(0.167763733043056,0.140770486521352,0.04));
#51081=CARTESIAN_POINT('',(0.183181375296344,0.162845275475035,0.04));
#51082=CARTESIAN_POINT('',(0.167763733043056,0.140770486521352,0.04));
#51083=CARTESIAN_POINT('Origin',(0.167763733043056,0.140770486521352,0.04));
#51084=CARTESIAN_POINT('',(0.173392913664475,0.143387229176604,0.235));
#51085=CARTESIAN_POINT('',(0.173392913664475,0.143387229176604,0.1175));
#51086=CARTESIAN_POINT('',(0.167763733043056,0.140770486521352,0.241));
#51087=CARTESIAN_POINT('',(0.167763733043056,0.140770486521352,0.04));
#51088=CARTESIAN_POINT('Ctrl Pts',(0.173392913664475,0.143387229176604,
0.235));
#51089=CARTESIAN_POINT('Ctrl Pts',(0.170540288349525,0.142061177155342,
0.238043395288999));
#51090=CARTESIAN_POINT('Ctrl Pts',(0.167763733043056,0.140770486521352,
0.241));
#51091=CARTESIAN_POINT('Origin',(0.183181375296344,0.162845275475035,0.04));
#51092=CARTESIAN_POINT('',(0.171318218454253,0.145859754646924,0.235));
#51093=CARTESIAN_POINT('',(0.171318218454253,0.145859754646924,0.1175));
#51094=CARTESIAN_POINT('Ctrl Pts',(0.167763733043056,0.140770486521352,
0.241));
#51095=CARTESIAN_POINT('Ctrl Pts',(0.169516958955354,0.14328073363737,0.238043395288925));
#51096=CARTESIAN_POINT('Ctrl Pts',(0.171318218454253,0.145859754646924,
0.235));
#51097=CARTESIAN_POINT('Origin',(0.20091789367799,0.116,0.04));
#51098=CARTESIAN_POINT('',(0.194043790355372,0.113894720793023,0.04));
#51099=CARTESIAN_POINT('',(0.195657616741379,0.111099491497862,0.04));
#51100=CARTESIAN_POINT('Origin',(0.,0.,0.04));
#51101=CARTESIAN_POINT('',(0.189659563428792,0.1095,0.04));
#51102=CARTESIAN_POINT('',(0.208676223927188,0.128562177826491,0.04));
#51103=CARTESIAN_POINT('',(0.189659563428792,0.1095,0.04));
#51104=CARTESIAN_POINT('Origin',(0.189659563428792,0.1095,0.04));
#51105=CARTESIAN_POINT('',(0.195657616741379,0.111099491497862,0.235));
#51106=CARTESIAN_POINT('',(0.195657616741379,0.111099491497862,0.1175));
#51107=CARTESIAN_POINT('',(0.189659563428792,0.1095,0.241));
#51108=CARTESIAN_POINT('',(0.189659563428792,0.1095,0.04));
#51109=CARTESIAN_POINT('Ctrl Pts',(0.195657616741379,0.111099491497862,
0.235));
#51110=CARTESIAN_POINT('Ctrl Pts',(0.192618062697788,0.110288938373932,
0.238043395289006));
#51111=CARTESIAN_POINT('Ctrl Pts',(0.189659563428792,0.1095,0.241));
#51112=CARTESIAN_POINT('Origin',(0.208676223927188,0.128562177826491,0.04));
#51113=CARTESIAN_POINT('',(0.194043790355372,0.113894720793023,0.235));
#51114=CARTESIAN_POINT('',(0.194043790355372,0.113894720793023,0.1175));
#51115=CARTESIAN_POINT('Ctrl Pts',(0.189659563428792,0.1095,0.241));
#51116=CARTESIAN_POINT('Ctrl Pts',(0.191822053737141,0.111667666337067,
0.238043395288999));
#51117=CARTESIAN_POINT('Ctrl Pts',(0.194043790355372,0.113894720793023,
0.235));
#51118=CARTESIAN_POINT('Origin',(0.218008688022331,0.0793486732515551,0.04));
#51119=CARTESIAN_POINT('',(0.210873439877438,0.0784690534813352,0.04));
#51120=CARTESIAN_POINT('',(0.211977362141128,0.0754360519890136,0.04));
#51121=CARTESIAN_POINT('Origin',(0.,0.,0.04));
#51122=CARTESIAN_POINT('',(0.205792683952114,0.0749024113883215,0.04));
#51123=CARTESIAN_POINT('',(0.227830551089268,0.0903727834602902,0.04));
#51124=CARTESIAN_POINT('',(0.205792683952114,0.0749024113883215,0.04));
#51125=CARTESIAN_POINT('Origin',(0.205792683952114,0.0749024113883215,0.04));
#51126=CARTESIAN_POINT('',(0.211977362141128,0.0754360519890136,0.235));
#51127=CARTESIAN_POINT('',(0.211977362141128,0.0754360519890136,0.1175));
#51128=CARTESIAN_POINT('',(0.205792683952114,0.0749024113883215,0.241));
#51129=CARTESIAN_POINT('',(0.205792683952114,0.0749024113883215,0.04));
#51130=CARTESIAN_POINT('Ctrl Pts',(0.211977362141128,0.0754360519890136,
0.235));
#51131=CARTESIAN_POINT('Ctrl Pts',(0.208843234680406,0.0751656260089268,
0.238043395289026));
#51132=CARTESIAN_POINT('Ctrl Pts',(0.205792683952114,0.0749024113883215,
0.241));
#51133=CARTESIAN_POINT('Origin',(0.227830551089268,0.0903727834602902,0.04));
#51134=CARTESIAN_POINT('',(0.210873439877438,0.0784690534813352,0.235));
#51135=CARTESIAN_POINT('',(0.210873439877438,0.0784690534813352,0.1175));
#51136=CARTESIAN_POINT('Ctrl Pts',(0.205792683952114,0.0749024113883215,
0.241));
#51137=CARTESIAN_POINT('Ctrl Pts',(0.208298732482853,0.0766616335017707,
0.23804339528895));
#51138=CARTESIAN_POINT('Ctrl Pts',(0.210873439877438,0.0784690534813352,
0.235));
#51139=CARTESIAN_POINT('Origin',(0.228475398698832,0.0402863772187278,0.04));
#51140=CARTESIAN_POINT('',(0.221295806635937,0.0406591436868745,0.04));
#51141=CARTESIAN_POINT('',(0.221856282657939,0.0374805262129628,0.04));
#51142=CARTESIAN_POINT('Origin',(0.,0.,0.04));
#51143=CARTESIAN_POINT('',(0.215672897909674,0.0380289509090578,0.04));
#51144=CARTESIAN_POINT('',(0.240062362244323,0.0494374577994834,0.04));
#51145=CARTESIAN_POINT('',(0.215672897909674,0.0380289509090578,0.04));
#51146=CARTESIAN_POINT('Origin',(0.215672897909674,0.0380289509090578,0.04));
#51147=CARTESIAN_POINT('',(0.221856282657939,0.0374805262129628,0.235));
#51148=CARTESIAN_POINT('',(0.221856282657939,0.0374805262129628,0.1175));
#51149=CARTESIAN_POINT('',(0.215672897909674,0.0380289509090578,0.241));
#51150=CARTESIAN_POINT('',(0.215672897909674,0.0380289509090578,0.04));
#51151=CARTESIAN_POINT('Ctrl Pts',(0.221856282657939,0.0374805262129628,
0.235));
#51152=CARTESIAN_POINT('Ctrl Pts',(0.218722810657102,0.0377584441332836,
0.238043395288982));
#51153=CARTESIAN_POINT('Ctrl Pts',(0.215672897909674,0.0380289509090578,
0.241));
#51154=CARTESIAN_POINT('Origin',(0.240062362244323,0.0494374577994834,0.04));
#51155=CARTESIAN_POINT('',(0.221295806635937,0.0406591436868745,0.235));
#51156=CARTESIAN_POINT('',(0.221295806635937,0.0406591436868745,0.1175));
#51157=CARTESIAN_POINT('Ctrl Pts',(0.215672897909674,0.0380289509090578,
0.241));
#51158=CARTESIAN_POINT('Ctrl Pts',(0.218446359646296,0.0393262757251521,
0.238043395288935));
#51159=CARTESIAN_POINT('Ctrl Pts',(0.221295806635937,0.0406591436868745,
0.235));
#51160=CARTESIAN_POINT('Origin',(0.,0.,0.1175));
#51161=CARTESIAN_POINT('Origin',(0.,0.,0.235));
#51162=CARTESIAN_POINT('Origin',(0.,0.,0.235));
#51163=CARTESIAN_POINT('Origin',(0.,0.,0.235));
#51164=CARTESIAN_POINT('Origin',(0.,0.,0.235));
#51165=CARTESIAN_POINT('Origin',(0.,0.,0.235));
#51166=CARTESIAN_POINT('Origin',(0.,0.,0.235));
#51167=CARTESIAN_POINT('Origin',(0.,0.,0.235));
#51168=CARTESIAN_POINT('Origin',(0.,0.,0.235));
#51169=CARTESIAN_POINT('Origin',(0.,0.,0.235));
#51170=CARTESIAN_POINT('Origin',(0.,0.,0.235));
#51171=CARTESIAN_POINT('Origin',(0.,0.,0.235));
#51172=CARTESIAN_POINT('Origin',(0.,0.,0.235));
#51173=CARTESIAN_POINT('Origin',(0.,0.,0.235));
#51174=CARTESIAN_POINT('Origin',(0.,0.,0.235));
#51175=CARTESIAN_POINT('Origin',(0.,0.,0.235));
#51176=CARTESIAN_POINT('Origin',(0.,0.,0.235));
#51177=CARTESIAN_POINT('Origin',(0.,0.,0.235));
#51178=CARTESIAN_POINT('',(-0.225,-2.75545529808154E-17,1.38777878078145E-17));
#51179=CARTESIAN_POINT('',(-0.225,-2.75545529808154E-17,0.1175));
#51180=CARTESIAN_POINT('Origin',(0.,0.,0.));
#51181=CARTESIAN_POINT('Origin',(0.,0.,0.235));
#51182=CARTESIAN_POINT('Origin',(0.,0.,0.235));
#51183=CARTESIAN_POINT('Origin',(0.,0.,0.235));
#51184=CARTESIAN_POINT('Origin',(0.,0.,0.235));
#51185=CARTESIAN_POINT('Origin',(0.,0.,0.235));
#51186=CARTESIAN_POINT('Origin',(0.,0.,0.235));
#51187=CARTESIAN_POINT('Origin',(0.,0.,0.235));
#51188=CARTESIAN_POINT('Origin',(0.,0.,0.235));
#51189=CARTESIAN_POINT('Origin',(0.,0.,0.235));
#51190=CARTESIAN_POINT('Origin',(0.,0.,0.235));
#51191=CARTESIAN_POINT('Origin',(0.,0.,0.235));
#51192=CARTESIAN_POINT('Origin',(0.,0.,0.235));
#51193=CARTESIAN_POINT('Origin',(0.,0.,0.235));
#51194=CARTESIAN_POINT('Origin',(0.,0.,0.235));
#51195=CARTESIAN_POINT('Origin',(0.,0.,0.235));
#51196=CARTESIAN_POINT('Origin',(0.,0.,0.235));
#51197=CARTESIAN_POINT('Origin',(0.,0.,0.235));
#51198=CARTESIAN_POINT('',(0.224994212290885,0.0016138263860075,0.235));
#51199=CARTESIAN_POINT('Origin',(0.,0.,0.235));
#51200=CARTESIAN_POINT('',(0.224994212290885,0.0016138263860075,0.04));
#51201=CARTESIAN_POINT('',(0.224994212290885,0.0016138263860075,0.1175));
#51202=CARTESIAN_POINT('',(0.224994212290885,-0.0016138263860075,0.04));
#51203=CARTESIAN_POINT('Origin',(0.,0.,0.04));
#51204=CARTESIAN_POINT('',(0.224994212290885,-0.0016138263860075,0.235));
#51205=CARTESIAN_POINT('',(0.224994212290885,-0.0016138263860075,0.1175));
#51206=CARTESIAN_POINT('Origin',(0.,0.,0.235));
#51207=CARTESIAN_POINT('Origin',(0.219,0.,0.04));
#51208=CARTESIAN_POINT('',(0.219,0.,0.04));
#51209=CARTESIAN_POINT('',(0.219,0.,0.04));
#51210=CARTESIAN_POINT('',(0.219,0.,0.241));
#51211=CARTESIAN_POINT('',(0.219,0.,0.04));
#51212=CARTESIAN_POINT('Ctrl Pts',(0.224994212290885,-0.0016138263860075,
0.235));
#51213=CARTESIAN_POINT('Ctrl Pts',(0.221956604710985,-0.000796008960649803,
0.238043395289015));
#51214=CARTESIAN_POINT('Ctrl Pts',(0.219,0.,0.241));
#51215=CARTESIAN_POINT('Origin',(0.245,0.007,0.04));
#51216=CARTESIAN_POINT('Ctrl Pts',(0.219,0.,0.241));
#51217=CARTESIAN_POINT('Ctrl Pts',(0.221956604710993,0.00079600896065191,
0.238043395289007));
#51218=CARTESIAN_POINT('Ctrl Pts',(0.224994212290885,0.00161382638600749,
0.235));
#51219=CARTESIAN_POINT('',(0.245,0.007,0.04));
#51220=CARTESIAN_POINT('Origin',(0.232,0.,0.04));
#51221=CARTESIAN_POINT('Origin',(0.,0.,0.2425));
#51222=CARTESIAN_POINT('',(-0.21,-2.57175827820944E-17,0.25));
#51223=CARTESIAN_POINT('Origin',(0.,0.,0.25));
#51224=CARTESIAN_POINT('',(-0.2175,-2.66360678814549E-17,0.2425));
#51225=CARTESIAN_POINT('Origin',(0.,0.,0.111632486540519));
#51226=CARTESIAN_POINT('',(0.,0.,0.0822649730810374));
#51227=CARTESIAN_POINT('',(-0.0908032840555568,1.11201951170706E-17,0.14));
#51228=CARTESIAN_POINT('',(-0.0461880215351701,-5.6564012731995E-18,0.111632486540519));
#51229=CARTESIAN_POINT('Origin',(0.,0.,0.14));
#51230=CARTESIAN_POINT('Origin',(1.38777878078145E-17,0.115470053837925,
0.25));
#51231=CARTESIAN_POINT('',(7.07050159149938E-18,0.115470053837925,0.25));
#51232=CARTESIAN_POINT('',(0.1,0.0577350269189626,0.25));
#51233=CARTESIAN_POINT('',(0.025,0.101036297108185,0.25));
#51234=CARTESIAN_POINT('',(1.38777878078145E-17,0.115470053837925,0.14));
#51235=CARTESIAN_POINT('',(7.07050159149938E-18,0.115470053837925,0.25));
#51236=CARTESIAN_POINT('',(0.1,0.0577350269189626,0.14));
#51237=CARTESIAN_POINT('',(0.1,0.0577350269189626,0.14));
#51238=CARTESIAN_POINT('',(0.1,0.0577350269189626,0.25));
#51239=CARTESIAN_POINT('Origin',(-0.1,0.0577350269189626,0.25));
#51240=CARTESIAN_POINT('',(-0.1,0.0577350269189626,0.25));
#51241=CARTESIAN_POINT('',(-0.075,0.0721687836487032,0.25));
#51242=CARTESIAN_POINT('',(-0.1,0.0577350269189626,0.14));
#51243=CARTESIAN_POINT('',(-0.1,0.0577350269189626,0.25));
#51244=CARTESIAN_POINT('',(7.07050159149938E-18,0.115470053837925,0.14));
#51245=CARTESIAN_POINT('Origin',(-0.1,-0.0577350269189626,0.25));
#51246=CARTESIAN_POINT('',(-0.1,-0.0577350269189626,0.25));
#51247=CARTESIAN_POINT('',(-0.1,-0.0288675134594813,0.25));
#51248=CARTESIAN_POINT('',(-0.1,-0.0577350269189626,0.14));
#51249=CARTESIAN_POINT('',(-0.1,-0.0577350269189626,0.25));
#51250=CARTESIAN_POINT('',(-0.1,0.0577350269189626,0.14));
#51251=CARTESIAN_POINT('Origin',(-2.77555756156289E-17,-0.115470053837925,
0.25));
#51252=CARTESIAN_POINT('',(-2.12115047744981E-17,-0.115470053837925,0.25));
#51253=CARTESIAN_POINT('',(-0.025,-0.101036297108185,0.25));
#51254=CARTESIAN_POINT('',(-2.77555756156289E-17,-0.115470053837925,0.14));
#51255=CARTESIAN_POINT('',(-2.12115047744981E-17,-0.115470053837925,0.25));
#51256=CARTESIAN_POINT('',(-0.1,-0.0577350269189626,0.14));
#51257=CARTESIAN_POINT('Origin',(0.1,-0.0577350269189626,0.25));
#51258=CARTESIAN_POINT('',(0.1,-0.0577350269189626,0.25));
#51259=CARTESIAN_POINT('',(0.075,-0.0721687836487033,0.25));
#51260=CARTESIAN_POINT('',(0.1,-0.0577350269189626,0.14));
#51261=CARTESIAN_POINT('',(0.1,-0.0577350269189626,0.25));
#51262=CARTESIAN_POINT('',(-2.12115047744981E-17,-0.115470053837925,0.14));
#51263=CARTESIAN_POINT('Origin',(0.1,0.0577350269189626,0.25));
#51264=CARTESIAN_POINT('',(0.1,0.0288675134594813,0.25));
#51265=CARTESIAN_POINT('',(0.1,-0.0577350269189626,0.14));
#51266=CARTESIAN_POINT('Origin',(0.,0.,0.14));
#51267=CARTESIAN_POINT('Origin',(0.095,0.,-0.6));
#51268=CARTESIAN_POINT('',(-0.095,-1.16341445918999E-17,-0.6));
#51269=CARTESIAN_POINT('Origin',(0.,0.,-0.6));
#51270=CARTESIAN_POINT('Origin',(0.,0.,-0.585));
#51271=CARTESIAN_POINT('',(-0.11,-1.34711147906209E-17,-0.585));
#51272=CARTESIAN_POINT('Origin',(0.,0.,-0.005));
#51273=CARTESIAN_POINT('',(-0.135,-1.65327317884893E-17,0.));
#51274=CARTESIAN_POINT('Origin',(0.,0.,0.));
#51275=CARTESIAN_POINT('',(-0.13,-1.59204083889156E-17,-0.005));
#51276=CARTESIAN_POINT('Origin',(0.225,0.,0.));
#51277=CARTESIAN_POINT('Origin',(0.,0.,0.25));
#54977=UNCERTAINTY_MEASURE_WITH_UNIT(LENGTH_MEASURE(0.001),#55003,
'DISTANCE_ACCURACY_VALUE',
'Maximum model space distance between geometric entities at asserted c
onnectivities');
#54980=UNCERTAINTY_MEASURE_WITH_UNIT(LENGTH_MEASURE(0.001),#55003,
'DISTANCE_ACCURACY_VALUE',
'Maximum model space distance between geometric entities at asserted c
onnectivities');
#54999=(
GEOMETRIC_REPRESENTATION_CONTEXT(3)
GLOBAL_UNCERTAINTY_ASSIGNED_CONTEXT((#54977))
GLOBAL_UNIT_ASSIGNED_CONTEXT((#55003,#55005,#55006))
REPRESENTATION_CONTEXT('','3D')
);
#55002=(
GEOMETRIC_REPRESENTATION_CONTEXT(3)
GLOBAL_UNCERTAINTY_ASSIGNED_CONTEXT((#54980))
GLOBAL_UNIT_ASSIGNED_CONTEXT((#55003,#55005,#55006))
REPRESENTATION_CONTEXT('','3D')
);
#55003=(
LENGTH_UNIT()
NAMED_UNIT(*)
SI_UNIT(.CENTI.,.METRE.)
);
#55005=(
NAMED_UNIT(*)
PLANE_ANGLE_UNIT()
SI_UNIT($,.RADIAN.)
);
#55006=(
NAMED_UNIT(*)
SI_UNIT($,.STERADIAN.)
SOLID_ANGLE_UNIT()
);
#55025=SHAPE_DEFINITION_REPRESENTATION(#55046,#55121);
#55046=PRODUCT_DEFINITION_SHAPE('',$,#55143);
#55121=SHAPE_REPRESENTATION('',(#26786),#54999);
#55124=PRODUCT_DEFINITION_CONTEXT('part definition',#55189,'design');
#55143=PRODUCT_DEFINITION('2026-10-18-23-36-59-357',
'17_ISO_4762_M2.5x6_A2',#55164,#55124);
#55164=PRODUCT_DEFINITION_FORMATION('',$,#55209);
#55189=APPLICATION_CONTEXT(
'Core Data for Automotive Mechanical Design Process');
#55190=PRODUCT_CONTEXT('part definition',#55189,'mechanical');
#55209=PRODUCT('2026-10-18-23-36-59-357','17_ISO_4762_M2.5x6_A2',$,(#55190));
#55387=COLOUR_RGB('Black',0.12,0.14,0.17);
#55388=FILL_AREA_STYLE_COLOUR('',#55387);
#55389=FILL_AREA_STYLE('',(#55388));
#55390=SURFACE_STYLE_FILL_AREA(#55389);
#55391=SURFACE_SIDE_STYLE('',(#55390));
#55392=SURFACE_STYLE_USAGE(.BOTH.,#55391);
#55393=PRESENTATION_STYLE_ASSIGNMENT((#55392));
ENDSEC;
END-ISO-10303-21;
